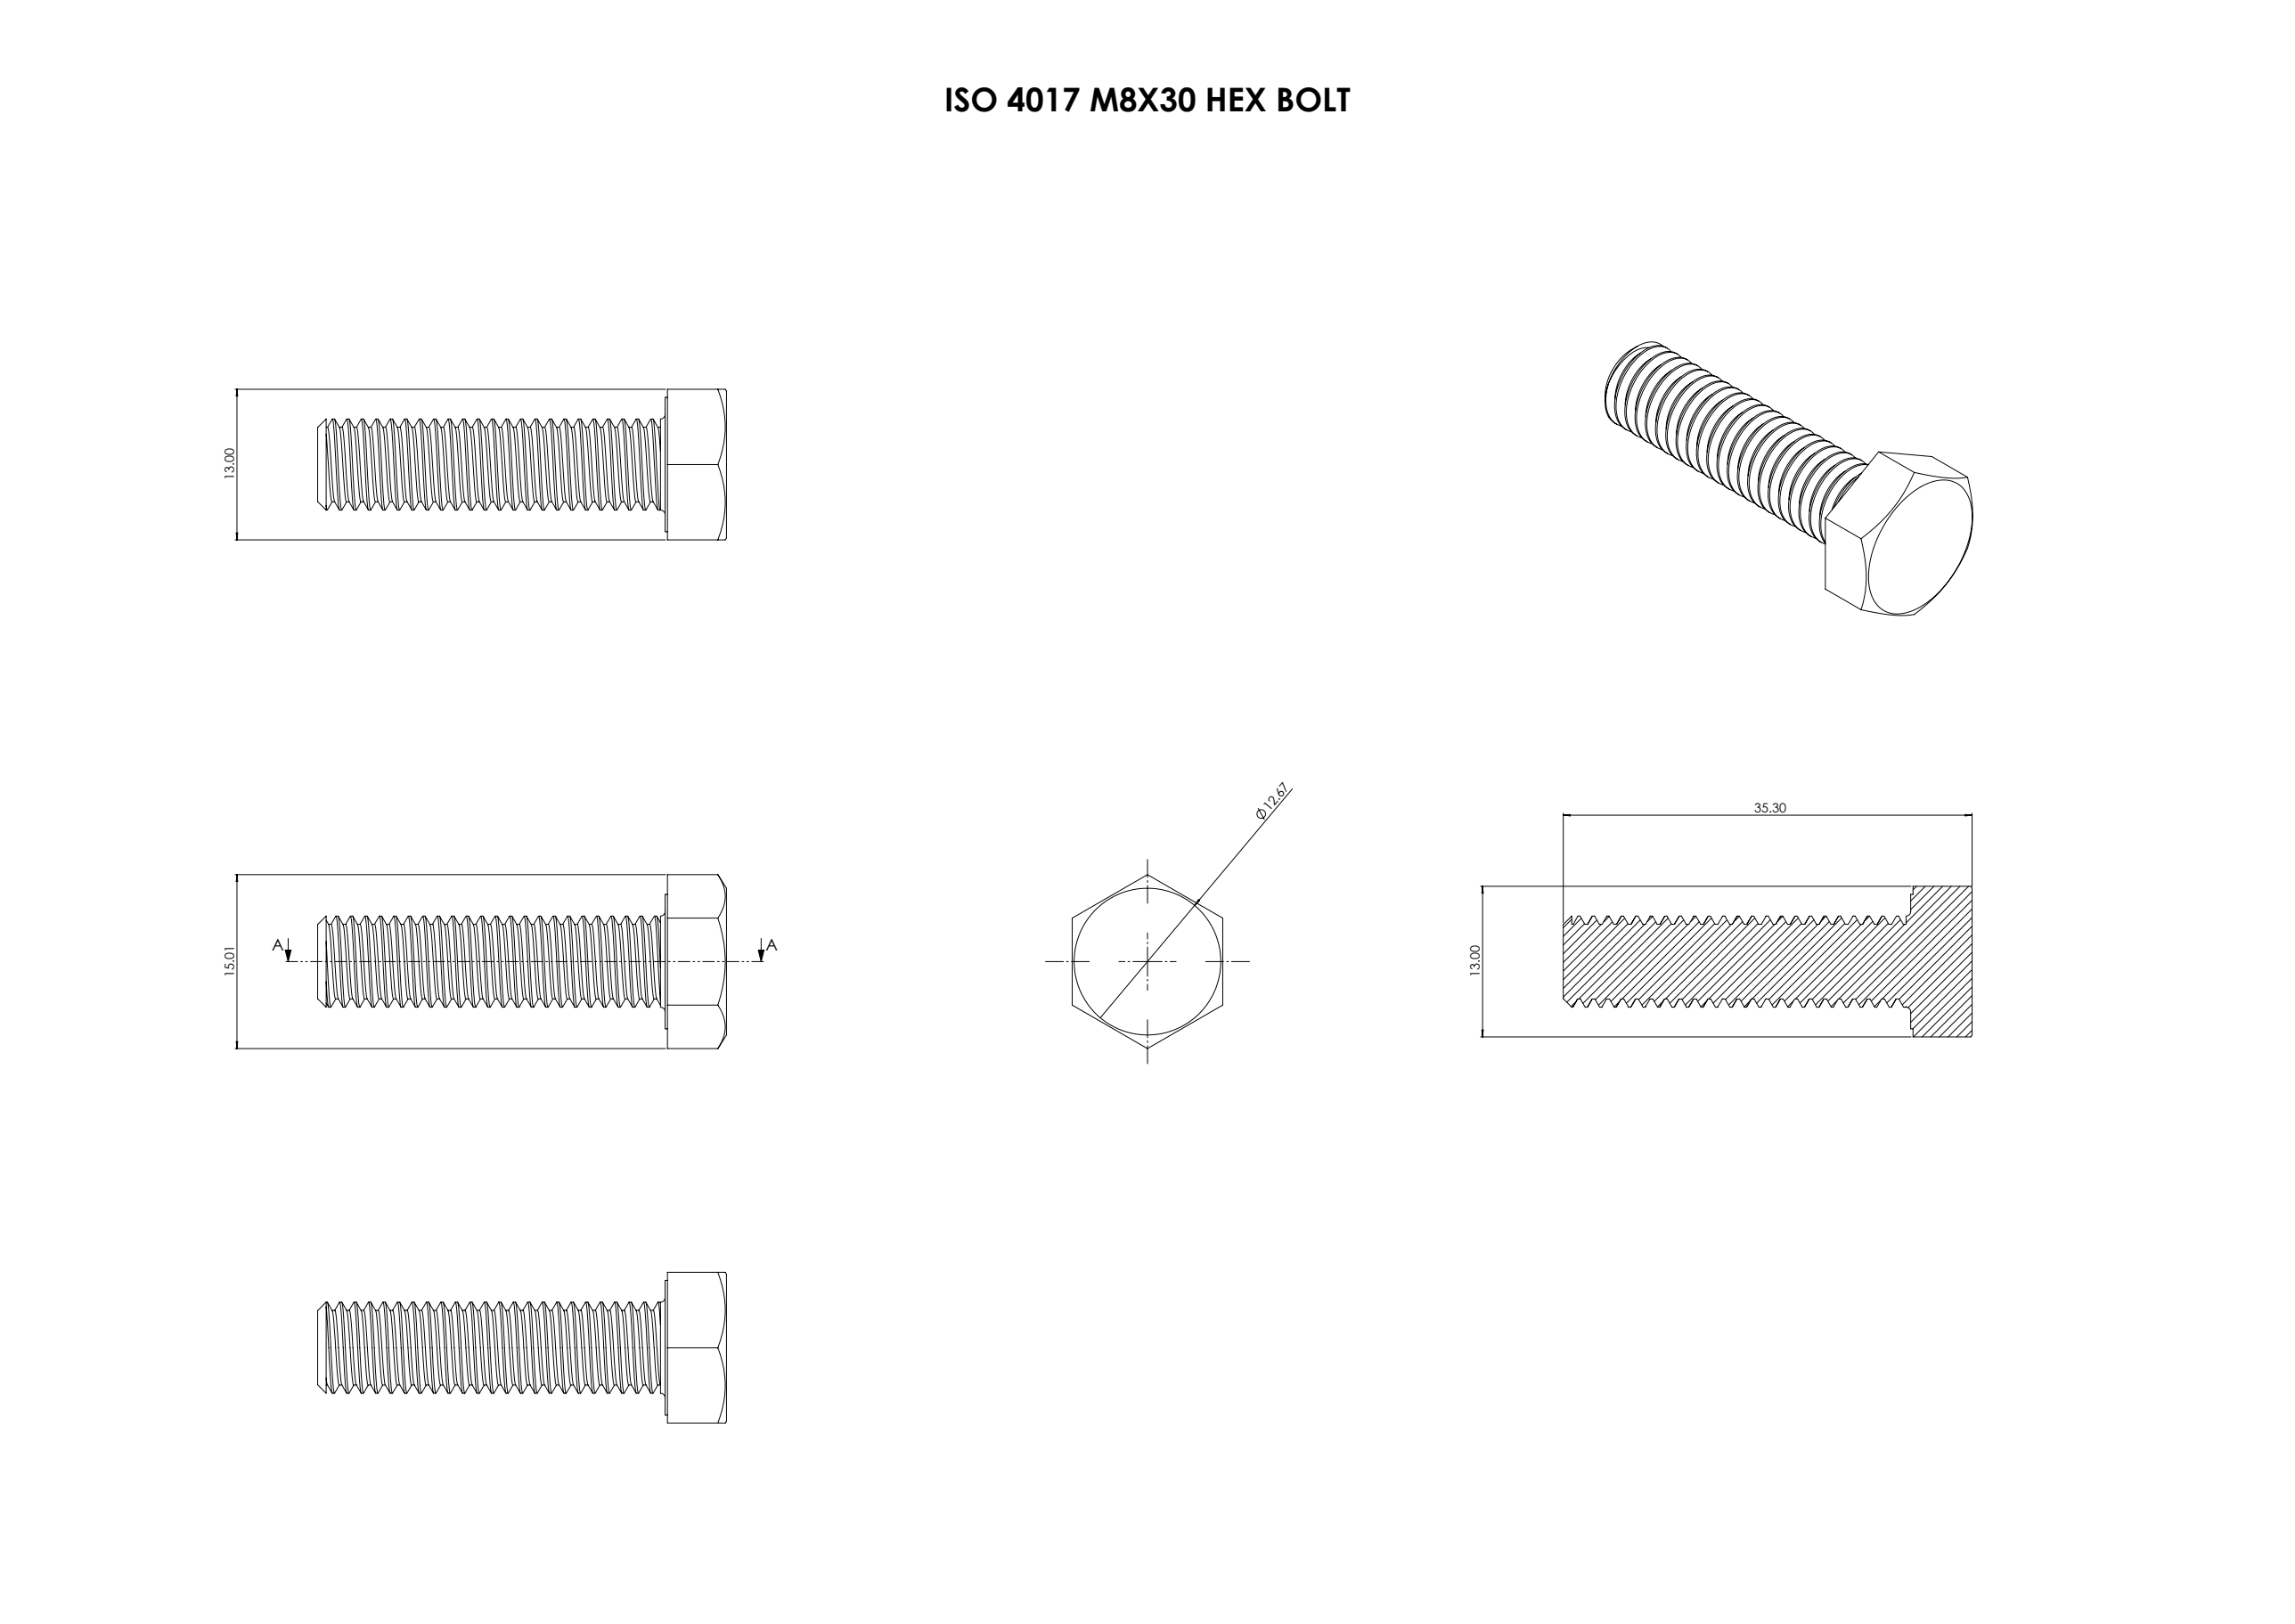
ISO-10303-21;
HEADER;
/* Generated by software containing ST-Developer
 * from STEP Tools, Inc. (www.steptools.com) 
 */

FILE_DESCRIPTION(
/* description */ (''),
/* implementation_level */ '2;1');

FILE_NAME(
/* name */ '11_ISO_4017_M8x30_Hex_Bolt.step',
/* time_stamp */ '2026-10-11T08:27:52-07:00',
/* author */ (''),
/* organization */ (''),
/* preprocessor_version */ 'ST-DEVELOPER v20.2',
/* originating_system */ 'Autodesk Translation Framework v15.15.0.0',
/* authorisation */ '');

FILE_SCHEMA (('AUTOMOTIVE_DESIGN { 1 0 10303 214 3 1 1 }'));
ENDSEC;

DATA;
#10=MECHANICAL_DESIGN_GEOMETRIC_PRESENTATION_REPRESENTATION('',(#929),#94301);
#619=B_SPLINE_CURVE_WITH_KNOTS('',3,(#90636,#90637,#90638,#90639,#90640,
#90641,#90642,#90643,#90644,#90645),.UNSPECIFIED.,.F.,.F.,(4,3,3,4),(-4.09274904019423,
-3.97736675155131,-2.98302506366348,-2.06120159751574),.UNSPECIFIED.);
#620=B_SPLINE_CURVE_WITH_KNOTS('',3,(#90648,#90649,#90650,#90651,#90652,
#90653,#90654),.UNSPECIFIED.,.F.,.F.,(4,3,4),(0.,0.994341687887822,1.11004521091126),
 .UNSPECIFIED.);
#621=B_SPLINE_CURVE_WITH_KNOTS('',3,(#90659,#90660,#90661,#90662,#90663,
#90664,#90665,#90666,#90667,#90668,#90669,#90670,#90671,#90672,#90673,#90674,
#90675,#90676,#90677,#90678,#90679,#90680),.UNSPECIFIED.,.F.,.F.,(4,3,3,
3,3,3,3,4),(-10.3759343473738,-9.94341687887826,-8.94907519099043,-7.95473350310261,
-6.96039181521478,-5.96605012732696,-4.97170843943913,-4.09274904019423),
 .UNSPECIFIED.);
#622=B_SPLINE_CURVE_WITH_KNOTS('',3,(#90681,#90682,#90683,#90684,#90685,
#90686,#90687,#90688,#90689,#90690,#90691,#90692,#90693,#90694,#90695,#90696,
#90697,#90698,#90699,#90700,#90701,#90702),.UNSPECIFIED.,.F.,.F.,(4,3,3,
3,3,3,3,4),(1.11004521091126,1.98868337577565,2.98302506366347,3.9773667515513,
4.97170843943912,5.96605012732695,6.96039181521477,7.39323051809085),
 .UNSPECIFIED.);
#623=B_SPLINE_CURVE_WITH_KNOTS('',3,(#90707,#90708,#90709,#90710,#90711,
#90712,#90713,#90714,#90715,#90716,#90717,#90718,#90719,#90720,#90721,#90722,
#90723,#90724,#90725,#90726,#90727,#90728),.UNSPECIFIED.,.F.,.F.,(4,3,3,
3,3,3,3,4),(-16.6591196545534,-15.9094670062052,-14.9151253183174,-13.9207836304296,
-12.9264419425417,-11.9321002546539,-10.9377585667661,-10.3759343473738),
 .UNSPECIFIED.);
#624=B_SPLINE_CURVE_WITH_KNOTS('',3,(#90729,#90730,#90731,#90732,#90733,
#90734,#90735,#90736,#90737,#90738,#90739,#90740,#90741,#90742,#90743,#90744,
#90745,#90746,#90747,#90748,#90749,#90750),.UNSPECIFIED.,.F.,.F.,(4,3,3,
3,3,3,3,4),(7.39323051809085,7.9547335031026,8.94907519099043,9.94341687887826,
10.9377585667661,11.9321002546539,12.9264419425418,13.6764158252704),
 .UNSPECIFIED.);
#625=B_SPLINE_CURVE_WITH_KNOTS('',3,(#90755,#90756,#90757,#90758,#90759,
#90760,#90761,#90762,#90763,#90764,#90765,#90766,#90767,#90768,#90769,#90770,
#90771,#90772,#90773,#90774,#90775,#90776,#90777,#90778,#90779),
 .UNSPECIFIED.,.F.,.F.,(4,3,3,3,3,3,3,3,4),(-22.942304961733,-22.86985882142,
-21.8755171335322,-20.8811754456444,-19.8868337577565,-18.8924920698687,
-17.8981503819809,-16.903808694093,-16.6591196545534),.UNSPECIFIED.);
#626=B_SPLINE_CURVE_WITH_KNOTS('',3,(#90780,#90781,#90782,#90783,#90784,
#90785,#90786,#90787,#90788,#90789,#90790,#90791,#90792,#90793,#90794,#90795,
#90796,#90797,#90798,#90799,#90800,#90801,#90802,#90803,#90804),
 .UNSPECIFIED.,.F.,.F.,(4,3,3,3,3,3,3,3,4),(13.6764158252704,13.9207836304296,
14.9151253183174,15.9094670062052,16.9038086940931,17.8981503819809,18.8924920698687,
19.8868337577565,19.95960113245),.UNSPECIFIED.);
#627=B_SPLINE_CURVE_WITH_KNOTS('',3,(#90809,#90810,#90811,#90812,#90813,
#90814,#90815,#90816,#90817,#90818,#90819,#90820,#90821,#90822,#90823,#90824,
#90825,#90826,#90827,#90828,#90829,#90830),.UNSPECIFIED.,.F.,.F.,(4,3,3,
3,3,3,3,4),(-29.2254902689126,-28.835908948747,-27.8415672608591,-26.8472255729713,
-25.8528838850835,-24.8585421971957,-23.8642005093078,-22.942304961733),
 .UNSPECIFIED.);
#628=B_SPLINE_CURVE_WITH_KNOTS('',3,(#90831,#90832,#90833,#90834,#90835,
#90836,#90837,#90838,#90839,#90840,#90841,#90842,#90843,#90844,#90845,#90846,
#90847,#90848,#90849,#90850,#90851,#90852),.UNSPECIFIED.,.F.,.F.,(4,3,3,
3,3,3,3,4),(19.95960113245,20.8811754456443,21.8755171335322,22.86985882142,
23.8642005093078,24.8585421971956,25.8528838850835,26.2427864396296),
 .UNSPECIFIED.);
#629=B_SPLINE_CURVE_WITH_KNOTS('',3,(#90857,#90858,#90859,#90860,#90861,
#90862,#90863,#90864,#90865,#90866,#90867,#90868,#90869,#90870,#90871,#90872,
#90873,#90874,#90875,#90876,#90877,#90878),.UNSPECIFIED.,.F.,.F.,(4,3,3,
3,3,3,3,4),(-35.5086755760922,-34.8019590760739,-33.8076173881861,-32.8132757002983,
-31.8189340124104,-30.8245923245226,-29.8302506366348,-29.2254902689126),
 .UNSPECIFIED.);
#630=B_SPLINE_CURVE_WITH_KNOTS('',3,(#90879,#90880,#90881,#90882,#90883,
#90884,#90885,#90886,#90887,#90888,#90889,#90890,#90891,#90892,#90893,#90894,
#90895,#90896,#90897,#90898,#90899,#90900),.UNSPECIFIED.,.F.,.F.,(4,3,3,
3,3,3,3,4),(26.2427864396296,26.8472255729713,27.8415672608591,28.8359089487469,
29.8302506366348,30.8245923245226,31.8189340124104,32.5259717468092),
 .UNSPECIFIED.);
#631=B_SPLINE_CURVE_WITH_KNOTS('',3,(#90905,#90906,#90907,#90908,#90909,
#90910,#90911,#90912,#90913,#90914,#90915,#90916,#90917,#90918,#90919,#90920,
#90921,#90922,#90923,#90924,#90925,#90926,#90927,#90928,#90929),
 .UNSPECIFIED.,.F.,.F.,(4,3,3,3,3,3,3,3,4),(-41.7918608832717,-41.7623508912887,
-40.7680092034009,-39.773667515513,-38.7793258276252,-37.7849841397374,
-36.7906424518496,-35.7963007639617,-35.5086755760922),.UNSPECIFIED.);
#632=B_SPLINE_CURVE_WITH_KNOTS('',3,(#90930,#90931,#90932,#90933,#90934,
#90935,#90936,#90937,#90938,#90939,#90940,#90941,#90942,#90943,#90944,#90945,
#90946,#90947,#90948,#90949,#90950,#90951,#90952,#90953,#90954),
 .UNSPECIFIED.,.F.,.F.,(4,3,3,3,3,3,3,3,4),(32.5259717468092,32.8132757002983,
33.8076173881861,34.8019590760739,35.7963007639617,36.7906424518496,37.7849841397374,
38.7793258276252,38.8091570539888),.UNSPECIFIED.);
#633=B_SPLINE_CURVE_WITH_KNOTS('',3,(#90959,#90960,#90961,#90962,#90963,
#90964,#90965,#90966,#90967,#90968,#90969,#90970,#90971,#90972,#90973,#90974,
#90975,#90976,#90977,#90978,#90979,#90980),.UNSPECIFIED.,.F.,.F.,(4,3,3,
3,3,3,3,4),(-48.0750461904514,-47.7284010186156,-46.7340593307278,-45.73971764284,
-44.7453759549522,-43.7510342670644,-42.7566925791765,-41.7918608832717),
 .UNSPECIFIED.);
#634=B_SPLINE_CURVE_WITH_KNOTS('',3,(#90981,#90982,#90983,#90984,#90985,
#90986,#90987,#90988,#90989,#90990,#90991,#90992,#90993,#90994,#90995,#90996,
#90997,#90998,#90999,#91000,#91001,#91002),.UNSPECIFIED.,.F.,.F.,(4,3,3,
3,3,3,3,4),(38.8091570539888,39.773667515513,40.7680092034009,41.7623508912887,
42.7566925791765,43.7510342670643,44.7453759549522,45.0923423611684),
 .UNSPECIFIED.);
#635=B_SPLINE_CURVE_WITH_KNOTS('',3,(#91007,#91008,#91009,#91010,#91011,
#91012,#91013,#91014,#91015,#91016,#91017,#91018,#91019,#91020,#91021,#91022,
#91023,#91024,#91025,#91026,#91027,#91028),.UNSPECIFIED.,.F.,.F.,(4,3,3,
3,3,3,3,4),(-54.3582314976309,-53.6944511459426,-52.7001094580548,-51.705767770167,
-50.7114260822791,-49.7170843943913,-48.7227427065035,-48.0750461904514),
 .UNSPECIFIED.);
#636=B_SPLINE_CURVE_WITH_KNOTS('',3,(#91029,#91030,#91031,#91032,#91033,
#91034,#91035,#91036,#91037,#91038,#91039,#91040,#91041,#91042,#91043,#91044,
#91045,#91046,#91047,#91048,#91049,#91050),.UNSPECIFIED.,.F.,.F.,(4,3,3,
3,3,3,3,4),(45.0923423611684,45.73971764284,46.7340593307278,47.7284010186156,
48.7227427065035,49.7170843943913,50.7114260822791,51.375527668348),
 .UNSPECIFIED.);
#637=B_SPLINE_CURVE_WITH_KNOTS('',3,(#91055,#91056,#91057,#91058,#91059,
#91060,#91061,#91062,#91063,#91064,#91065,#91066,#91067,#91068,#91069,#91070,
#91071,#91072,#91073,#91074,#91075,#91076),.UNSPECIFIED.,.F.,.F.,(4,3,3,
3,3,3,3,4),(-60.6414168048105,-59.6605012732696,-58.6661595853817,-57.6718178974939,
-56.6774762096061,-55.6831345217183,-54.6887928338304,-54.3582314976309),
 .UNSPECIFIED.);
#638=B_SPLINE_CURVE_WITH_KNOTS('',3,(#91077,#91078,#91079,#91080,#91081,
#91082,#91083,#91084,#91085,#91086,#91087,#91088,#91089,#91090,#91091,#91092,
#91093,#91094,#91095,#91096,#91097,#91098),.UNSPECIFIED.,.F.,.F.,(4,3,3,
3,3,3,3,4),(51.375527668348,51.705767770167,52.7001094580548,53.6944511459426,
54.6887928338304,55.6831345217183,56.6774762096061,57.6587129755276),
 .UNSPECIFIED.);
#639=B_SPLINE_CURVE_WITH_KNOTS('',3,(#91103,#91104,#91105,#91106,#91107,
#91108,#91109,#91110,#91111,#91112,#91113,#91114,#91115,#91116,#91117,#91118,
#91119,#91120,#91121,#91122,#91123,#91124,#91125,#91126,#91127),
 .UNSPECIFIED.,.F.,.F.,(4,3,3,3,3,3,3,3,4),(-66.9246021119901,-66.6208930884844,
-65.6265514005965,-64.6322097127087,-63.6378680248209,-62.643526336933,
-61.6491846490452,-60.6548429611574,-60.6414168048105),.UNSPECIFIED.);
#640=B_SPLINE_CURVE_WITH_KNOTS('',3,(#91128,#91129,#91130,#91131,#91132,
#91133,#91134,#91135,#91136,#91137,#91138,#91139,#91140,#91141,#91142,#91143,
#91144,#91145,#91146,#91147,#91148,#91149,#91150,#91151,#91152),
 .UNSPECIFIED.,.F.,.F.,(4,3,3,3,3,3,3,3,4),(57.6587129755276,57.6718178974939,
58.6661595853817,59.6605012732696,60.6548429611574,61.6491846490452,62.643526336933,
63.6378680248209,63.9418982827072),.UNSPECIFIED.);
#641=B_SPLINE_CURVE_WITH_KNOTS('',3,(#91157,#91158,#91159,#91160,#91161,
#91162,#91163,#91164,#91165,#91166,#91167,#91168,#91169,#91170,#91171,#91172,
#91173,#91174,#91175,#91176,#91177,#91178),.UNSPECIFIED.,.F.,.F.,(4,3,3,
3,3,3,3,4),(-73.2077874191697,-72.5869432158113,-71.5926015279235,-70.5982598400356,
-69.6039181521478,-68.60957646426,-67.6152347763722,-66.9246021119901),
 .UNSPECIFIED.);
#642=B_SPLINE_CURVE_WITH_KNOTS('',3,(#91179,#91180,#91181,#91182,#91183,
#91184,#91185,#91186,#91187,#91188,#91189,#91190,#91191,#91192,#91193,#91194,
#91195,#91196,#91197,#91198,#91199,#91200),.UNSPECIFIED.,.F.,.F.,(4,3,3,
3,3,3,3,4),(63.9418982827072,64.6322097127087,65.6265514005965,66.6208930884843,
67.6152347763722,68.60957646426,69.6039181521478,70.2250835898868),
 .UNSPECIFIED.);
#643=B_SPLINE_CURVE_WITH_KNOTS('',3,(#91205,#91206,#91207,#91208,#91209,
#91210,#91211,#91212,#91213,#91214,#91215,#91216,#91217,#91218,#91219,#91220,
#91221,#91222,#91223,#91224,#91225,#91226),.UNSPECIFIED.,.F.,.F.,(4,3,3,
3,3,3,3,4),(-79.4909727263493,-78.5529933431383,-77.5586516552504,-76.5643099673626,
-75.5699682794748,-74.575626591587,-73.5812849036991,-73.2077874191697),
 .UNSPECIFIED.);
#644=B_SPLINE_CURVE_WITH_KNOTS('',3,(#91227,#91228,#91229,#91230,#91231,
#91232,#91233,#91234,#91235,#91236,#91237,#91238,#91239,#91240,#91241,#91242,
#91243,#91244,#91245,#91246,#91247,#91248),.UNSPECIFIED.,.F.,.F.,(4,3,3,
3,3,3,3,4),(70.2250835898868,70.5982598400356,71.5926015279234,72.5869432158113,
73.5812849036991,74.5756265915869,75.5699682794748,76.5082688970663),
 .UNSPECIFIED.);
#645=B_SPLINE_CURVE_WITH_KNOTS('',3,(#91253,#91254,#91255,#91256,#91257,
#91258,#91259,#91260,#91261,#91262,#91263,#91264,#91265,#91266,#91267,#91268,
#91269,#91270,#91271,#91272,#91273,#91274,#91275,#91276,#91277),
 .UNSPECIFIED.,.F.,.F.,(4,3,3,3,3,3,3,3,4),(-85.7741580335289,-85.513385158353,
-84.5190434704652,-83.5247017825774,-82.5303600946896,-81.5360184068017,
-80.5416767189139,-79.5473350310261,-79.4909727263493),.UNSPECIFIED.);
#646=B_SPLINE_CURVE_WITH_KNOTS('',3,(#91278,#91279,#91280,#91281,#91282,
#91283,#91284,#91285,#91286,#91287,#91288,#91289,#91290,#91291,#91292,#91293,
#91294,#91295,#91296,#91297,#91298,#91299,#91300,#91301,#91302),
 .UNSPECIFIED.,.F.,.F.,(4,3,3,3,3,3,3,3,4),(76.5082688970663,76.5643099673626,
77.5586516552504,78.5529933431382,79.5473350310261,80.5416767189139,81.5360184068017,
82.5303600946895,82.7914542042459),.UNSPECIFIED.);
#647=B_SPLINE_CURVE_WITH_KNOTS('',3,(#91307,#91308,#91309,#91310,#91311,
#91312,#91313,#91314,#91315,#91316,#91317,#91318,#91319,#91320,#91321,#91322,
#91323,#91324,#91325,#91326,#91327,#91328),.UNSPECIFIED.,.F.,.F.,(4,3,3,
3,3,3,3,4),(-92.0573433407085,-91.47943528568,-90.4850935977922,-89.4907519099043,
-88.4964102220165,-87.5020685341287,-86.5077268462409,-85.7741580335289),
 .UNSPECIFIED.);
#648=B_SPLINE_CURVE_WITH_KNOTS('',3,(#91329,#91330,#91331,#91332,#91333,
#91334,#91335,#91336,#91337,#91338,#91339,#91340,#91341,#91342,#91343,#91344,
#91345,#91346,#91347,#91348,#91349,#91350),.UNSPECIFIED.,.F.,.F.,(4,3,3,
3,3,3,3,4),(82.7914542042459,83.5247017825774,84.5190434704652,85.513385158353,
86.5077268462408,87.5020685341287,88.4964102220165,89.0746395114255),
 .UNSPECIFIED.);
#649=B_SPLINE_CURVE_WITH_KNOTS('',3,(#91355,#91356,#91357,#91358,#91359,
#91360,#91361,#91362,#91363,#91364,#91365,#91366,#91367,#91368,#91369,#91370,
#91371,#91372,#91373,#91374,#91375,#91376),.UNSPECIFIED.,.F.,.F.,(4,3,3,
3,3,3,3,4),(-98.3405286478881,-97.4454854130069,-96.4511437251191,-95.4568020372313,
-94.4624603493435,-93.4681186614556,-92.4737769735678,-92.0573433407085),
 .UNSPECIFIED.);
#650=B_SPLINE_CURVE_WITH_KNOTS('',3,(#91377,#91378,#91379,#91380,#91381,
#91382,#91383,#91384,#91385,#91386,#91387,#91388,#91389,#91390,#91391,#91392,
#91393,#91394,#91395,#91396,#91397,#91398),.UNSPECIFIED.,.F.,.F.,(4,3,3,
3,3,3,3,4),(89.0746395114255,89.4907519099043,90.4850935977922,91.47943528568,
92.4737769735678,93.4681186614556,94.4624603493435,95.3578248186051),
 .UNSPECIFIED.);
#651=B_SPLINE_CURVE_WITH_KNOTS('',3,(#91403,#91404,#91405,#91406,#91407,
#91408,#91409,#91410,#91411,#91412,#91413,#91414,#91415,#91416,#91417,#91418,
#91419,#91420,#91421,#91422,#91423,#91424,#91425,#91426,#91427),
 .UNSPECIFIED.,.F.,.F.,(4,3,3,3,3,3,3,3,4),(-104.623713955068,-104.405877228222,
-103.411535540334,-102.417193852446,-101.422852164558,-100.42851047667,
-99.4341687887826,-98.4398271008948,-98.3405286478881),.UNSPECIFIED.);
#652=B_SPLINE_CURVE_WITH_KNOTS('',3,(#91428,#91429,#91430,#91431,#91432,
#91433,#91434,#91435,#91436,#91437,#91438,#91439,#91440,#91441,#91442,#91443,
#91444,#91445,#91446,#91447,#91448,#91449,#91450,#91451,#91452),
 .UNSPECIFIED.,.F.,.F.,(4,3,3,3,3,3,3,3,4),(95.3578248186051,95.4568020372313,
96.4511437251191,97.4454854130069,98.4398271008948,99.4341687887826,100.42851047667,
101.422852164558,101.641010125785),.UNSPECIFIED.);
#653=B_SPLINE_CURVE_WITH_KNOTS('',3,(#91457,#91458,#91459,#91460,#91461,
#91462,#91463,#91464,#91465,#91466,#91467,#91468,#91469,#91470,#91471,#91472,
#91473,#91474,#91475,#91476,#91477,#91478),.UNSPECIFIED.,.F.,.F.,(4,3,3,
3,3,3,3,4),(-110.906899262247,-110.371927355549,-109.377585667661,-108.383243979773,
-107.388902291885,-106.394560603997,-105.40021891611,-104.623713955068),
 .UNSPECIFIED.);
#654=B_SPLINE_CURVE_WITH_KNOTS('',3,(#91479,#91480,#91481,#91482,#91483,
#91484,#91485,#91486,#91487,#91488,#91489,#91490,#91491,#91492,#91493,#91494,
#91495,#91496,#91497,#91498,#91499,#91500),.UNSPECIFIED.,.F.,.F.,(4,3,3,
3,3,3,3,4),(101.641010125785,102.417193852446,103.411535540334,104.405877228222,
105.40021891611,106.394560603997,107.388902291885,107.924195432964),
 .UNSPECIFIED.);
#655=B_SPLINE_CURVE_WITH_KNOTS('',3,(#91505,#91506,#91507,#91508,#91509,
#91510,#91511,#91512,#91513,#91514,#91515,#91516,#91517,#91518,#91519,#91520,
#91521,#91522,#91523,#91524,#91525,#91526),.UNSPECIFIED.,.F.,.F.,(4,3,3,
3,3,3,3,4),(-117.190084569427,-116.337977482876,-115.343635794988,-114.3492941071,
-113.354952419212,-112.360610731324,-111.366269043437,-110.906899262247),
 .UNSPECIFIED.);
#656=B_SPLINE_CURVE_WITH_KNOTS('',3,(#91527,#91528,#91529,#91530,#91531,
#91532,#91533,#91534,#91535,#91536,#91537,#91538,#91539,#91540,#91541,#91542,
#91543,#91544,#91545,#91546,#91547,#91548),.UNSPECIFIED.,.F.,.F.,(4,3,3,
3,3,3,3,4),(107.924195432964,108.383243979773,109.377585667661,110.371927355549,
111.366269043437,112.360610731324,113.354952419212,114.207380740144),
 .UNSPECIFIED.);
#657=B_SPLINE_CURVE_WITH_KNOTS('',3,(#91553,#91554,#91555,#91556,#91557,
#91558,#91559,#91560,#91561,#91562,#91563,#91564,#91565,#91566,#91567,#91568,
#91569,#91570,#91571,#91572,#91573,#91574,#91575,#91576,#91577),
 .UNSPECIFIED.,.F.,.F.,(4,3,3,3,3,3,3,3,4),(-123.473269876606,-123.29836929809,
-122.304027610203,-121.309685922315,-120.315344234427,-119.321002546539,
-118.326660858651,-117.332319170763,-117.190084569427),.UNSPECIFIED.);
#658=B_SPLINE_CURVE_WITH_KNOTS('',3,(#91578,#91579,#91580,#91581,#91582,
#91583,#91584,#91585,#91586,#91587,#91588,#91589,#91590,#91591,#91592,#91593,
#91594,#91595,#91596,#91597,#91598,#91599,#91600,#91601,#91602),
 .UNSPECIFIED.,.F.,.F.,(4,3,3,3,3,3,3,3,4),(114.207380740144,114.3492941071,
115.343635794988,116.337977482876,117.332319170763,118.326660858651,119.321002546539,
120.315344234427,120.490566047323),.UNSPECIFIED.);
#659=B_SPLINE_CURVE_WITH_KNOTS('',3,(#91607,#91608,#91609,#91610,#91611,
#91612,#91613,#91614,#91615,#91616,#91617,#91618,#91619,#91620,#91621,#91622,
#91623,#91624,#91625,#91626,#91627,#91628),.UNSPECIFIED.,.F.,.F.,(4,3,3,
3,3,3,3,4),(-129.756455183786,-129.264419425417,-128.27007773753,-127.275736049642,
-126.281394361754,-125.287052673866,-124.292710985978,-123.473269876606),
 .UNSPECIFIED.);
#660=B_SPLINE_CURVE_WITH_KNOTS('',3,(#91629,#91630,#91631,#91632,#91633,
#91634,#91635,#91636,#91637,#91638,#91639,#91640,#91641,#91642,#91643,#91644,
#91645,#91646,#91647,#91648,#91649,#91650),.UNSPECIFIED.,.F.,.F.,(4,3,3,
3,3,3,3,4),(120.490566047323,121.309685922315,122.304027610203,123.29836929809,
124.292710985978,125.287052673866,126.281394361754,126.773751354503),
 .UNSPECIFIED.);
#661=B_SPLINE_CURVE_WITH_KNOTS('',3,(#91655,#91656,#91657,#91658,#91659,
#91660,#91661,#91662,#91663,#91664,#91665,#91666,#91667,#91668,#91669,#91670,
#91671,#91672,#91673,#91674,#91675,#91676),.UNSPECIFIED.,.F.,.F.,(4,3,3,
3,3,3,3,4),(-136.039640490966,-135.230469552744,-134.236127864856,-133.241786176969,
-132.247444489081,-131.253102801193,-130.258761113305,-129.756455183786),
 .UNSPECIFIED.);
#662=B_SPLINE_CURVE_WITH_KNOTS('',3,(#91677,#91678,#91679,#91680,#91681,
#91682,#91683,#91684,#91685,#91686,#91687,#91688,#91689,#91690,#91691,#91692,
#91693,#91694,#91695,#91696,#91697,#91698),.UNSPECIFIED.,.F.,.F.,(4,3,3,
3,3,3,3,4),(126.773751354503,127.275736049642,128.27007773753,129.264419425417,
130.258761113305,131.253102801193,132.247444489081,133.056936661683),
 .UNSPECIFIED.);
#663=B_SPLINE_CURVE_WITH_KNOTS('',3,(#91703,#91704,#91705,#91706,#91707,
#91708,#91709,#91710,#91711,#91712,#91713,#91714,#91715,#91716,#91717,#91718,
#91719,#91720,#91721,#91722,#91723,#91724,#91725,#91726,#91727),
 .UNSPECIFIED.,.F.,.F.,(4,3,3,3,3,3,3,3,4),(-142.322825798145,-142.190861367959,
-141.196519680071,-140.202177992183,-139.207836304296,-138.213494616408,
-137.21915292852,-136.224811240632,-136.039640490966),.UNSPECIFIED.);
#664=B_SPLINE_CURVE_WITH_KNOTS('',3,(#91728,#91729,#91730,#91731,#91732,
#91733,#91734,#91735,#91736,#91737,#91738,#91739,#91740,#91741,#91742,#91743,
#91744,#91745,#91746,#91747,#91748,#91749,#91750,#91751,#91752),
 .UNSPECIFIED.,.F.,.F.,(4,3,3,3,3,3,3,3,4),(133.056936661683,133.241786176969,
134.236127864857,135.230469552744,136.224811240632,137.21915292852,138.213494616408,
139.207836304296,139.340121968862),.UNSPECIFIED.);
#665=B_SPLINE_CURVE_WITH_KNOTS('',3,(#91758,#91759,#91760,#91761,#91762,
#91763),.UNSPECIFIED.,.F.,.F.,(4,1,1,4),(153.9380400259,154.800417283602,
155.79475897149,156.716582437637),.UNSPECIFIED.);
#666=B_SPLINE_CURVE_WITH_KNOTS('',3,(#91766,#91767,#91768,#91769,#91770),
 .UNSPECIFIED.,.F.,.F.,(4,1,4),(153.9380400259,154.482960869368,155.477302557256),
 .UNSPECIFIED.);
#667=B_SPLINE_CURVE_WITH_KNOTS('',3,(#91775,#91776,#91777,#91778,#91779,
#91780,#91781,#91782,#91783,#91784,#91785),.UNSPECIFIED.,.F.,.F.,(4,1,1,
1,1,1,1,1,4),(147.65485471872,147.840025468387,148.834367156275,149.828708844163,
150.82305053205,151.817392219938,152.811733907826,153.806075595714,153.9380400259),
 .UNSPECIFIED.);
#668=B_SPLINE_CURVE_WITH_KNOTS('',3,(#91786,#91787,#91788,#91789,#91790,
#91791,#91792,#91793,#91794,#91795),.UNSPECIFIED.,.F.,.F.,(4,1,1,1,1,1,
1,4),(147.65485471872,148.516910742041,149.511252429929,150.505594117817,
151.499935805705,152.494277493593,153.488619181481,153.9380400259),
 .UNSPECIFIED.);
#669=B_SPLINE_CURVE_WITH_KNOTS('',3,(#91800,#91801,#91802,#91803,#91804,
#91805,#91806,#91807,#91808,#91809),.UNSPECIFIED.,.F.,.F.,(4,1,1,1,1,1,
1,4),(141.371669411541,141.87397534106,142.868317028948,143.862658716836,
144.857000404723,145.851342092611,146.845683780499,147.65485471872),
 .UNSPECIFIED.);
#670=B_SPLINE_CURVE_WITH_KNOTS('',3,(#91810,#91811,#91812,#91813,#91814,
#91815,#91816,#91817,#91818,#91819,#91820),.UNSPECIFIED.,.F.,.F.,(4,1,1,
1,1,1,1,1,4),(141.371669411541,141.556518926827,142.550860614715,143.545202302602,
144.53954399049,145.533885678378,146.528227366266,147.522569054154,147.65485471872),
 .UNSPECIFIED.);
#671=B_SPLINE_CURVE_WITH_KNOTS('',3,(#91825,#91826,#91827,#91828,#91829,
#91830,#91831,#91832,#91833,#91834),.UNSPECIFIED.,.F.,.F.,(4,1,1,1,1,1,
1,4),(135.088484104361,135.907925213733,136.902266901621,137.896608589509,
138.890950277396,139.885291965284,140.879633653172,141.371669411541),
 .UNSPECIFIED.);
#672=B_SPLINE_CURVE_WITH_KNOTS('',3,(#91835,#91836,#91837,#91838,#91839,
#91840,#91841,#91842,#91843,#91844),.UNSPECIFIED.,.F.,.F.,(4,1,1,1,1,1,
1,4),(135.088484104361,135.5904687995,136.584810487388,137.579152175275,
138.573493863163,139.567835551051,140.562177238939,141.371669411541),
 .UNSPECIFIED.);
#673=B_SPLINE_CURVE_WITH_KNOTS('',3,(#91849,#91850,#91851,#91852,#91853,
#91854,#91855,#91856,#91857,#91858,#91859),.UNSPECIFIED.,.F.,.F.,(4,1,1,
1,1,1,1,1,4),(128.805298797182,128.947533398518,129.941875086406,130.936216774294,
131.930558462182,132.92490015007,133.919241837957,134.913583525845,135.088484104361),
 .UNSPECIFIED.);
#674=B_SPLINE_CURVE_WITH_KNOTS('',3,(#91860,#91861,#91862,#91863,#91864,
#91865,#91866,#91867,#91868,#91869),.UNSPECIFIED.,.F.,.F.,(4,1,1,1,1,1,
1,4),(128.805298797182,129.624418672173,130.618760360061,131.613102047948,
132.607443735836,133.601785423724,134.596127111612,135.088484104361),
 .UNSPECIFIED.);
#675=B_SPLINE_CURVE_WITH_KNOTS('',3,(#91874,#91875,#91876,#91877,#91878,
#91879,#91880,#91881,#91882,#91883),.UNSPECIFIED.,.F.,.F.,(4,1,1,1,1,1,
1,4),(122.522113490002,122.981483271191,123.975824959079,124.970166646967,
125.964508334855,126.958850022743,127.95319171063,128.805298797182),
 .UNSPECIFIED.);
#676=B_SPLINE_CURVE_WITH_KNOTS('',3,(#91884,#91885,#91886,#91887,#91888,
#91889,#91890,#91891,#91892,#91893,#91894),.UNSPECIFIED.,.F.,.F.,(4,1,1,
1,1,1,1,1,4),(122.522113490002,122.664026856958,123.658368544846,124.652710232734,
125.647051920622,126.641393608509,127.635735296397,128.630076984285,128.805298797182),
 .UNSPECIFIED.);
#677=B_SPLINE_CURVE_WITH_KNOTS('',3,(#91899,#91900,#91901,#91902,#91903,
#91904,#91905,#91906,#91907,#91908),.UNSPECIFIED.,.F.,.F.,(4,1,1,1,1,1,
1,4),(116.238928182822,117.015433143864,118.009774831752,119.00411651964,
119.998458207528,120.992799895416,121.987141583303,122.522113490002),
 .UNSPECIFIED.);
#678=B_SPLINE_CURVE_WITH_KNOTS('',3,(#91909,#91910,#91911,#91912,#91913,
#91914,#91915,#91916,#91917,#91918),.UNSPECIFIED.,.F.,.F.,(4,1,1,1,1,1,
1,4),(116.238928182822,116.697976729631,117.692318417519,118.686660105407,
119.681001793295,120.675343481182,121.66968516907,122.522113490002),
 .UNSPECIFIED.);
#679=B_SPLINE_CURVE_WITH_KNOTS('',3,(#91923,#91924,#91925,#91926,#91927,
#91928,#91929,#91930,#91931,#91932,#91933),.UNSPECIFIED.,.F.,.F.,(4,1,1,
1,1,1,1,1,4),(109.955742875643,110.05504132865,111.049383016537,112.043724704425,
113.038066392313,114.032408080201,115.026749768089,116.021091455976,116.238928182822),
 .UNSPECIFIED.);
#680=B_SPLINE_CURVE_WITH_KNOTS('',3,(#91934,#91935,#91936,#91937,#91938,
#91939,#91940,#91941,#91942,#91943),.UNSPECIFIED.,.F.,.F.,(4,1,1,1,1,1,
1,4),(109.955742875643,110.731926602304,111.726268290192,112.72060997808,
113.714951665968,114.709293353855,115.703635041743,116.238928182822),
 .UNSPECIFIED.);
#681=B_SPLINE_CURVE_WITH_KNOTS('',3,(#91948,#91949,#91950,#91951,#91952,
#91953,#91954,#91955,#91956,#91957),.UNSPECIFIED.,.F.,.F.,(4,1,1,1,1,1,
1,4),(103.672557568463,104.088991201323,105.08333288921,106.077674577098,
107.072016264986,108.066357952874,109.060699640762,109.955742875643),
 .UNSPECIFIED.);
#682=B_SPLINE_CURVE_WITH_KNOTS('',3,(#91958,#91959,#91960,#91961,#91962,
#91963,#91964,#91965,#91966,#91967,#91968),.UNSPECIFIED.,.F.,.F.,(4,1,1,
1,1,1,1,1,4),(103.672557568463,103.771534787089,104.765876474977,105.760218162865,
106.754559850753,107.748901538641,108.743243226528,109.737584914416,109.955742875643),
 .UNSPECIFIED.);
#683=B_SPLINE_CURVE_WITH_KNOTS('',3,(#91973,#91974,#91975,#91976,#91977,
#91978,#91979,#91980,#91981,#91982),.UNSPECIFIED.,.F.,.F.,(4,1,1,1,1,1,
1,4),(97.3893722612836,98.1229410739956,99.1172827618834,100.111624449771,
101.105966137659,102.100307825547,103.094649513435,103.672557568463),
 .UNSPECIFIED.);
#684=B_SPLINE_CURVE_WITH_KNOTS('',3,(#91983,#91984,#91985,#91986,#91987,
#91988,#91989,#91990,#91991,#91992),.UNSPECIFIED.,.F.,.F.,(4,1,1,1,1,1,
1,4),(97.3893722612836,97.8054846597624,98.7998263476502,99.794168035538,
100.788509723426,101.782851411314,102.777193099202,103.672557568463),
 .UNSPECIFIED.);
#685=B_SPLINE_CURVE_WITH_KNOTS('',3,(#91997,#91998,#91999,#92000,#92001,
#92002,#92003,#92004,#92005,#92006,#92007),.UNSPECIFIED.,.F.,.F.,(4,1,1,
1,1,1,1,1,4),(91.106186954104,91.1625492587808,92.1568909466686,93.1512326345565,
94.1455743224443,95.1399160103321,96.13425769822,97.1285993861078,97.3893722612836),
 .UNSPECIFIED.);
#686=B_SPLINE_CURVE_WITH_KNOTS('',3,(#92008,#92009,#92010,#92011,#92012,
#92013,#92014,#92015,#92016,#92017),.UNSPECIFIED.,.F.,.F.,(4,1,1,1,1,1,
1,4),(91.106186954104,91.8394345324354,92.8337762203232,93.8281179082111,
94.8224595960989,95.8168012839867,96.8111429718745,97.3893722612836),
 .UNSPECIFIED.);
#687=B_SPLINE_CURVE_WITH_KNOTS('',3,(#92022,#92023,#92024,#92025,#92026,
#92027,#92028,#92029,#92030,#92031),.UNSPECIFIED.,.F.,.F.,(4,1,1,1,1,1,
1,4),(84.8230016469244,85.1964991314539,86.1908408193417,87.1851825072295,
88.1795241951173,89.1738658830052,90.168207570893,91.106186954104),
 .UNSPECIFIED.);
#688=B_SPLINE_CURVE_WITH_KNOTS('',3,(#92032,#92033,#92034,#92035,#92036,
#92037,#92038,#92039,#92040,#92041,#92042),.UNSPECIFIED.,.F.,.F.,(4,1,1,
1,1,1,1,1,4),(84.8230016469244,84.8790427172206,85.8733844051085,86.8677260929963,
87.8620677808841,88.8564094687719,89.8507511566598,90.8450928445476,91.106186954104),
 .UNSPECIFIED.);
#689=B_SPLINE_CURVE_WITH_KNOTS('',3,(#92047,#92048,#92049,#92050,#92051,
#92052,#92053,#92054,#92055,#92056),.UNSPECIFIED.,.F.,.F.,(4,1,1,1,1,1,
1,4),(78.5398163397448,79.2304490041269,80.2247906920147,81.2191323799026,
82.2134740677904,83.2078157556782,84.202157443566,84.8230016469244),
 .UNSPECIFIED.);
#690=B_SPLINE_CURVE_WITH_KNOTS('',3,(#92057,#92058,#92059,#92060,#92061,
#92062,#92063,#92064,#92065,#92066),.UNSPECIFIED.,.F.,.F.,(4,1,1,1,1,1,
1,4),(78.5398163397448,78.9129925898937,79.9073342777815,80.9016759656693,
81.8960176535572,82.890359341445,83.8847010293328,84.8230016469244),
 .UNSPECIFIED.);
#691=B_SPLINE_CURVE_WITH_KNOTS('',3,(#92071,#92072,#92073,#92074,#92075,
#92076,#92077,#92078,#92079,#92080,#92081),.UNSPECIFIED.,.F.,.F.,(4,1,1,
1,1,1,1,1,4),(72.2566310325653,72.2700571889121,73.2643988768,74.2587405646878,
75.2530822525756,76.2474239404634,77.2417656283513,78.2361073162391,78.5398163397448),
 .UNSPECIFIED.);
#692=B_SPLINE_CURVE_WITH_KNOTS('',3,(#92082,#92083,#92084,#92085,#92086,
#92087,#92088,#92089,#92090,#92091),.UNSPECIFIED.,.F.,.F.,(4,1,1,1,1,1,
1,4),(72.2566310325653,72.9469424625667,73.9412841504546,74.9356258383424,
75.9299675262302,76.924309214118,77.9186509020059,78.5398163397448),
 .UNSPECIFIED.);
#693=B_SPLINE_CURVE_WITH_KNOTS('',3,(#92096,#92097,#92098,#92099,#92100,
#92101,#92102,#92103,#92104,#92105),.UNSPECIFIED.,.F.,.F.,(4,1,1,1,1,1,
1,4),(65.9734457253856,66.3040070615852,67.298348749473,68.2926904373608,
69.2870321252486,70.2813738131365,71.2757155010243,72.2566310325653),
 .UNSPECIFIED.);
#694=B_SPLINE_CURVE_WITH_KNOTS('',3,(#92106,#92107,#92108,#92109,#92110,
#92111,#92112,#92113,#92114,#92115,#92116),.UNSPECIFIED.,.F.,.F.,(4,1,1,
1,1,1,1,1,4),(65.9734457253856,65.9865506473519,66.9808923352398,67.9752340231276,
68.9695757110154,69.9639173989032,70.9582590867911,71.9526007746789,72.2566310325653),
 .UNSPECIFIED.);
#695=B_SPLINE_CURVE_WITH_KNOTS('',3,(#92121,#92122,#92123,#92124,#92125,
#92126,#92127,#92128,#92129,#92130),.UNSPECIFIED.,.F.,.F.,(4,1,1,1,1,1,
1,4),(59.6902604182061,60.3379569342582,61.332298622146,62.3266403100339,
63.3209819979217,64.3153236858095,65.3096653736973,65.9734457253856),
 .UNSPECIFIED.);
#696=B_SPLINE_CURVE_WITH_KNOTS('',3,(#92131,#92132,#92133,#92134,#92135,
#92136,#92137,#92138,#92139,#92140),.UNSPECIFIED.,.F.,.F.,(4,1,1,1,1,1,
1,4),(59.6902604182061,60.020500520025,61.0148422079128,62.0091838958006,
63.0035255836885,63.9978672715763,64.9922089594641,65.9734457253856),
 .UNSPECIFIED.);
#697=B_SPLINE_CURVE_WITH_KNOTS('',3,(#92145,#92146,#92147,#92148,#92149,
#92150,#92151,#92152,#92153,#92154),.UNSPECIFIED.,.F.,.F.,(4,1,1,1,1,1,
1,4),(53.4070751110265,54.3719068069313,55.3662484948191,56.3605901827069,
57.3549318705947,58.3492735584826,59.3436152463704,59.6902604182061),
 .UNSPECIFIED.);
#698=B_SPLINE_CURVE_WITH_KNOTS('',3,(#92155,#92156,#92157,#92158,#92159,
#92160,#92161,#92162,#92163,#92164),.UNSPECIFIED.,.F.,.F.,(4,1,1,1,1,1,
1,4),(53.4070751110265,54.054450392698,55.0487920805859,56.0431337684737,
57.0374754563615,58.0318171442493,59.0261588321372,59.6902604182061),
 .UNSPECIFIED.);
#699=B_SPLINE_CURVE_WITH_KNOTS('',3,(#92169,#92170,#92171,#92172,#92173,
#92174,#92175,#92176,#92177,#92178,#92179),.UNSPECIFIED.,.F.,.F.,(4,1,1,
1,1,1,1,1,4),(47.1238898038469,47.4115149917165,48.4058566796043,49.4001983674921,
50.3945400553799,51.3888817432678,52.3832234311556,53.3775651190434,53.4070751110265),
 .UNSPECIFIED.);
#700=B_SPLINE_CURVE_WITH_KNOTS('',3,(#92180,#92181,#92182,#92183,#92184,
#92185,#92186,#92187,#92188,#92189),.UNSPECIFIED.,.F.,.F.,(4,1,1,1,1,1,
1,4),(47.1238898038469,48.0884002653711,49.0827419532589,50.0770836411467,
51.0714253290346,52.0657670169224,53.0601087048102,53.4070751110265),
 .UNSPECIFIED.);
#701=B_SPLINE_CURVE_WITH_KNOTS('',3,(#92194,#92195,#92196,#92197,#92198,
#92199,#92200,#92201,#92202,#92203),.UNSPECIFIED.,.F.,.F.,(4,1,1,1,1,1,
1,4),(40.8407044966673,41.4454648643895,42.4398065522773,43.4341482401652,
44.428489928053,45.4228316159408,46.4171733038286,47.1238898038469),
 .UNSPECIFIED.);
#702=B_SPLINE_CURVE_WITH_KNOTS('',3,(#92204,#92205,#92206,#92207,#92208,
#92209,#92210,#92211,#92212,#92213,#92214),.UNSPECIFIED.,.F.,.F.,(4,1,1,
1,1,1,1,1,4),(40.8407044966673,41.1280084501563,42.1223501380441,43.116691825932,
44.1110335138198,45.1053752017076,46.0997168895954,47.0940585774833,47.1238898038469),
 .UNSPECIFIED.);
#703=B_SPLINE_CURVE_WITH_KNOTS('',3,(#92219,#92220,#92221,#92222,#92223,
#92224,#92225,#92226,#92227,#92228),.UNSPECIFIED.,.F.,.F.,(4,1,1,1,1,1,
1,4),(34.5575191894877,35.4794147370626,36.4737564249504,37.4680981128382,
38.462439800726,39.4567814886139,40.4511231765017,40.8407044966673),
 .UNSPECIFIED.);
#704=B_SPLINE_CURVE_WITH_KNOTS('',3,(#92229,#92230,#92231,#92232,#92233,
#92234,#92235,#92236,#92237,#92238),.UNSPECIFIED.,.F.,.F.,(4,1,1,1,1,1,
1,4),(34.5575191894877,35.1619583228293,36.1563000107172,37.150641698605,
38.1449833864928,39.1393250743807,40.1336667622685,40.8407044966673),
 .UNSPECIFIED.);
#705=B_SPLINE_CURVE_WITH_KNOTS('',3,(#92243,#92244,#92245,#92246,#92247,
#92248,#92249,#92250,#92251,#92252,#92253),.UNSPECIFIED.,.F.,.F.,(4,1,1,
1,1,1,1,1,4),(28.2743338823081,28.5190229218478,29.5133646097356,30.5077062976234,
31.5020479855113,32.4963896733991,33.4907313612869,34.4850730491747,34.5575191894877),
 .UNSPECIFIED.);
#706=B_SPLINE_CURVE_WITH_KNOTS('',3,(#92254,#92255,#92256,#92257,#92258,
#92259,#92260,#92261,#92262,#92263),.UNSPECIFIED.,.F.,.F.,(4,1,1,1,1,1,
1,4),(28.2743338823081,29.1959081955024,30.1902498833902,31.184591571278,
32.1789332591659,33.1732749470537,34.1676166349415,34.5575191894877),
 .UNSPECIFIED.);
#707=B_SPLINE_CURVE_WITH_KNOTS('',3,(#92268,#92269,#92270,#92271,#92272,
#92273,#92274,#92275,#92276,#92277),.UNSPECIFIED.,.F.,.F.,(4,1,1,1,1,1,
1,4),(21.9911485751285,22.5529727945208,23.5473144824086,24.5416561702965,
25.5359978581843,26.5303395460721,27.52468123396,28.2743338823081),
 .UNSPECIFIED.);
#708=B_SPLINE_CURVE_WITH_KNOTS('',3,(#92278,#92279,#92280,#92281,#92282,
#92283,#92284,#92285,#92286,#92287,#92288),.UNSPECIFIED.,.F.,.F.,(4,1,1,
1,1,1,1,1,4),(21.9911485751285,22.2355163802876,23.2298580681754,24.2241997560633,
25.2185414439511,26.2128831318389,27.2072248197267,28.2015665076146,28.2743338823081),
 .UNSPECIFIED.);
#709=B_SPLINE_CURVE_WITH_KNOTS('',3,(#92293,#92294,#92295,#92296,#92297,
#92298,#92299,#92300,#92301,#92302),.UNSPECIFIED.,.F.,.F.,(4,1,1,1,1,1,
1,4),(15.7079632679489,16.5869226671939,17.5812643550817,18.5756060429695,
19.5699477308573,20.5642894187452,21.558631106633,21.9911485751285),
 .UNSPECIFIED.);
#710=B_SPLINE_CURVE_WITH_KNOTS('',3,(#92303,#92304,#92305,#92306,#92307,
#92308,#92309,#92310,#92311,#92312),.UNSPECIFIED.,.F.,.F.,(4,1,1,1,1,1,
1,4),(15.7079632679489,16.2694662529607,17.2638079408485,18.2581496287363,
19.2524913166241,20.246833004512,21.2411746923998,21.9911485751285),
 .UNSPECIFIED.);
#711=B_SPLINE_CURVE_WITH_KNOTS('',3,(#92315,#92316,#92317,#92318,#92319,
#92320,#92321,#92322,#92323,#92324,#92325,#92326,#92327,#92328,#92329,#92330,
#92331,#92332,#92333,#92334,#92335,#92336,#92337,#92338,#92339,#92340,#92341,
#92342,#92343,#92344,#92345,#92346,#92347,#92348,#92349,#92350,#92351,#92352,
#92353,#92354,#92355,#92356,#92357,#92358,#92359,#92360,#92361,#92362,#92363,
#92364,#92365,#92366,#92367,#92368,#92369,#92370,#92371,#92372,#92373,#92374,
#92375,#92376,#92377,#92378,#92379,#92380,#92381,#92382,#92383,#92384,#92385,
#92386,#92387,#92388,#92389,#92390,#92391,#92392,#92393,#92394,#92395,#92396,
#92397,#92398,#92399,#92400,#92401,#92402,#92403,#92404,#92405,#92406,#92407,
#92408,#92409,#92410,#92411),.UNSPECIFIED.,.F.,.F.,(4,3,3,3,3,3,3,3,3,3,
3,3,3,3,3,3,3,3,3,3,3,3,3,3,3,3,3,3,3,3,3,3,4),(-0.744397949170625,-0.720695733926605,
-0.689559276510196,-0.670036103351393,-0.659844114683856,-0.653655602764569,
-0.621646994773415,-0.591089683672906,-0.577510322236719,-0.571672000985749,
-0.566558200256387,-0.533181563358221,-0.499287246195234,-0.465487035108622,
-0.443412402823803,-0.436945256166294,-0.431748865628828,-0.396836613409468,
-0.377188505969346,-0.343448059020756,-0.309075827600796,-0.297163948119586,
-0.292811939195563,-0.258415064258314,-0.222910728343378,-0.187071424676623,
-0.163687496592045,-0.150656708009009,-0.145666602593747,-0.108928864805471,
-0.0721282795251585,-0.0360213506839708,0.),.UNSPECIFIED.);
#712=B_SPLINE_CURVE_WITH_KNOTS('',3,(#92416,#92417,#92418,#92419,#92420,
#92421,#92422,#92423,#92424,#92425,#92426,#92427,#92428,#92429,#92430,#92431,
#92432,#92433,#92434,#92435,#92436,#92437,#92438,#92439,#92440,#92441,#92442,
#92443,#92444,#92445,#92446,#92447,#92448,#92449,#92450,#92451,#92452,#92453,
#92454,#92455,#92456,#92457,#92458,#92459,#92460,#92461,#92462,#92463,#92464,
#92465,#92466,#92467,#92468,#92469,#92470,#92471,#92472,#92473,#92474,#92475,
#92476,#92477,#92478,#92479,#92480,#92481,#92482,#92483,#92484,#92485,#92486,
#92487,#92488,#92489,#92490,#92491,#92492,#92493,#92494,#92495,#92496,#92497,
#92498,#92499,#92500,#92501,#92502,#92503,#92504,#92505,#92506,#92507,#92508,
#92509,#92510,#92511,#92512),.UNSPECIFIED.,.F.,.F.,(4,3,3,3,3,3,3,3,3,3,
3,3,3,3,3,3,3,3,3,3,3,3,3,3,3,3,3,3,3,3,3,3,4),(-0.741270768406274,-0.712807950605837,
-0.676238641188094,-0.655219890693859,-0.642041516507432,-0.635990628203364,
-0.598984128837985,-0.566603441893278,-0.552436891354969,-0.544103215434064,
-0.537640090039063,-0.502240448549675,-0.467092661838385,-0.432981215367342,
-0.409720569845589,-0.402357089590634,-0.397540473388326,-0.363890224767345,
-0.339938633280332,-0.305661805073138,-0.27125659544551,-0.263740502835797,
-0.257191774771573,-0.223767368565723,-0.190306650667009,-0.157253142518131,
-0.137596499703365,-0.128270421992769,-0.123230695487105,-0.0910288793094783,
-0.0592786340288667,-0.0285032472800834,0.),.UNSPECIFIED.);
#713=B_SPLINE_CURVE_WITH_KNOTS('',3,(#93117,#93118,#93119,#93120,#93121,
#93122,#93123,#93124,#93125,#93126,#93127,#93128,#93129,#93130,#93131,#93132,
#93133,#93134,#93135),.UNSPECIFIED.,.F.,.F.,(4,3,3,3,3,3,4),(139.340121968862,
140.202177992183,141.196519680071,142.190861367959,143.185203055847,144.179544743735,
145.101368209882),.UNSPECIFIED.);
#714=B_SPLINE_CURVE_WITH_KNOTS('',3,(#93137,#93138,#93139,#93140,#93141,
#93142,#93143,#93144,#93145,#93146,#93147,#93148,#93149,#93150,#93151,#93152,
#93153,#93154,#93155,#93156,#93157,#93158,#93159,#93160,#93161,#93162,#93163,
#93164,#93165,#93166,#93167,#93168,#93169,#93170,#93171,#93172,#93173,#93174,
#93175,#93176,#93177,#93178,#93179,#93180,#93181,#93182,#93183,#93184,#93185,
#93186,#93187,#93188,#93189,#93190,#93191,#93192,#93193,#93194,#93195,#93196,
#93197,#93198,#93199,#93200,#93201,#93202,#93203,#93204,#93205,#93206,#93207,
#93208,#93209,#93210,#93211,#93212,#93213,#93214,#93215,#93216,#93217,#93218,
#93219,#93220,#93221,#93222,#93223,#93224,#93225,#93226,#93227,#93228,#93229,
#93230,#93231,#93232,#93233),.UNSPECIFIED.,.F.,.F.,(4,3,3,3,3,3,3,3,3,3,
3,3,3,3,3,3,3,3,3,3,3,3,3,3,3,3,3,3,3,3,3,3,4),(-0.744397949170602,-0.720695733926586,
-0.6895592934692,-0.670036119250459,-0.659844170884589,-0.653655608554017,
-0.621647015639673,-0.591089701930882,-0.577510352001926,-0.571671825159275,
-0.566558171753553,-0.533181542619665,-0.499287226983445,-0.465487016280342,
-0.443412388702592,-0.436945445960127,-0.431748880838135,-0.39683662780105,
-0.377188505969343,-0.343448066421773,-0.309075843625405,-0.297163975261819,
-0.292811966402081,-0.258415099070131,-0.222910772035957,-0.187071472120164,
-0.163687538105144,-0.150656788140358,-0.145666622445593,-0.108928889508498,
-0.072128300796967,-0.0360213509544539,0.),.UNSPECIFIED.);
#715=B_SPLINE_CURVE_WITH_KNOTS('',3,(#93234,#93235,#93236,#93237,#93238,
#93239,#93240,#93241,#93242),.UNSPECIFIED.,.F.,.F.,(4,1,1,1,1,1,4),(10.3759343473738,
11.2977578135215,12.2920995014094,13.2864411892972,14.280782877185,15.2751245650728,
15.7079632679489),.UNSPECIFIED.);
#716=B_SPLINE_CURVE_WITH_KNOTS('',3,(#93248,#93249,#93250,#93251,#93252,
#93253,#93254,#93255,#93256,#93257,#93258,#93259,#93260,#93261,#93262,#93263,
#93264,#93265,#93266,#93267,#93268,#93269,#93270,#93271,#93272,#93273,#93274,
#93275,#93276,#93277,#93278,#93279,#93280,#93281,#93282,#93283,#93284,#93285,
#93286,#93287,#93288,#93289,#93290,#93291,#93292,#93293,#93294,#93295,#93296,
#93297,#93298,#93299,#93300,#93301,#93302,#93303,#93304,#93305,#93306,#93307,
#93308,#93309,#93310,#93311,#93312,#93313,#93314,#93315,#93316,#93317,#93318,
#93319,#93320,#93321,#93322,#93323,#93324,#93325,#93326,#93327,#93328,#93329,
#93330,#93331,#93332,#93333,#93334,#93335,#93336,#93337,#93338,#93339,#93340,
#93341,#93342,#93343,#93344),.UNSPECIFIED.,.F.,.F.,(4,3,3,3,3,3,3,3,3,3,
3,3,3,3,3,3,3,3,3,3,3,3,3,3,3,3,3,3,3,3,3,3,4),(-0.741270768406348,-0.712807950605888,
-0.676238640305255,-0.655219889866198,-0.642041511505912,-0.635990623215072,
-0.598984124473231,-0.566603438074119,-0.552436887774508,-0.544103204743418,
-0.537640086026196,-0.50224044348667,-0.467092649849235,-0.432981184709489,
-0.409720546852202,-0.402357044665001,-0.397540380185969,-0.36389011877745,
-0.33993863328034,-0.305661795379487,-0.271256588274296,-0.263740488713404,
-0.2571917764368,-0.223767364341805,-0.190306652230719,-0.15725316132804,
-0.137596516162035,-0.128270487710825,-0.123230703086563,-0.091028901639038,
-0.0592786783268478,-0.0285033201413548,0.),.UNSPECIFIED.);
#717=B_SPLINE_CURVE_WITH_KNOTS('',3,(#93347,#93348,#93349,#93350,#93351,
#93352,#93353,#93354),.UNSPECIFIED.,.F.,.F.,(4,1,1,1,1,4),(11.6152142277547,
12.6095559156426,13.6038976035304,14.5982392914182,15.592580979306,15.7079632679489),
 .UNSPECIFIED.);
#718=B_SPLINE_CURVE_WITH_KNOTS('',3,(#93959,#93960,#93961,#93962,#93963,
#93964,#93965,#93966,#93967,#93968,#93969,#93970,#93971,#93972,#93973,#93974),
 .UNSPECIFIED.,.F.,.F.,(4,3,3,3,3,4),(-147.162569807398,-146.16822811951,
-145.173886431623,-144.179544743735,-143.185203055847,-142.322825798145),
 .UNSPECIFIED.);
#889=B_SPLINE_SURFACE_WITH_KNOTS('',3,3,((#92513,#92514,#92515,#92516,#92517,
#92518,#92519,#92520,#92521,#92522,#92523,#92524,#92525,#92526,#92527,#92528,
#92529,#92530,#92531,#92532,#92533,#92534,#92535,#92536,#92537,#92538,#92539,
#92540,#92541,#92542,#92543,#92544,#92545,#92546,#92547,#92548,#92549,#92550,
#92551,#92552,#92553,#92554,#92555,#92556,#92557,#92558,#92559,#92560,#92561,
#92562,#92563,#92564,#92565,#92566,#92567,#92568,#92569,#92570,#92571,#92572,
#92573,#92574,#92575,#92576,#92577,#92578,#92579,#92580,#92581,#92582,#92583,
#92584,#92585,#92586,#92587,#92588,#92589,#92590,#92591,#92592,#92593,#92594,
#92595,#92596,#92597,#92598,#92599,#92600,#92601,#92602,#92603,#92604,#92605,
#92606,#92607,#92608,#92609,#92610,#92611,#92612,#92613,#92614,#92615,#92616,
#92617,#92618,#92619,#92620,#92621,#92622,#92623,#92624,#92625,#92626,#92627,
#92628,#92629,#92630,#92631,#92632,#92633,#92634,#92635,#92636,#92637,#92638,
#92639,#92640,#92641,#92642,#92643,#92644,#92645,#92646,#92647,#92648,#92649,
#92650,#92651,#92652,#92653,#92654,#92655,#92656,#92657,#92658,#92659,#92660,
#92661,#92662,#92663),(#92664,#92665,#92666,#92667,#92668,#92669,#92670,
#92671,#92672,#92673,#92674,#92675,#92676,#92677,#92678,#92679,#92680,#92681,
#92682,#92683,#92684,#92685,#92686,#92687,#92688,#92689,#92690,#92691,#92692,
#92693,#92694,#92695,#92696,#92697,#92698,#92699,#92700,#92701,#92702,#92703,
#92704,#92705,#92706,#92707,#92708,#92709,#92710,#92711,#92712,#92713,#92714,
#92715,#92716,#92717,#92718,#92719,#92720,#92721,#92722,#92723,#92724,#92725,
#92726,#92727,#92728,#92729,#92730,#92731,#92732,#92733,#92734,#92735,#92736,
#92737,#92738,#92739,#92740,#92741,#92742,#92743,#92744,#92745,#92746,#92747,
#92748,#92749,#92750,#92751,#92752,#92753,#92754,#92755,#92756,#92757,#92758,
#92759,#92760,#92761,#92762,#92763,#92764,#92765,#92766,#92767,#92768,#92769,
#92770,#92771,#92772,#92773,#92774,#92775,#92776,#92777,#92778,#92779,#92780,
#92781,#92782,#92783,#92784,#92785,#92786,#92787,#92788,#92789,#92790,#92791,
#92792,#92793,#92794,#92795,#92796,#92797,#92798,#92799,#92800,#92801,#92802,
#92803,#92804,#92805,#92806,#92807,#92808,#92809,#92810,#92811,#92812,#92813,
#92814),(#92815,#92816,#92817,#92818,#92819,#92820,#92821,#92822,#92823,
#92824,#92825,#92826,#92827,#92828,#92829,#92830,#92831,#92832,#92833,#92834,
#92835,#92836,#92837,#92838,#92839,#92840,#92841,#92842,#92843,#92844,#92845,
#92846,#92847,#92848,#92849,#92850,#92851,#92852,#92853,#92854,#92855,#92856,
#92857,#92858,#92859,#92860,#92861,#92862,#92863,#92864,#92865,#92866,#92867,
#92868,#92869,#92870,#92871,#92872,#92873,#92874,#92875,#92876,#92877,#92878,
#92879,#92880,#92881,#92882,#92883,#92884,#92885,#92886,#92887,#92888,#92889,
#92890,#92891,#92892,#92893,#92894,#92895,#92896,#92897,#92898,#92899,#92900,
#92901,#92902,#92903,#92904,#92905,#92906,#92907,#92908,#92909,#92910,#92911,
#92912,#92913,#92914,#92915,#92916,#92917,#92918,#92919,#92920,#92921,#92922,
#92923,#92924,#92925,#92926,#92927,#92928,#92929,#92930,#92931,#92932,#92933,
#92934,#92935,#92936,#92937,#92938,#92939,#92940,#92941,#92942,#92943,#92944,
#92945,#92946,#92947,#92948,#92949,#92950,#92951,#92952,#92953,#92954,#92955,
#92956,#92957,#92958,#92959,#92960,#92961,#92962,#92963,#92964,#92965),
(#92966,#92967,#92968,#92969,#92970,#92971,#92972,#92973,#92974,#92975,
#92976,#92977,#92978,#92979,#92980,#92981,#92982,#92983,#92984,#92985,#92986,
#92987,#92988,#92989,#92990,#92991,#92992,#92993,#92994,#92995,#92996,#92997,
#92998,#92999,#93000,#93001,#93002,#93003,#93004,#93005,#93006,#93007,#93008,
#93009,#93010,#93011,#93012,#93013,#93014,#93015,#93016,#93017,#93018,#93019,
#93020,#93021,#93022,#93023,#93024,#93025,#93026,#93027,#93028,#93029,#93030,
#93031,#93032,#93033,#93034,#93035,#93036,#93037,#93038,#93039,#93040,#93041,
#93042,#93043,#93044,#93045,#93046,#93047,#93048,#93049,#93050,#93051,#93052,
#93053,#93054,#93055,#93056,#93057,#93058,#93059,#93060,#93061,#93062,#93063,
#93064,#93065,#93066,#93067,#93068,#93069,#93070,#93071,#93072,#93073,#93074,
#93075,#93076,#93077,#93078,#93079,#93080,#93081,#93082,#93083,#93084,#93085,
#93086,#93087,#93088,#93089,#93090,#93091,#93092,#93093,#93094,#93095,#93096,
#93097,#93098,#93099,#93100,#93101,#93102,#93103,#93104,#93105,#93106,#93107,
#93108,#93109,#93110,#93111,#93112,#93113,#93114,#93115,#93116)),
 .UNSPECIFIED.,.F.,.F.,.F.,(4,4),(4,1,1,1,1,1,1,1,1,1,1,1,1,1,1,1,1,1,1,
1,1,1,1,1,1,1,1,1,1,1,1,1,1,1,1,1,1,1,1,1,1,1,1,1,1,1,1,1,1,1,1,1,1,1,1,
1,1,1,1,1,1,1,1,1,1,1,1,1,1,1,1,1,1,1,1,1,1,1,1,1,1,1,1,1,1,1,1,1,1,1,1,
1,1,1,1,1,1,1,1,1,1,1,1,1,1,1,1,1,1,1,1,1,1,1,1,1,1,1,1,1,1,1,1,1,1,1,1,
1,1,1,1,1,1,1,1,1,1,1,1,1,1,1,1,1,1,1,1,1,4),(0.,0.0820126057383863),(8.31473274985805,
9.30907443774587,10.3034161256337,11.2977578135215,12.2920995014094,13.2864411892972,
14.280782877185,15.2751245650728,16.2694662529607,17.2638079408485,18.2581496287363,
19.2524913166241,20.246833004512,21.2411746923998,22.2355163802876,23.2298580681754,
24.2241997560633,25.2185414439511,26.2128831318389,27.2072248197267,28.2015665076146,
29.1959081955024,30.1902498833902,31.184591571278,32.1789332591659,33.1732749470537,
34.1676166349415,35.1619583228293,36.1563000107172,37.150641698605,38.1449833864928,
39.1393250743807,40.1336667622685,41.1280084501563,42.1223501380441,43.116691825932,
44.1110335138198,45.1053752017076,46.0997168895954,47.0940585774833,48.0884002653711,
49.0827419532589,50.0770836411467,51.0714253290346,52.0657670169224,53.0601087048102,
54.054450392698,55.0487920805859,56.0431337684737,57.0374754563615,58.0318171442493,
59.0261588321372,60.020500520025,61.0148422079128,62.0091838958006,63.0035255836885,
63.9978672715763,64.9922089594641,65.9865506473519,66.9808923352398,67.9752340231276,
68.9695757110154,69.9639173989032,70.9582590867911,71.9526007746789,72.9469424625667,
73.9412841504546,74.9356258383424,75.9299675262302,76.924309214118,77.9186509020059,
78.9129925898937,79.9073342777815,80.9016759656693,81.8960176535572,82.890359341445,
83.8847010293328,84.8790427172206,85.8733844051085,86.8677260929963,87.8620677808841,
88.8564094687719,89.8507511566598,90.8450928445476,91.8394345324354,92.8337762203232,
93.8281179082111,94.8224595960989,95.8168012839867,96.8111429718745,97.8054846597624,
98.7998263476502,99.794168035538,100.788509723426,101.782851411314,102.777193099202,
103.771534787089,104.765876474977,105.760218162865,106.754559850753,107.748901538641,
108.743243226528,109.737584914416,110.731926602304,111.726268290192,112.72060997808,
113.714951665968,114.709293353855,115.703635041743,116.697976729631,117.692318417519,
118.686660105407,119.681001793295,120.675343481182,121.66968516907,122.664026856958,
123.658368544846,124.652710232734,125.647051920622,126.641393608509,127.635735296397,
128.630076984285,129.624418672173,130.618760360061,131.613102047948,132.607443735836,
133.601785423724,134.596127111612,135.5904687995,136.584810487388,137.579152175275,
138.573493863163,139.567835551051,140.562177238939,141.556518926827,142.550860614715,
143.545202302602,144.53954399049,145.533885678378,146.528227366266,147.522569054154,
148.516910742041,149.511252429929,150.505594117817,151.499935805705,152.494277493593,
153.488619181481,154.482960869368,155.477302557256),.UNSPECIFIED.);
#890=B_SPLINE_SURFACE_WITH_KNOTS('',3,3,((#93355,#93356,#93357,#93358,#93359,
#93360,#93361,#93362,#93363,#93364,#93365,#93366,#93367,#93368,#93369,#93370,
#93371,#93372,#93373,#93374,#93375,#93376,#93377,#93378,#93379,#93380,#93381,
#93382,#93383,#93384,#93385,#93386,#93387,#93388,#93389,#93390,#93391,#93392,
#93393,#93394,#93395,#93396,#93397,#93398,#93399,#93400,#93401,#93402,#93403,
#93404,#93405,#93406,#93407,#93408,#93409,#93410,#93411,#93412,#93413,#93414,
#93415,#93416,#93417,#93418,#93419,#93420,#93421,#93422,#93423,#93424,#93425,
#93426,#93427,#93428,#93429,#93430,#93431,#93432,#93433,#93434,#93435,#93436,
#93437,#93438,#93439,#93440,#93441,#93442,#93443,#93444,#93445,#93446,#93447,
#93448,#93449,#93450,#93451,#93452,#93453,#93454,#93455,#93456,#93457,#93458,
#93459,#93460,#93461,#93462,#93463,#93464,#93465,#93466,#93467,#93468,#93469,
#93470,#93471,#93472,#93473,#93474,#93475,#93476,#93477,#93478,#93479,#93480,
#93481,#93482,#93483,#93484,#93485,#93486,#93487,#93488,#93489,#93490,#93491,
#93492,#93493,#93494,#93495,#93496,#93497,#93498,#93499,#93500,#93501,#93502,
#93503,#93504,#93505),(#93506,#93507,#93508,#93509,#93510,#93511,#93512,
#93513,#93514,#93515,#93516,#93517,#93518,#93519,#93520,#93521,#93522,#93523,
#93524,#93525,#93526,#93527,#93528,#93529,#93530,#93531,#93532,#93533,#93534,
#93535,#93536,#93537,#93538,#93539,#93540,#93541,#93542,#93543,#93544,#93545,
#93546,#93547,#93548,#93549,#93550,#93551,#93552,#93553,#93554,#93555,#93556,
#93557,#93558,#93559,#93560,#93561,#93562,#93563,#93564,#93565,#93566,#93567,
#93568,#93569,#93570,#93571,#93572,#93573,#93574,#93575,#93576,#93577,#93578,
#93579,#93580,#93581,#93582,#93583,#93584,#93585,#93586,#93587,#93588,#93589,
#93590,#93591,#93592,#93593,#93594,#93595,#93596,#93597,#93598,#93599,#93600,
#93601,#93602,#93603,#93604,#93605,#93606,#93607,#93608,#93609,#93610,#93611,
#93612,#93613,#93614,#93615,#93616,#93617,#93618,#93619,#93620,#93621,#93622,
#93623,#93624,#93625,#93626,#93627,#93628,#93629,#93630,#93631,#93632,#93633,
#93634,#93635,#93636,#93637,#93638,#93639,#93640,#93641,#93642,#93643,#93644,
#93645,#93646,#93647,#93648,#93649,#93650,#93651,#93652,#93653,#93654,#93655,
#93656),(#93657,#93658,#93659,#93660,#93661,#93662,#93663,#93664,#93665,
#93666,#93667,#93668,#93669,#93670,#93671,#93672,#93673,#93674,#93675,#93676,
#93677,#93678,#93679,#93680,#93681,#93682,#93683,#93684,#93685,#93686,#93687,
#93688,#93689,#93690,#93691,#93692,#93693,#93694,#93695,#93696,#93697,#93698,
#93699,#93700,#93701,#93702,#93703,#93704,#93705,#93706,#93707,#93708,#93709,
#93710,#93711,#93712,#93713,#93714,#93715,#93716,#93717,#93718,#93719,#93720,
#93721,#93722,#93723,#93724,#93725,#93726,#93727,#93728,#93729,#93730,#93731,
#93732,#93733,#93734,#93735,#93736,#93737,#93738,#93739,#93740,#93741,#93742,
#93743,#93744,#93745,#93746,#93747,#93748,#93749,#93750,#93751,#93752,#93753,
#93754,#93755,#93756,#93757,#93758,#93759,#93760,#93761,#93762,#93763,#93764,
#93765,#93766,#93767,#93768,#93769,#93770,#93771,#93772,#93773,#93774,#93775,
#93776,#93777,#93778,#93779,#93780,#93781,#93782,#93783,#93784,#93785,#93786,
#93787,#93788,#93789,#93790,#93791,#93792,#93793,#93794,#93795,#93796,#93797,
#93798,#93799,#93800,#93801,#93802,#93803,#93804,#93805,#93806,#93807),
(#93808,#93809,#93810,#93811,#93812,#93813,#93814,#93815,#93816,#93817,
#93818,#93819,#93820,#93821,#93822,#93823,#93824,#93825,#93826,#93827,#93828,
#93829,#93830,#93831,#93832,#93833,#93834,#93835,#93836,#93837,#93838,#93839,
#93840,#93841,#93842,#93843,#93844,#93845,#93846,#93847,#93848,#93849,#93850,
#93851,#93852,#93853,#93854,#93855,#93856,#93857,#93858,#93859,#93860,#93861,
#93862,#93863,#93864,#93865,#93866,#93867,#93868,#93869,#93870,#93871,#93872,
#93873,#93874,#93875,#93876,#93877,#93878,#93879,#93880,#93881,#93882,#93883,
#93884,#93885,#93886,#93887,#93888,#93889,#93890,#93891,#93892,#93893,#93894,
#93895,#93896,#93897,#93898,#93899,#93900,#93901,#93902,#93903,#93904,#93905,
#93906,#93907,#93908,#93909,#93910,#93911,#93912,#93913,#93914,#93915,#93916,
#93917,#93918,#93919,#93920,#93921,#93922,#93923,#93924,#93925,#93926,#93927,
#93928,#93929,#93930,#93931,#93932,#93933,#93934,#93935,#93936,#93937,#93938,
#93939,#93940,#93941,#93942,#93943,#93944,#93945,#93946,#93947,#93948,#93949,
#93950,#93951,#93952,#93953,#93954,#93955,#93956,#93957,#93958)),
 .UNSPECIFIED.,.F.,.F.,.F.,(4,4),(4,1,1,1,1,1,1,1,1,1,1,1,1,1,1,1,1,1,1,
1,1,1,1,1,1,1,1,1,1,1,1,1,1,1,1,1,1,1,1,1,1,1,1,1,1,1,1,1,1,1,1,1,1,1,1,
1,1,1,1,1,1,1,1,1,1,1,1,1,1,1,1,1,1,1,1,1,1,1,1,1,1,1,1,1,1,1,1,1,1,1,1,
1,1,1,1,1,1,1,1,1,1,1,1,1,1,1,1,1,1,1,1,1,1,1,1,1,1,1,1,1,1,1,1,1,1,1,1,
1,1,1,1,1,1,1,1,1,1,1,1,1,1,1,1,1,1,1,1,1,4),(0.,0.0820126057383863),(11.6152142277547,
12.6095559156426,13.6038976035304,14.5982392914182,15.592580979306,16.5869226671939,
17.5812643550817,18.5756060429695,19.5699477308573,20.5642894187452,21.558631106633,
22.5529727945208,23.5473144824086,24.5416561702965,25.5359978581843,26.5303395460721,
27.52468123396,28.5190229218478,29.5133646097356,30.5077062976234,31.5020479855113,
32.4963896733991,33.4907313612869,34.4850730491747,35.4794147370626,36.4737564249504,
37.4680981128382,38.462439800726,39.4567814886139,40.4511231765017,41.4454648643895,
42.4398065522773,43.4341482401652,44.428489928053,45.4228316159408,46.4171733038286,
47.4115149917165,48.4058566796043,49.4001983674921,50.3945400553799,51.3888817432678,
52.3832234311556,53.3775651190434,54.3719068069313,55.3662484948191,56.3605901827069,
57.3549318705947,58.3492735584826,59.3436152463704,60.3379569342582,61.332298622146,
62.3266403100339,63.3209819979217,64.3153236858095,65.3096653736973,66.3040070615852,
67.298348749473,68.2926904373608,69.2870321252486,70.2813738131365,71.2757155010243,
72.2700571889121,73.2643988768,74.2587405646878,75.2530822525756,76.2474239404634,
77.2417656283513,78.2361073162391,79.2304490041269,80.2247906920147,81.2191323799026,
82.2134740677904,83.2078157556782,84.202157443566,85.1964991314539,86.1908408193417,
87.1851825072295,88.1795241951173,89.1738658830052,90.168207570893,91.1625492587808,
92.1568909466686,93.1512326345565,94.1455743224443,95.1399160103321,96.13425769822,
97.1285993861078,98.1229410739956,99.1172827618834,100.111624449771,101.105966137659,
102.100307825547,103.094649513435,104.088991201323,105.08333288921,106.077674577098,
107.072016264986,108.066357952874,109.060699640762,110.05504132865,111.049383016537,
112.043724704425,113.038066392313,114.032408080201,115.026749768089,116.021091455976,
117.015433143864,118.009774831752,119.00411651964,119.998458207528,120.992799895416,
121.987141583303,122.981483271191,123.975824959079,124.970166646967,125.964508334855,
126.958850022743,127.95319171063,128.947533398518,129.941875086406,130.936216774294,
131.930558462182,132.92490015007,133.919241837957,134.913583525845,135.907925213733,
136.902266901621,137.896608589509,138.890950277396,139.885291965284,140.879633653172,
141.87397534106,142.868317028948,143.862658716836,144.857000404723,145.851342092611,
146.845683780499,147.840025468387,148.834367156275,149.828708844163,150.82305053205,
151.817392219938,152.811733907826,153.806075595714,154.800417283602,155.79475897149,
156.789100659377,157.783442347265,158.777784035153),.UNSPECIFIED.);
#901=SHAPE_REPRESENTATION_RELATIONSHIP('SRR','None',#94381,#915);
#915=ADVANCED_BREP_SHAPE_REPRESENTATION('',(#943),#94297);
#929=STYLED_ITEM('',(#94588),#943);
#943=MANIFOLD_SOLID_BREP('Body1',#51028);
#958=TOROIDAL_SURFACE('',#55249,4.333,0.4);
#1038=FACE_BOUND('',#18648,.T.);
#1039=FACE_BOUND('',#18661,.T.);
#1233=CYLINDRICAL_SURFACE('',#55193,3.933);
#1234=CYLINDRICAL_SURFACE('',#55195,3.933);
#1235=CYLINDRICAL_SURFACE('',#55196,3.933);
#1236=CYLINDRICAL_SURFACE('',#55197,3.933);
#1237=CYLINDRICAL_SURFACE('',#55198,3.933);
#1238=CYLINDRICAL_SURFACE('',#55199,3.933);
#1239=CYLINDRICAL_SURFACE('',#55200,3.933);
#1240=CYLINDRICAL_SURFACE('',#55201,3.933);
#1241=CYLINDRICAL_SURFACE('',#55202,3.933);
#1242=CYLINDRICAL_SURFACE('',#55203,3.933);
#1243=CYLINDRICAL_SURFACE('',#55204,3.933);
#1244=CYLINDRICAL_SURFACE('',#55205,3.933);
#1245=CYLINDRICAL_SURFACE('',#55206,3.933);
#1246=CYLINDRICAL_SURFACE('',#55207,3.933);
#1247=CYLINDRICAL_SURFACE('',#55208,3.933);
#1248=CYLINDRICAL_SURFACE('',#55209,3.933);
#1249=CYLINDRICAL_SURFACE('',#55210,3.933);
#1250=CYLINDRICAL_SURFACE('',#55211,3.933);
#1251=CYLINDRICAL_SURFACE('',#55212,3.933);
#1252=CYLINDRICAL_SURFACE('',#55213,3.933);
#1253=CYLINDRICAL_SURFACE('',#55214,3.933);
#1254=CYLINDRICAL_SURFACE('',#55215,3.933);
#1255=CYLINDRICAL_SURFACE('',#55216,3.933);
#1256=CYLINDRICAL_SURFACE('',#55217,3.22275);
#1257=CYLINDRICAL_SURFACE('',#55219,3.22275);
#1258=CYLINDRICAL_SURFACE('',#55220,3.22275);
#1259=CYLINDRICAL_SURFACE('',#55221,3.22275);
#1260=CYLINDRICAL_SURFACE('',#55222,3.22275);
#1261=CYLINDRICAL_SURFACE('',#55223,3.22275);
#1262=CYLINDRICAL_SURFACE('',#55224,3.22275);
#1263=CYLINDRICAL_SURFACE('',#55225,3.22275);
#1264=CYLINDRICAL_SURFACE('',#55226,3.22275);
#1265=CYLINDRICAL_SURFACE('',#55227,3.22275);
#1266=CYLINDRICAL_SURFACE('',#55228,3.22275);
#1267=CYLINDRICAL_SURFACE('',#55229,3.22275);
#1268=CYLINDRICAL_SURFACE('',#55230,3.22275);
#1269=CYLINDRICAL_SURFACE('',#55231,3.22275);
#1270=CYLINDRICAL_SURFACE('',#55232,3.22275);
#1271=CYLINDRICAL_SURFACE('',#55233,3.22275);
#1272=CYLINDRICAL_SURFACE('',#55234,3.22275);
#1273=CYLINDRICAL_SURFACE('',#55235,3.22275);
#1274=CYLINDRICAL_SURFACE('',#55236,3.22275);
#1275=CYLINDRICAL_SURFACE('',#55237,3.22275);
#1276=CYLINDRICAL_SURFACE('',#55238,3.22275);
#1277=CYLINDRICAL_SURFACE('',#55239,3.22275);
#1278=CYLINDRICAL_SURFACE('',#55240,3.22275);
#1279=CYLINDRICAL_SURFACE('',#55248,3.22275);
#1280=CYLINDRICAL_SURFACE('',#55253,3.933);
#1281=CYLINDRICAL_SURFACE('',#55261,5.8);
#6605=LINE('',#90634,#11133);
#6606=LINE('',#90658,#11134);
#6607=LINE('',#90706,#11135);
#6608=LINE('',#90754,#11136);
#6609=LINE('',#90808,#11137);
#6610=LINE('',#90856,#11138);
#6611=LINE('',#90904,#11139);
#6612=LINE('',#90958,#11140);
#6613=LINE('',#91006,#11141);
#6614=LINE('',#91054,#11142);
#6615=LINE('',#91102,#11143);
#6616=LINE('',#91156,#11144);
#6617=LINE('',#91204,#11145);
#6618=LINE('',#91252,#11146);
#6619=LINE('',#91306,#11147);
#6620=LINE('',#91354,#11148);
#6621=LINE('',#91402,#11149);
#6622=LINE('',#91456,#11150);
#6623=LINE('',#91504,#11151);
#6624=LINE('',#91552,#11152);
#6625=LINE('',#91606,#11153);
#6626=LINE('',#91654,#11154);
#6627=LINE('',#91702,#11155);
#6628=LINE('',#91756,#11156);
#6629=LINE('',#91774,#11157);
#6630=LINE('',#91799,#11158);
#6631=LINE('',#91824,#11159);
#6632=LINE('',#91848,#11160);
#6633=LINE('',#91873,#11161);
#6634=LINE('',#91898,#11162);
#6635=LINE('',#91922,#11163);
#6636=LINE('',#91947,#11164);
#6637=LINE('',#91972,#11165);
#6638=LINE('',#91996,#11166);
#6639=LINE('',#92021,#11167);
#6640=LINE('',#92046,#11168);
#6641=LINE('',#92070,#11169);
#6642=LINE('',#92095,#11170);
#6643=LINE('',#92120,#11171);
#6644=LINE('',#92144,#11172);
#6645=LINE('',#92168,#11173);
#6646=LINE('',#92193,#11174);
#6647=LINE('',#92218,#11175);
#6648=LINE('',#92242,#11176);
#6649=LINE('',#92267,#11177);
#6650=LINE('',#92292,#11178);
#6651=LINE('',#94007,#11179);
#6652=LINE('',#94014,#11180);
#6653=LINE('',#94016,#11181);
#6654=LINE('',#94017,#11182);
#6655=LINE('',#94020,#11183);
#6656=LINE('',#94021,#11184);
#6657=LINE('',#94024,#11185);
#6658=LINE('',#94025,#11186);
#6659=LINE('',#94029,#11187);
#6660=LINE('',#94034,#11188);
#6661=LINE('',#94037,#11189);
#6662=LINE('',#94038,#11190);
#6663=LINE('',#94041,#11191);
#6664=LINE('',#94042,#11192);
#6665=LINE('',#94044,#11193);
#11133=VECTOR('',#67827,4.);
#11134=VECTOR('',#67832,4.);
#11135=VECTOR('',#67835,4.);
#11136=VECTOR('',#67838,4.);
#11137=VECTOR('',#67841,4.);
#11138=VECTOR('',#67844,4.);
#11139=VECTOR('',#67847,4.);
#11140=VECTOR('',#67850,4.);
#11141=VECTOR('',#67853,4.);
#11142=VECTOR('',#67856,4.);
#11143=VECTOR('',#67859,4.);
#11144=VECTOR('',#67862,4.);
#11145=VECTOR('',#67865,4.);
#11146=VECTOR('',#67868,4.);
#11147=VECTOR('',#67871,4.);
#11148=VECTOR('',#67874,4.);
#11149=VECTOR('',#67877,4.);
#11150=VECTOR('',#67880,4.);
#11151=VECTOR('',#67883,4.);
#11152=VECTOR('',#67886,4.);
#11153=VECTOR('',#67889,4.);
#11154=VECTOR('',#67892,4.);
#11155=VECTOR('',#67895,4.);
#11156=VECTOR('',#67898,3.22275);
#11157=VECTOR('',#67903,3.22275);
#11158=VECTOR('',#67906,3.22275);
#11159=VECTOR('',#67909,3.22275);
#11160=VECTOR('',#67912,3.22275);
#11161=VECTOR('',#67915,3.22275);
#11162=VECTOR('',#67918,3.22275);
#11163=VECTOR('',#67921,3.22275);
#11164=VECTOR('',#67924,3.22275);
#11165=VECTOR('',#67927,3.22275);
#11166=VECTOR('',#67930,3.22275);
#11167=VECTOR('',#67933,3.22275);
#11168=VECTOR('',#67936,3.22275);
#11169=VECTOR('',#67939,3.22275);
#11170=VECTOR('',#67942,3.22275);
#11171=VECTOR('',#67945,3.22275);
#11172=VECTOR('',#67948,3.22275);
#11173=VECTOR('',#67951,3.22275);
#11174=VECTOR('',#67954,3.22275);
#11175=VECTOR('',#67957,3.22275);
#11176=VECTOR('',#67960,3.22275);
#11177=VECTOR('',#67963,3.22275);
#11178=VECTOR('',#67966,3.22275);
#11179=VECTOR('',#67999,7.09027674973257);
#11180=VECTOR('',#68004,10.);
#11181=VECTOR('',#68005,10.);
#11182=VECTOR('',#68006,10.);
#11183=VECTOR('',#68009,10.);
#11184=VECTOR('',#68010,10.);
#11185=VECTOR('',#68013,10.);
#11186=VECTOR('',#68014,10.);
#11187=VECTOR('',#68019,5.8);
#11188=VECTOR('',#68026,3.6);
#11189=VECTOR('',#68029,10.);
#11190=VECTOR('',#68030,10.);
#11191=VECTOR('',#68033,10.);
#11192=VECTOR('',#68034,10.);
#11193=VECTOR('',#68037,10.);
#13223=PLANE('',#55241);
#13224=PLANE('',#55244);
#13225=PLANE('',#55254);
#13226=PLANE('',#55258);
#13227=PLANE('',#55259);
#13228=PLANE('',#55260);
#13229=PLANE('',#55263);
#13230=PLANE('',#55266);
#13231=PLANE('',#55267);
#13232=PLANE('',#55268);
#13233=PLANE('',#55269);
#13234=PLANE('',#55270);
#15833=FACE_OUTER_BOUND('',#18594,.T.);
#15834=FACE_OUTER_BOUND('',#18595,.T.);
#15835=FACE_OUTER_BOUND('',#18596,.T.);
#15836=FACE_OUTER_BOUND('',#18597,.T.);
#15837=FACE_OUTER_BOUND('',#18598,.T.);
#15838=FACE_OUTER_BOUND('',#18599,.T.);
#15839=FACE_OUTER_BOUND('',#18600,.T.);
#15840=FACE_OUTER_BOUND('',#18601,.T.);
#15841=FACE_OUTER_BOUND('',#18602,.T.);
#15842=FACE_OUTER_BOUND('',#18603,.T.);
#15843=FACE_OUTER_BOUND('',#18604,.T.);
#15844=FACE_OUTER_BOUND('',#18605,.T.);
#15845=FACE_OUTER_BOUND('',#18606,.T.);
#15846=FACE_OUTER_BOUND('',#18607,.T.);
#15847=FACE_OUTER_BOUND('',#18608,.T.);
#15848=FACE_OUTER_BOUND('',#18609,.T.);
#15849=FACE_OUTER_BOUND('',#18610,.T.);
#15850=FACE_OUTER_BOUND('',#18611,.T.);
#15851=FACE_OUTER_BOUND('',#18612,.T.);
#15852=FACE_OUTER_BOUND('',#18613,.T.);
#15853=FACE_OUTER_BOUND('',#18614,.T.);
#15854=FACE_OUTER_BOUND('',#18615,.T.);
#15855=FACE_OUTER_BOUND('',#18616,.T.);
#15856=FACE_OUTER_BOUND('',#18617,.T.);
#15857=FACE_OUTER_BOUND('',#18618,.T.);
#15858=FACE_OUTER_BOUND('',#18619,.T.);
#15859=FACE_OUTER_BOUND('',#18620,.T.);
#15860=FACE_OUTER_BOUND('',#18621,.T.);
#15861=FACE_OUTER_BOUND('',#18622,.T.);
#15862=FACE_OUTER_BOUND('',#18623,.T.);
#15863=FACE_OUTER_BOUND('',#18624,.T.);
#15864=FACE_OUTER_BOUND('',#18625,.T.);
#15865=FACE_OUTER_BOUND('',#18626,.T.);
#15866=FACE_OUTER_BOUND('',#18627,.T.);
#15867=FACE_OUTER_BOUND('',#18628,.T.);
#15868=FACE_OUTER_BOUND('',#18629,.T.);
#15869=FACE_OUTER_BOUND('',#18630,.T.);
#15870=FACE_OUTER_BOUND('',#18631,.T.);
#15871=FACE_OUTER_BOUND('',#18632,.T.);
#15872=FACE_OUTER_BOUND('',#18633,.T.);
#15873=FACE_OUTER_BOUND('',#18634,.T.);
#15874=FACE_OUTER_BOUND('',#18635,.T.);
#15875=FACE_OUTER_BOUND('',#18636,.T.);
#15876=FACE_OUTER_BOUND('',#18637,.T.);
#15877=FACE_OUTER_BOUND('',#18638,.T.);
#15878=FACE_OUTER_BOUND('',#18639,.T.);
#15879=FACE_OUTER_BOUND('',#18640,.T.);
#15880=FACE_OUTER_BOUND('',#18641,.T.);
#15881=FACE_OUTER_BOUND('',#18642,.T.);
#15882=FACE_OUTER_BOUND('',#18643,.T.);
#15883=FACE_OUTER_BOUND('',#18644,.T.);
#15884=FACE_OUTER_BOUND('',#18645,.T.);
#15885=FACE_OUTER_BOUND('',#18646,.T.);
#15886=FACE_OUTER_BOUND('',#18647,.T.);
#15887=FACE_OUTER_BOUND('',#18649,.T.);
#15888=FACE_OUTER_BOUND('',#18650,.T.);
#15889=FACE_OUTER_BOUND('',#18651,.T.);
#15890=FACE_OUTER_BOUND('',#18652,.T.);
#15891=FACE_OUTER_BOUND('',#18653,.T.);
#15892=FACE_OUTER_BOUND('',#18654,.T.);
#15893=FACE_OUTER_BOUND('',#18655,.T.);
#15894=FACE_OUTER_BOUND('',#18656,.T.);
#15895=FACE_OUTER_BOUND('',#18657,.T.);
#15896=FACE_OUTER_BOUND('',#18658,.T.);
#15897=FACE_OUTER_BOUND('',#18659,.T.);
#15898=FACE_OUTER_BOUND('',#18660,.T.);
#18594=EDGE_LOOP('',(#47613,#47614,#47615,#47616));
#18595=EDGE_LOOP('',(#47617,#47618,#47619,#47620));
#18596=EDGE_LOOP('',(#47621,#47622,#47623,#47624));
#18597=EDGE_LOOP('',(#47625,#47626,#47627,#47628));
#18598=EDGE_LOOP('',(#47629,#47630,#47631,#47632));
#18599=EDGE_LOOP('',(#47633,#47634,#47635,#47636));
#18600=EDGE_LOOP('',(#47637,#47638,#47639,#47640));
#18601=EDGE_LOOP('',(#47641,#47642,#47643,#47644));
#18602=EDGE_LOOP('',(#47645,#47646,#47647,#47648));
#18603=EDGE_LOOP('',(#47649,#47650,#47651,#47652));
#18604=EDGE_LOOP('',(#47653,#47654,#47655,#47656));
#18605=EDGE_LOOP('',(#47657,#47658,#47659,#47660));
#18606=EDGE_LOOP('',(#47661,#47662,#47663,#47664));
#18607=EDGE_LOOP('',(#47665,#47666,#47667,#47668));
#18608=EDGE_LOOP('',(#47669,#47670,#47671,#47672));
#18609=EDGE_LOOP('',(#47673,#47674,#47675,#47676));
#18610=EDGE_LOOP('',(#47677,#47678,#47679,#47680));
#18611=EDGE_LOOP('',(#47681,#47682,#47683,#47684));
#18612=EDGE_LOOP('',(#47685,#47686,#47687,#47688));
#18613=EDGE_LOOP('',(#47689,#47690,#47691,#47692));
#18614=EDGE_LOOP('',(#47693,#47694,#47695,#47696));
#18615=EDGE_LOOP('',(#47697,#47698,#47699,#47700));
#18616=EDGE_LOOP('',(#47701,#47702,#47703,#47704));
#18617=EDGE_LOOP('',(#47705,#47706,#47707,#47708));
#18618=EDGE_LOOP('',(#47709,#47710,#47711,#47712));
#18619=EDGE_LOOP('',(#47713,#47714,#47715,#47716));
#18620=EDGE_LOOP('',(#47717,#47718,#47719,#47720));
#18621=EDGE_LOOP('',(#47721,#47722,#47723,#47724));
#18622=EDGE_LOOP('',(#47725,#47726,#47727,#47728));
#18623=EDGE_LOOP('',(#47729,#47730,#47731,#47732));
#18624=EDGE_LOOP('',(#47733,#47734,#47735,#47736));
#18625=EDGE_LOOP('',(#47737,#47738,#47739,#47740));
#18626=EDGE_LOOP('',(#47741,#47742,#47743,#47744));
#18627=EDGE_LOOP('',(#47745,#47746,#47747,#47748));
#18628=EDGE_LOOP('',(#47749,#47750,#47751,#47752));
#18629=EDGE_LOOP('',(#47753,#47754,#47755,#47756));
#18630=EDGE_LOOP('',(#47757,#47758,#47759,#47760));
#18631=EDGE_LOOP('',(#47761,#47762,#47763,#47764));
#18632=EDGE_LOOP('',(#47765,#47766,#47767,#47768));
#18633=EDGE_LOOP('',(#47769,#47770,#47771,#47772));
#18634=EDGE_LOOP('',(#47773,#47774,#47775,#47776));
#18635=EDGE_LOOP('',(#47777,#47778,#47779,#47780));
#18636=EDGE_LOOP('',(#47781,#47782,#47783,#47784));
#18637=EDGE_LOOP('',(#47785,#47786,#47787,#47788));
#18638=EDGE_LOOP('',(#47789,#47790,#47791,#47792));
#18639=EDGE_LOOP('',(#47793,#47794,#47795,#47796));
#18640=EDGE_LOOP('',(#47797,#47798,#47799,#47800,#47801));
#18641=EDGE_LOOP('',(#47802,#47803,#47804,#47805,#47806,#47807,#47808,#47809,
#47810,#47811,#47812,#47813,#47814,#47815,#47816,#47817,#47818,#47819,#47820,
#47821,#47822,#47823,#47824,#47825,#47826,#47827,#47828,#47829,#47830,#47831,
#47832,#47833,#47834,#47835,#47836,#47837,#47838,#47839,#47840,#47841,#47842,
#47843,#47844,#47845,#47846,#47847,#47848,#47849,#47850,#47851));
#18642=EDGE_LOOP('',(#47852,#47853,#47854,#47855,#47856));
#18643=EDGE_LOOP('',(#47857,#47858,#47859,#47860));
#18644=EDGE_LOOP('',(#47861,#47862,#47863,#47864,#47865,#47866,#47867,#47868,
#47869,#47870,#47871,#47872,#47873,#47874,#47875,#47876,#47877,#47878,#47879,
#47880,#47881,#47882,#47883,#47884,#47885,#47886,#47887,#47888,#47889,#47890,
#47891,#47892,#47893,#47894,#47895,#47896,#47897,#47898,#47899,#47900,#47901,
#47902,#47903,#47904,#47905,#47906,#47907,#47908,#47909,#47910));
#18645=EDGE_LOOP('',(#47911,#47912,#47913,#47914,#47915,#47916));
#18646=EDGE_LOOP('',(#47917,#47918,#47919,#47920));
#18647=EDGE_LOOP('',(#47921));
#18648=EDGE_LOOP('',(#47922));
#18649=EDGE_LOOP('',(#47923,#47924,#47925,#47926,#47927,#47928,#47929,#47930,
#47931));
#18650=EDGE_LOOP('',(#47932,#47933,#47934,#47935));
#18651=EDGE_LOOP('',(#47936,#47937,#47938,#47939));
#18652=EDGE_LOOP('',(#47940,#47941,#47942,#47943));
#18653=EDGE_LOOP('',(#47944,#47945,#47946,#47947));
#18654=EDGE_LOOP('',(#47948));
#18655=EDGE_LOOP('',(#47949,#47950,#47951,#47952,#47953,#47954));
#18656=EDGE_LOOP('',(#47955,#47956,#47957,#47958));
#18657=EDGE_LOOP('',(#47959,#47960,#47961,#47962));
#18658=EDGE_LOOP('',(#47963,#47964,#47965,#47966));
#18659=EDGE_LOOP('',(#47967));
#18660=EDGE_LOOP('',(#47968,#47969,#47970,#47971,#47972,#47973));
#18661=EDGE_LOOP('',(#47974));
#19548=(
BOUNDED_CURVE()
B_SPLINE_CURVE(2,(#93987,#93988,#93989),.UNSPECIFIED.,.F.,.F.)
B_SPLINE_CURVE_WITH_KNOTS((3,3),(0.0802593534055511,0.873558161927064),
 .UNSPECIFIED.)
CURVE()
GEOMETRIC_REPRESENTATION_ITEM()
RATIONAL_B_SPLINE_CURVE((1.03570012424137,1.19592349106096,1.03570012424137))
REPRESENTATION_ITEM('')
);
#19549=(
BOUNDED_CURVE()
B_SPLINE_CURVE(2,(#93991,#93992,#93993),.UNSPECIFIED.,.F.,.F.)
B_SPLINE_CURVE_WITH_KNOTS((3,3),(0.0802593534055511,0.873558161927064),
 .UNSPECIFIED.)
CURVE()
GEOMETRIC_REPRESENTATION_ITEM()
RATIONAL_B_SPLINE_CURVE((1.03570012424137,1.19592349106096,1.03570012424137))
REPRESENTATION_ITEM('')
);
#19550=(
BOUNDED_CURVE()
B_SPLINE_CURVE(2,(#93995,#93996,#93997),.UNSPECIFIED.,.F.,.F.)
B_SPLINE_CURVE_WITH_KNOTS((3,3),(0.0802593534055514,0.873558161927064),
 .UNSPECIFIED.)
CURVE()
GEOMETRIC_REPRESENTATION_ITEM()
RATIONAL_B_SPLINE_CURVE((1.03570012424137,1.19592349106096,1.03570012424137))
REPRESENTATION_ITEM('')
);
#19551=(
BOUNDED_CURVE()
B_SPLINE_CURVE(2,(#93999,#94000,#94001),.UNSPECIFIED.,.F.,.F.)
B_SPLINE_CURVE_WITH_KNOTS((3,3),(0.0802593534055513,0.873558161927064),
 .UNSPECIFIED.)
CURVE()
GEOMETRIC_REPRESENTATION_ITEM()
RATIONAL_B_SPLINE_CURVE((1.03570012424137,1.19592349106096,1.03570012424137))
REPRESENTATION_ITEM('')
);
#19552=(
BOUNDED_CURVE()
B_SPLINE_CURVE(2,(#94003,#94004,#94005),.UNSPECIFIED.,.F.,.F.)
B_SPLINE_CURVE_WITH_KNOTS((3,3),(0.080259353405551,0.873558161927064),
 .UNSPECIFIED.)
CURVE()
GEOMETRIC_REPRESENTATION_ITEM()
RATIONAL_B_SPLINE_CURVE((1.03570012424137,1.19592349106096,1.03570012424137))
REPRESENTATION_ITEM('')
);
#19553=(
BOUNDED_CURVE()
B_SPLINE_CURVE(2,(#94009,#94010,#94011),.UNSPECIFIED.,.F.,.F.)
B_SPLINE_CURVE_WITH_KNOTS((3,3),(0.0802593534055507,0.873558161927063),
 .UNSPECIFIED.)
CURVE()
GEOMETRIC_REPRESENTATION_ITEM()
RATIONAL_B_SPLINE_CURVE((1.03570012424137,1.19592349106096,1.03570012424137))
REPRESENTATION_ITEM('')
);
#20286=CIRCLE('',#55194,3.933);
#20287=CIRCLE('',#55218,3.22275);
#20288=CIRCLE('',#55242,3.933);
#20289=CIRCLE('',#55243,3.933);
#20290=CIRCLE('',#55245,3.933);
#20291=CIRCLE('',#55246,3.933);
#20292=CIRCLE('',#55247,3.22275);
#20293=CIRCLE('',#55250,0.4);
#20294=CIRCLE('',#55251,4.333);
#20295=CIRCLE('',#55252,3.933);
#20296=CIRCLE('',#55255,5.8);
#20297=CIRCLE('',#55257,6.33323321723195);
#20298=CIRCLE('',#55262,5.8);
#20299=CIRCLE('',#55264,3.2);
#25158=VERTEX_POINT('',#90632);
#25159=VERTEX_POINT('',#90633);
#25160=VERTEX_POINT('',#90635);
#25161=VERTEX_POINT('',#90646);
#25162=VERTEX_POINT('',#90656);
#25163=VERTEX_POINT('',#90657);
#25164=VERTEX_POINT('',#90704);
#25165=VERTEX_POINT('',#90705);
#25166=VERTEX_POINT('',#90752);
#25167=VERTEX_POINT('',#90753);
#25168=VERTEX_POINT('',#90806);
#25169=VERTEX_POINT('',#90807);
#25170=VERTEX_POINT('',#90854);
#25171=VERTEX_POINT('',#90855);
#25172=VERTEX_POINT('',#90902);
#25173=VERTEX_POINT('',#90903);
#25174=VERTEX_POINT('',#90956);
#25175=VERTEX_POINT('',#90957);
#25176=VERTEX_POINT('',#91004);
#25177=VERTEX_POINT('',#91005);
#25178=VERTEX_POINT('',#91052);
#25179=VERTEX_POINT('',#91053);
#25180=VERTEX_POINT('',#91100);
#25181=VERTEX_POINT('',#91101);
#25182=VERTEX_POINT('',#91154);
#25183=VERTEX_POINT('',#91155);
#25184=VERTEX_POINT('',#91202);
#25185=VERTEX_POINT('',#91203);
#25186=VERTEX_POINT('',#91250);
#25187=VERTEX_POINT('',#91251);
#25188=VERTEX_POINT('',#91304);
#25189=VERTEX_POINT('',#91305);
#25190=VERTEX_POINT('',#91352);
#25191=VERTEX_POINT('',#91353);
#25192=VERTEX_POINT('',#91400);
#25193=VERTEX_POINT('',#91401);
#25194=VERTEX_POINT('',#91454);
#25195=VERTEX_POINT('',#91455);
#25196=VERTEX_POINT('',#91502);
#25197=VERTEX_POINT('',#91503);
#25198=VERTEX_POINT('',#91550);
#25199=VERTEX_POINT('',#91551);
#25200=VERTEX_POINT('',#91604);
#25201=VERTEX_POINT('',#91605);
#25202=VERTEX_POINT('',#91652);
#25203=VERTEX_POINT('',#91653);
#25204=VERTEX_POINT('',#91700);
#25205=VERTEX_POINT('',#91701);
#25206=VERTEX_POINT('',#91754);
#25207=VERTEX_POINT('',#91755);
#25208=VERTEX_POINT('',#91757);
#25209=VERTEX_POINT('',#91764);
#25210=VERTEX_POINT('',#91772);
#25211=VERTEX_POINT('',#91773);
#25212=VERTEX_POINT('',#91797);
#25213=VERTEX_POINT('',#91798);
#25214=VERTEX_POINT('',#91822);
#25215=VERTEX_POINT('',#91823);
#25216=VERTEX_POINT('',#91846);
#25217=VERTEX_POINT('',#91847);
#25218=VERTEX_POINT('',#91871);
#25219=VERTEX_POINT('',#91872);
#25220=VERTEX_POINT('',#91896);
#25221=VERTEX_POINT('',#91897);
#25222=VERTEX_POINT('',#91920);
#25223=VERTEX_POINT('',#91921);
#25224=VERTEX_POINT('',#91945);
#25225=VERTEX_POINT('',#91946);
#25226=VERTEX_POINT('',#91970);
#25227=VERTEX_POINT('',#91971);
#25228=VERTEX_POINT('',#91994);
#25229=VERTEX_POINT('',#91995);
#25230=VERTEX_POINT('',#92019);
#25231=VERTEX_POINT('',#92020);
#25232=VERTEX_POINT('',#92044);
#25233=VERTEX_POINT('',#92045);
#25234=VERTEX_POINT('',#92068);
#25235=VERTEX_POINT('',#92069);
#25236=VERTEX_POINT('',#92093);
#25237=VERTEX_POINT('',#92094);
#25238=VERTEX_POINT('',#92118);
#25239=VERTEX_POINT('',#92119);
#25240=VERTEX_POINT('',#92142);
#25241=VERTEX_POINT('',#92143);
#25242=VERTEX_POINT('',#92166);
#25243=VERTEX_POINT('',#92167);
#25244=VERTEX_POINT('',#92191);
#25245=VERTEX_POINT('',#92192);
#25246=VERTEX_POINT('',#92216);
#25247=VERTEX_POINT('',#92217);
#25248=VERTEX_POINT('',#92240);
#25249=VERTEX_POINT('',#92241);
#25250=VERTEX_POINT('',#92265);
#25251=VERTEX_POINT('',#92266);
#25252=VERTEX_POINT('',#92290);
#25253=VERTEX_POINT('',#92291);
#25254=VERTEX_POINT('',#92314);
#25255=VERTEX_POINT('',#92412);
#25256=VERTEX_POINT('',#92414);
#25257=VERTEX_POINT('',#93136);
#25258=VERTEX_POINT('',#93244);
#25259=VERTEX_POINT('',#93247);
#25260=VERTEX_POINT('',#93976);
#25261=VERTEX_POINT('',#93982);
#25262=VERTEX_POINT('',#93985);
#25263=VERTEX_POINT('',#93986);
#25264=VERTEX_POINT('',#93990);
#25265=VERTEX_POINT('',#93994);
#25266=VERTEX_POINT('',#93998);
#25267=VERTEX_POINT('',#94002);
#25268=VERTEX_POINT('',#94006);
#25269=VERTEX_POINT('',#94013);
#25270=VERTEX_POINT('',#94015);
#25271=VERTEX_POINT('',#94019);
#25272=VERTEX_POINT('',#94023);
#25273=VERTEX_POINT('',#94027);
#25274=VERTEX_POINT('',#94031);
#25275=VERTEX_POINT('',#94036);
#25276=VERTEX_POINT('',#94040);
#32668=EDGE_CURVE('',#25158,#25159,#6605,.T.);
#32669=EDGE_CURVE('',#25158,#25160,#619,.T.);
#32670=EDGE_CURVE('',#25160,#25161,#20286,.T.);
#32671=EDGE_CURVE('',#25161,#25159,#620,.T.);
#32672=EDGE_CURVE('',#25162,#25163,#6606,.T.);
#32673=EDGE_CURVE('',#25162,#25158,#621,.T.);
#32674=EDGE_CURVE('',#25159,#25163,#622,.T.);
#32675=EDGE_CURVE('',#25164,#25165,#6607,.T.);
#32676=EDGE_CURVE('',#25164,#25162,#623,.T.);
#32677=EDGE_CURVE('',#25163,#25165,#624,.T.);
#32678=EDGE_CURVE('',#25166,#25167,#6608,.T.);
#32679=EDGE_CURVE('',#25166,#25164,#625,.T.);
#32680=EDGE_CURVE('',#25165,#25167,#626,.T.);
#32681=EDGE_CURVE('',#25168,#25169,#6609,.T.);
#32682=EDGE_CURVE('',#25168,#25166,#627,.T.);
#32683=EDGE_CURVE('',#25167,#25169,#628,.T.);
#32684=EDGE_CURVE('',#25170,#25171,#6610,.T.);
#32685=EDGE_CURVE('',#25170,#25168,#629,.T.);
#32686=EDGE_CURVE('',#25169,#25171,#630,.T.);
#32687=EDGE_CURVE('',#25172,#25173,#6611,.T.);
#32688=EDGE_CURVE('',#25172,#25170,#631,.T.);
#32689=EDGE_CURVE('',#25171,#25173,#632,.T.);
#32690=EDGE_CURVE('',#25174,#25175,#6612,.T.);
#32691=EDGE_CURVE('',#25174,#25172,#633,.T.);
#32692=EDGE_CURVE('',#25173,#25175,#634,.T.);
#32693=EDGE_CURVE('',#25176,#25177,#6613,.T.);
#32694=EDGE_CURVE('',#25176,#25174,#635,.T.);
#32695=EDGE_CURVE('',#25175,#25177,#636,.T.);
#32696=EDGE_CURVE('',#25178,#25179,#6614,.T.);
#32697=EDGE_CURVE('',#25178,#25176,#637,.T.);
#32698=EDGE_CURVE('',#25177,#25179,#638,.T.);
#32699=EDGE_CURVE('',#25180,#25181,#6615,.T.);
#32700=EDGE_CURVE('',#25180,#25178,#639,.T.);
#32701=EDGE_CURVE('',#25179,#25181,#640,.T.);
#32702=EDGE_CURVE('',#25182,#25183,#6616,.T.);
#32703=EDGE_CURVE('',#25182,#25180,#641,.T.);
#32704=EDGE_CURVE('',#25181,#25183,#642,.T.);
#32705=EDGE_CURVE('',#25184,#25185,#6617,.T.);
#32706=EDGE_CURVE('',#25184,#25182,#643,.T.);
#32707=EDGE_CURVE('',#25183,#25185,#644,.T.);
#32708=EDGE_CURVE('',#25186,#25187,#6618,.T.);
#32709=EDGE_CURVE('',#25186,#25184,#645,.T.);
#32710=EDGE_CURVE('',#25185,#25187,#646,.T.);
#32711=EDGE_CURVE('',#25188,#25189,#6619,.T.);
#32712=EDGE_CURVE('',#25188,#25186,#647,.T.);
#32713=EDGE_CURVE('',#25187,#25189,#648,.T.);
#32714=EDGE_CURVE('',#25190,#25191,#6620,.T.);
#32715=EDGE_CURVE('',#25190,#25188,#649,.T.);
#32716=EDGE_CURVE('',#25189,#25191,#650,.T.);
#32717=EDGE_CURVE('',#25192,#25193,#6621,.T.);
#32718=EDGE_CURVE('',#25192,#25190,#651,.T.);
#32719=EDGE_CURVE('',#25191,#25193,#652,.T.);
#32720=EDGE_CURVE('',#25194,#25195,#6622,.T.);
#32721=EDGE_CURVE('',#25194,#25192,#653,.T.);
#32722=EDGE_CURVE('',#25193,#25195,#654,.T.);
#32723=EDGE_CURVE('',#25196,#25197,#6623,.T.);
#32724=EDGE_CURVE('',#25196,#25194,#655,.T.);
#32725=EDGE_CURVE('',#25195,#25197,#656,.T.);
#32726=EDGE_CURVE('',#25198,#25199,#6624,.T.);
#32727=EDGE_CURVE('',#25198,#25196,#657,.T.);
#32728=EDGE_CURVE('',#25197,#25199,#658,.T.);
#32729=EDGE_CURVE('',#25200,#25201,#6625,.T.);
#32730=EDGE_CURVE('',#25200,#25198,#659,.T.);
#32731=EDGE_CURVE('',#25199,#25201,#660,.T.);
#32732=EDGE_CURVE('',#25202,#25203,#6626,.T.);
#32733=EDGE_CURVE('',#25202,#25200,#661,.T.);
#32734=EDGE_CURVE('',#25201,#25203,#662,.T.);
#32735=EDGE_CURVE('',#25204,#25205,#6627,.T.);
#32736=EDGE_CURVE('',#25204,#25202,#663,.T.);
#32737=EDGE_CURVE('',#25203,#25205,#664,.T.);
#32738=EDGE_CURVE('',#25206,#25207,#6628,.T.);
#32739=EDGE_CURVE('',#25206,#25208,#665,.T.);
#32740=EDGE_CURVE('',#25209,#25208,#20287,.T.);
#32741=EDGE_CURVE('',#25207,#25209,#666,.T.);
#32742=EDGE_CURVE('',#25210,#25211,#6629,.T.);
#32743=EDGE_CURVE('',#25210,#25206,#667,.T.);
#32744=EDGE_CURVE('',#25211,#25207,#668,.T.);
#32745=EDGE_CURVE('',#25212,#25213,#6630,.T.);
#32746=EDGE_CURVE('',#25212,#25210,#669,.T.);
#32747=EDGE_CURVE('',#25213,#25211,#670,.T.);
#32748=EDGE_CURVE('',#25214,#25215,#6631,.T.);
#32749=EDGE_CURVE('',#25214,#25212,#671,.T.);
#32750=EDGE_CURVE('',#25215,#25213,#672,.T.);
#32751=EDGE_CURVE('',#25216,#25217,#6632,.T.);
#32752=EDGE_CURVE('',#25216,#25214,#673,.T.);
#32753=EDGE_CURVE('',#25217,#25215,#674,.T.);
#32754=EDGE_CURVE('',#25218,#25219,#6633,.T.);
#32755=EDGE_CURVE('',#25218,#25216,#675,.T.);
#32756=EDGE_CURVE('',#25219,#25217,#676,.T.);
#32757=EDGE_CURVE('',#25220,#25221,#6634,.T.);
#32758=EDGE_CURVE('',#25220,#25218,#677,.T.);
#32759=EDGE_CURVE('',#25221,#25219,#678,.T.);
#32760=EDGE_CURVE('',#25222,#25223,#6635,.T.);
#32761=EDGE_CURVE('',#25222,#25220,#679,.T.);
#32762=EDGE_CURVE('',#25223,#25221,#680,.T.);
#32763=EDGE_CURVE('',#25224,#25225,#6636,.T.);
#32764=EDGE_CURVE('',#25224,#25222,#681,.T.);
#32765=EDGE_CURVE('',#25225,#25223,#682,.T.);
#32766=EDGE_CURVE('',#25226,#25227,#6637,.T.);
#32767=EDGE_CURVE('',#25226,#25224,#683,.T.);
#32768=EDGE_CURVE('',#25227,#25225,#684,.T.);
#32769=EDGE_CURVE('',#25228,#25229,#6638,.T.);
#32770=EDGE_CURVE('',#25228,#25226,#685,.T.);
#32771=EDGE_CURVE('',#25229,#25227,#686,.T.);
#32772=EDGE_CURVE('',#25230,#25231,#6639,.T.);
#32773=EDGE_CURVE('',#25230,#25228,#687,.T.);
#32774=EDGE_CURVE('',#25231,#25229,#688,.T.);
#32775=EDGE_CURVE('',#25232,#25233,#6640,.T.);
#32776=EDGE_CURVE('',#25232,#25230,#689,.T.);
#32777=EDGE_CURVE('',#25233,#25231,#690,.T.);
#32778=EDGE_CURVE('',#25234,#25235,#6641,.T.);
#32779=EDGE_CURVE('',#25234,#25232,#691,.T.);
#32780=EDGE_CURVE('',#25235,#25233,#692,.T.);
#32781=EDGE_CURVE('',#25236,#25237,#6642,.T.);
#32782=EDGE_CURVE('',#25236,#25234,#693,.T.);
#32783=EDGE_CURVE('',#25237,#25235,#694,.T.);
#32784=EDGE_CURVE('',#25238,#25239,#6643,.T.);
#32785=EDGE_CURVE('',#25238,#25236,#695,.T.);
#32786=EDGE_CURVE('',#25239,#25237,#696,.T.);
#32787=EDGE_CURVE('',#25240,#25241,#6644,.T.);
#32788=EDGE_CURVE('',#25240,#25238,#697,.T.);
#32789=EDGE_CURVE('',#25241,#25239,#698,.T.);
#32790=EDGE_CURVE('',#25242,#25243,#6645,.T.);
#32791=EDGE_CURVE('',#25242,#25240,#699,.T.);
#32792=EDGE_CURVE('',#25243,#25241,#700,.T.);
#32793=EDGE_CURVE('',#25244,#25245,#6646,.T.);
#32794=EDGE_CURVE('',#25244,#25242,#701,.T.);
#32795=EDGE_CURVE('',#25245,#25243,#702,.T.);
#32796=EDGE_CURVE('',#25246,#25247,#6647,.T.);
#32797=EDGE_CURVE('',#25246,#25244,#703,.T.);
#32798=EDGE_CURVE('',#25247,#25245,#704,.T.);
#32799=EDGE_CURVE('',#25248,#25249,#6648,.T.);
#32800=EDGE_CURVE('',#25248,#25246,#705,.T.);
#32801=EDGE_CURVE('',#25249,#25247,#706,.T.);
#32802=EDGE_CURVE('',#25250,#25251,#6649,.T.);
#32803=EDGE_CURVE('',#25250,#25248,#707,.T.);
#32804=EDGE_CURVE('',#25251,#25249,#708,.T.);
#32805=EDGE_CURVE('',#25252,#25253,#6650,.T.);
#32806=EDGE_CURVE('',#25252,#25250,#709,.T.);
#32807=EDGE_CURVE('',#25253,#25251,#710,.T.);
#32808=EDGE_CURVE('',#25208,#25254,#711,.T.);
#32809=EDGE_CURVE('',#25255,#25254,#20288,.T.);
#32810=EDGE_CURVE('',#25256,#25255,#20289,.T.);
#32811=EDGE_CURVE('',#25256,#25209,#712,.T.);
#32812=EDGE_CURVE('',#25205,#25256,#713,.T.);
#32813=EDGE_CURVE('',#25257,#25161,#714,.T.);
#32814=EDGE_CURVE('',#25257,#25253,#715,.T.);
#32815=EDGE_CURVE('',#25161,#25258,#20290,.T.);
#32816=EDGE_CURVE('',#25258,#25160,#20291,.T.);
#32817=EDGE_CURVE('',#25160,#25259,#716,.T.);
#32818=EDGE_CURVE('',#25259,#25257,#20292,.T.);
#32819=EDGE_CURVE('',#25259,#25252,#717,.T.);
#32820=EDGE_CURVE('',#25254,#25204,#718,.T.);
#32821=EDGE_CURVE('',#25255,#25260,#20293,.T.);
#32822=EDGE_CURVE('',#25260,#25260,#20294,.T.);
#32823=EDGE_CURVE('',#25254,#25256,#20295,.T.);
#32824=EDGE_CURVE('',#25261,#25261,#20296,.T.);
#32825=EDGE_CURVE('',#25262,#25263,#19548,.T.);
#32826=EDGE_CURVE('',#25264,#25262,#19549,.T.);
#32827=EDGE_CURVE('',#25265,#25264,#19550,.T.);
#32828=EDGE_CURVE('',#25266,#25265,#19551,.T.);
#32829=EDGE_CURVE('',#25267,#25266,#19552,.T.);
#32830=EDGE_CURVE('',#25267,#25268,#6651,.T.);
#32831=EDGE_CURVE('',#25268,#25268,#20297,.T.);
#32832=EDGE_CURVE('',#25263,#25267,#19553,.T.);
#32833=EDGE_CURVE('',#25269,#25265,#6652,.T.);
#32834=EDGE_CURVE('',#25269,#25270,#6653,.T.);
#32835=EDGE_CURVE('',#25270,#25266,#6654,.T.);
#32836=EDGE_CURVE('',#25271,#25264,#6655,.T.);
#32837=EDGE_CURVE('',#25271,#25269,#6656,.T.);
#32838=EDGE_CURVE('',#25272,#25262,#6657,.T.);
#32839=EDGE_CURVE('',#25272,#25271,#6658,.T.);
#32840=EDGE_CURVE('',#25273,#25273,#20298,.T.);
#32841=EDGE_CURVE('',#25273,#25261,#6659,.T.);
#32842=EDGE_CURVE('',#25274,#25274,#20299,.T.);
#32843=EDGE_CURVE('',#25258,#25274,#6660,.T.);
#32844=EDGE_CURVE('',#25275,#25263,#6661,.T.);
#32845=EDGE_CURVE('',#25275,#25272,#6662,.T.);
#32846=EDGE_CURVE('',#25276,#25267,#6663,.T.);
#32847=EDGE_CURVE('',#25276,#25275,#6664,.T.);
#32848=EDGE_CURVE('',#25270,#25276,#6665,.T.);
#47613=ORIENTED_EDGE('',*,*,#32668,.F.);
#47614=ORIENTED_EDGE('',*,*,#32669,.T.);
#47615=ORIENTED_EDGE('',*,*,#32670,.T.);
#47616=ORIENTED_EDGE('',*,*,#32671,.T.);
#47617=ORIENTED_EDGE('',*,*,#32672,.F.);
#47618=ORIENTED_EDGE('',*,*,#32673,.T.);
#47619=ORIENTED_EDGE('',*,*,#32668,.T.);
#47620=ORIENTED_EDGE('',*,*,#32674,.T.);
#47621=ORIENTED_EDGE('',*,*,#32675,.F.);
#47622=ORIENTED_EDGE('',*,*,#32676,.T.);
#47623=ORIENTED_EDGE('',*,*,#32672,.T.);
#47624=ORIENTED_EDGE('',*,*,#32677,.T.);
#47625=ORIENTED_EDGE('',*,*,#32678,.F.);
#47626=ORIENTED_EDGE('',*,*,#32679,.T.);
#47627=ORIENTED_EDGE('',*,*,#32675,.T.);
#47628=ORIENTED_EDGE('',*,*,#32680,.T.);
#47629=ORIENTED_EDGE('',*,*,#32681,.F.);
#47630=ORIENTED_EDGE('',*,*,#32682,.T.);
#47631=ORIENTED_EDGE('',*,*,#32678,.T.);
#47632=ORIENTED_EDGE('',*,*,#32683,.T.);
#47633=ORIENTED_EDGE('',*,*,#32684,.F.);
#47634=ORIENTED_EDGE('',*,*,#32685,.T.);
#47635=ORIENTED_EDGE('',*,*,#32681,.T.);
#47636=ORIENTED_EDGE('',*,*,#32686,.T.);
#47637=ORIENTED_EDGE('',*,*,#32687,.F.);
#47638=ORIENTED_EDGE('',*,*,#32688,.T.);
#47639=ORIENTED_EDGE('',*,*,#32684,.T.);
#47640=ORIENTED_EDGE('',*,*,#32689,.T.);
#47641=ORIENTED_EDGE('',*,*,#32690,.F.);
#47642=ORIENTED_EDGE('',*,*,#32691,.T.);
#47643=ORIENTED_EDGE('',*,*,#32687,.T.);
#47644=ORIENTED_EDGE('',*,*,#32692,.T.);
#47645=ORIENTED_EDGE('',*,*,#32693,.F.);
#47646=ORIENTED_EDGE('',*,*,#32694,.T.);
#47647=ORIENTED_EDGE('',*,*,#32690,.T.);
#47648=ORIENTED_EDGE('',*,*,#32695,.T.);
#47649=ORIENTED_EDGE('',*,*,#32696,.F.);
#47650=ORIENTED_EDGE('',*,*,#32697,.T.);
#47651=ORIENTED_EDGE('',*,*,#32693,.T.);
#47652=ORIENTED_EDGE('',*,*,#32698,.T.);
#47653=ORIENTED_EDGE('',*,*,#32699,.F.);
#47654=ORIENTED_EDGE('',*,*,#32700,.T.);
#47655=ORIENTED_EDGE('',*,*,#32696,.T.);
#47656=ORIENTED_EDGE('',*,*,#32701,.T.);
#47657=ORIENTED_EDGE('',*,*,#32702,.F.);
#47658=ORIENTED_EDGE('',*,*,#32703,.T.);
#47659=ORIENTED_EDGE('',*,*,#32699,.T.);
#47660=ORIENTED_EDGE('',*,*,#32704,.T.);
#47661=ORIENTED_EDGE('',*,*,#32705,.F.);
#47662=ORIENTED_EDGE('',*,*,#32706,.T.);
#47663=ORIENTED_EDGE('',*,*,#32702,.T.);
#47664=ORIENTED_EDGE('',*,*,#32707,.T.);
#47665=ORIENTED_EDGE('',*,*,#32708,.F.);
#47666=ORIENTED_EDGE('',*,*,#32709,.T.);
#47667=ORIENTED_EDGE('',*,*,#32705,.T.);
#47668=ORIENTED_EDGE('',*,*,#32710,.T.);
#47669=ORIENTED_EDGE('',*,*,#32711,.F.);
#47670=ORIENTED_EDGE('',*,*,#32712,.T.);
#47671=ORIENTED_EDGE('',*,*,#32708,.T.);
#47672=ORIENTED_EDGE('',*,*,#32713,.T.);
#47673=ORIENTED_EDGE('',*,*,#32714,.F.);
#47674=ORIENTED_EDGE('',*,*,#32715,.T.);
#47675=ORIENTED_EDGE('',*,*,#32711,.T.);
#47676=ORIENTED_EDGE('',*,*,#32716,.T.);
#47677=ORIENTED_EDGE('',*,*,#32717,.F.);
#47678=ORIENTED_EDGE('',*,*,#32718,.T.);
#47679=ORIENTED_EDGE('',*,*,#32714,.T.);
#47680=ORIENTED_EDGE('',*,*,#32719,.T.);
#47681=ORIENTED_EDGE('',*,*,#32720,.F.);
#47682=ORIENTED_EDGE('',*,*,#32721,.T.);
#47683=ORIENTED_EDGE('',*,*,#32717,.T.);
#47684=ORIENTED_EDGE('',*,*,#32722,.T.);
#47685=ORIENTED_EDGE('',*,*,#32723,.F.);
#47686=ORIENTED_EDGE('',*,*,#32724,.T.);
#47687=ORIENTED_EDGE('',*,*,#32720,.T.);
#47688=ORIENTED_EDGE('',*,*,#32725,.T.);
#47689=ORIENTED_EDGE('',*,*,#32726,.F.);
#47690=ORIENTED_EDGE('',*,*,#32727,.T.);
#47691=ORIENTED_EDGE('',*,*,#32723,.T.);
#47692=ORIENTED_EDGE('',*,*,#32728,.T.);
#47693=ORIENTED_EDGE('',*,*,#32729,.F.);
#47694=ORIENTED_EDGE('',*,*,#32730,.T.);
#47695=ORIENTED_EDGE('',*,*,#32726,.T.);
#47696=ORIENTED_EDGE('',*,*,#32731,.T.);
#47697=ORIENTED_EDGE('',*,*,#32732,.F.);
#47698=ORIENTED_EDGE('',*,*,#32733,.T.);
#47699=ORIENTED_EDGE('',*,*,#32729,.T.);
#47700=ORIENTED_EDGE('',*,*,#32734,.T.);
#47701=ORIENTED_EDGE('',*,*,#32735,.F.);
#47702=ORIENTED_EDGE('',*,*,#32736,.T.);
#47703=ORIENTED_EDGE('',*,*,#32732,.T.);
#47704=ORIENTED_EDGE('',*,*,#32737,.T.);
#47705=ORIENTED_EDGE('',*,*,#32738,.F.);
#47706=ORIENTED_EDGE('',*,*,#32739,.T.);
#47707=ORIENTED_EDGE('',*,*,#32740,.F.);
#47708=ORIENTED_EDGE('',*,*,#32741,.F.);
#47709=ORIENTED_EDGE('',*,*,#32742,.F.);
#47710=ORIENTED_EDGE('',*,*,#32743,.T.);
#47711=ORIENTED_EDGE('',*,*,#32738,.T.);
#47712=ORIENTED_EDGE('',*,*,#32744,.F.);
#47713=ORIENTED_EDGE('',*,*,#32745,.F.);
#47714=ORIENTED_EDGE('',*,*,#32746,.T.);
#47715=ORIENTED_EDGE('',*,*,#32742,.T.);
#47716=ORIENTED_EDGE('',*,*,#32747,.F.);
#47717=ORIENTED_EDGE('',*,*,#32748,.F.);
#47718=ORIENTED_EDGE('',*,*,#32749,.T.);
#47719=ORIENTED_EDGE('',*,*,#32745,.T.);
#47720=ORIENTED_EDGE('',*,*,#32750,.F.);
#47721=ORIENTED_EDGE('',*,*,#32751,.F.);
#47722=ORIENTED_EDGE('',*,*,#32752,.T.);
#47723=ORIENTED_EDGE('',*,*,#32748,.T.);
#47724=ORIENTED_EDGE('',*,*,#32753,.F.);
#47725=ORIENTED_EDGE('',*,*,#32754,.F.);
#47726=ORIENTED_EDGE('',*,*,#32755,.T.);
#47727=ORIENTED_EDGE('',*,*,#32751,.T.);
#47728=ORIENTED_EDGE('',*,*,#32756,.F.);
#47729=ORIENTED_EDGE('',*,*,#32757,.F.);
#47730=ORIENTED_EDGE('',*,*,#32758,.T.);
#47731=ORIENTED_EDGE('',*,*,#32754,.T.);
#47732=ORIENTED_EDGE('',*,*,#32759,.F.);
#47733=ORIENTED_EDGE('',*,*,#32760,.F.);
#47734=ORIENTED_EDGE('',*,*,#32761,.T.);
#47735=ORIENTED_EDGE('',*,*,#32757,.T.);
#47736=ORIENTED_EDGE('',*,*,#32762,.F.);
#47737=ORIENTED_EDGE('',*,*,#32763,.F.);
#47738=ORIENTED_EDGE('',*,*,#32764,.T.);
#47739=ORIENTED_EDGE('',*,*,#32760,.T.);
#47740=ORIENTED_EDGE('',*,*,#32765,.F.);
#47741=ORIENTED_EDGE('',*,*,#32766,.F.);
#47742=ORIENTED_EDGE('',*,*,#32767,.T.);
#47743=ORIENTED_EDGE('',*,*,#32763,.T.);
#47744=ORIENTED_EDGE('',*,*,#32768,.F.);
#47745=ORIENTED_EDGE('',*,*,#32769,.F.);
#47746=ORIENTED_EDGE('',*,*,#32770,.T.);
#47747=ORIENTED_EDGE('',*,*,#32766,.T.);
#47748=ORIENTED_EDGE('',*,*,#32771,.F.);
#47749=ORIENTED_EDGE('',*,*,#32772,.F.);
#47750=ORIENTED_EDGE('',*,*,#32773,.T.);
#47751=ORIENTED_EDGE('',*,*,#32769,.T.);
#47752=ORIENTED_EDGE('',*,*,#32774,.F.);
#47753=ORIENTED_EDGE('',*,*,#32775,.F.);
#47754=ORIENTED_EDGE('',*,*,#32776,.T.);
#47755=ORIENTED_EDGE('',*,*,#32772,.T.);
#47756=ORIENTED_EDGE('',*,*,#32777,.F.);
#47757=ORIENTED_EDGE('',*,*,#32778,.F.);
#47758=ORIENTED_EDGE('',*,*,#32779,.T.);
#47759=ORIENTED_EDGE('',*,*,#32775,.T.);
#47760=ORIENTED_EDGE('',*,*,#32780,.F.);
#47761=ORIENTED_EDGE('',*,*,#32781,.F.);
#47762=ORIENTED_EDGE('',*,*,#32782,.T.);
#47763=ORIENTED_EDGE('',*,*,#32778,.T.);
#47764=ORIENTED_EDGE('',*,*,#32783,.F.);
#47765=ORIENTED_EDGE('',*,*,#32784,.F.);
#47766=ORIENTED_EDGE('',*,*,#32785,.T.);
#47767=ORIENTED_EDGE('',*,*,#32781,.T.);
#47768=ORIENTED_EDGE('',*,*,#32786,.F.);
#47769=ORIENTED_EDGE('',*,*,#32787,.F.);
#47770=ORIENTED_EDGE('',*,*,#32788,.T.);
#47771=ORIENTED_EDGE('',*,*,#32784,.T.);
#47772=ORIENTED_EDGE('',*,*,#32789,.F.);
#47773=ORIENTED_EDGE('',*,*,#32790,.F.);
#47774=ORIENTED_EDGE('',*,*,#32791,.T.);
#47775=ORIENTED_EDGE('',*,*,#32787,.T.);
#47776=ORIENTED_EDGE('',*,*,#32792,.F.);
#47777=ORIENTED_EDGE('',*,*,#32793,.F.);
#47778=ORIENTED_EDGE('',*,*,#32794,.T.);
#47779=ORIENTED_EDGE('',*,*,#32790,.T.);
#47780=ORIENTED_EDGE('',*,*,#32795,.F.);
#47781=ORIENTED_EDGE('',*,*,#32796,.F.);
#47782=ORIENTED_EDGE('',*,*,#32797,.T.);
#47783=ORIENTED_EDGE('',*,*,#32793,.T.);
#47784=ORIENTED_EDGE('',*,*,#32798,.F.);
#47785=ORIENTED_EDGE('',*,*,#32799,.F.);
#47786=ORIENTED_EDGE('',*,*,#32800,.T.);
#47787=ORIENTED_EDGE('',*,*,#32796,.T.);
#47788=ORIENTED_EDGE('',*,*,#32801,.F.);
#47789=ORIENTED_EDGE('',*,*,#32802,.F.);
#47790=ORIENTED_EDGE('',*,*,#32803,.T.);
#47791=ORIENTED_EDGE('',*,*,#32799,.T.);
#47792=ORIENTED_EDGE('',*,*,#32804,.F.);
#47793=ORIENTED_EDGE('',*,*,#32805,.F.);
#47794=ORIENTED_EDGE('',*,*,#32806,.T.);
#47795=ORIENTED_EDGE('',*,*,#32802,.T.);
#47796=ORIENTED_EDGE('',*,*,#32807,.F.);
#47797=ORIENTED_EDGE('',*,*,#32740,.T.);
#47798=ORIENTED_EDGE('',*,*,#32808,.T.);
#47799=ORIENTED_EDGE('',*,*,#32809,.F.);
#47800=ORIENTED_EDGE('',*,*,#32810,.F.);
#47801=ORIENTED_EDGE('',*,*,#32811,.T.);
#47802=ORIENTED_EDGE('',*,*,#32811,.F.);
#47803=ORIENTED_EDGE('',*,*,#32812,.F.);
#47804=ORIENTED_EDGE('',*,*,#32737,.F.);
#47805=ORIENTED_EDGE('',*,*,#32734,.F.);
#47806=ORIENTED_EDGE('',*,*,#32731,.F.);
#47807=ORIENTED_EDGE('',*,*,#32728,.F.);
#47808=ORIENTED_EDGE('',*,*,#32725,.F.);
#47809=ORIENTED_EDGE('',*,*,#32722,.F.);
#47810=ORIENTED_EDGE('',*,*,#32719,.F.);
#47811=ORIENTED_EDGE('',*,*,#32716,.F.);
#47812=ORIENTED_EDGE('',*,*,#32713,.F.);
#47813=ORIENTED_EDGE('',*,*,#32710,.F.);
#47814=ORIENTED_EDGE('',*,*,#32707,.F.);
#47815=ORIENTED_EDGE('',*,*,#32704,.F.);
#47816=ORIENTED_EDGE('',*,*,#32701,.F.);
#47817=ORIENTED_EDGE('',*,*,#32698,.F.);
#47818=ORIENTED_EDGE('',*,*,#32695,.F.);
#47819=ORIENTED_EDGE('',*,*,#32692,.F.);
#47820=ORIENTED_EDGE('',*,*,#32689,.F.);
#47821=ORIENTED_EDGE('',*,*,#32686,.F.);
#47822=ORIENTED_EDGE('',*,*,#32683,.F.);
#47823=ORIENTED_EDGE('',*,*,#32680,.F.);
#47824=ORIENTED_EDGE('',*,*,#32677,.F.);
#47825=ORIENTED_EDGE('',*,*,#32674,.F.);
#47826=ORIENTED_EDGE('',*,*,#32671,.F.);
#47827=ORIENTED_EDGE('',*,*,#32813,.F.);
#47828=ORIENTED_EDGE('',*,*,#32814,.T.);
#47829=ORIENTED_EDGE('',*,*,#32807,.T.);
#47830=ORIENTED_EDGE('',*,*,#32804,.T.);
#47831=ORIENTED_EDGE('',*,*,#32801,.T.);
#47832=ORIENTED_EDGE('',*,*,#32798,.T.);
#47833=ORIENTED_EDGE('',*,*,#32795,.T.);
#47834=ORIENTED_EDGE('',*,*,#32792,.T.);
#47835=ORIENTED_EDGE('',*,*,#32789,.T.);
#47836=ORIENTED_EDGE('',*,*,#32786,.T.);
#47837=ORIENTED_EDGE('',*,*,#32783,.T.);
#47838=ORIENTED_EDGE('',*,*,#32780,.T.);
#47839=ORIENTED_EDGE('',*,*,#32777,.T.);
#47840=ORIENTED_EDGE('',*,*,#32774,.T.);
#47841=ORIENTED_EDGE('',*,*,#32771,.T.);
#47842=ORIENTED_EDGE('',*,*,#32768,.T.);
#47843=ORIENTED_EDGE('',*,*,#32765,.T.);
#47844=ORIENTED_EDGE('',*,*,#32762,.T.);
#47845=ORIENTED_EDGE('',*,*,#32759,.T.);
#47846=ORIENTED_EDGE('',*,*,#32756,.T.);
#47847=ORIENTED_EDGE('',*,*,#32753,.T.);
#47848=ORIENTED_EDGE('',*,*,#32750,.T.);
#47849=ORIENTED_EDGE('',*,*,#32747,.T.);
#47850=ORIENTED_EDGE('',*,*,#32744,.T.);
#47851=ORIENTED_EDGE('',*,*,#32741,.T.);
#47852=ORIENTED_EDGE('',*,*,#32815,.T.);
#47853=ORIENTED_EDGE('',*,*,#32816,.T.);
#47854=ORIENTED_EDGE('',*,*,#32817,.T.);
#47855=ORIENTED_EDGE('',*,*,#32818,.T.);
#47856=ORIENTED_EDGE('',*,*,#32813,.T.);
#47857=ORIENTED_EDGE('',*,*,#32805,.T.);
#47858=ORIENTED_EDGE('',*,*,#32814,.F.);
#47859=ORIENTED_EDGE('',*,*,#32818,.F.);
#47860=ORIENTED_EDGE('',*,*,#32819,.T.);
#47861=ORIENTED_EDGE('',*,*,#32808,.F.);
#47862=ORIENTED_EDGE('',*,*,#32739,.F.);
#47863=ORIENTED_EDGE('',*,*,#32743,.F.);
#47864=ORIENTED_EDGE('',*,*,#32746,.F.);
#47865=ORIENTED_EDGE('',*,*,#32749,.F.);
#47866=ORIENTED_EDGE('',*,*,#32752,.F.);
#47867=ORIENTED_EDGE('',*,*,#32755,.F.);
#47868=ORIENTED_EDGE('',*,*,#32758,.F.);
#47869=ORIENTED_EDGE('',*,*,#32761,.F.);
#47870=ORIENTED_EDGE('',*,*,#32764,.F.);
#47871=ORIENTED_EDGE('',*,*,#32767,.F.);
#47872=ORIENTED_EDGE('',*,*,#32770,.F.);
#47873=ORIENTED_EDGE('',*,*,#32773,.F.);
#47874=ORIENTED_EDGE('',*,*,#32776,.F.);
#47875=ORIENTED_EDGE('',*,*,#32779,.F.);
#47876=ORIENTED_EDGE('',*,*,#32782,.F.);
#47877=ORIENTED_EDGE('',*,*,#32785,.F.);
#47878=ORIENTED_EDGE('',*,*,#32788,.F.);
#47879=ORIENTED_EDGE('',*,*,#32791,.F.);
#47880=ORIENTED_EDGE('',*,*,#32794,.F.);
#47881=ORIENTED_EDGE('',*,*,#32797,.F.);
#47882=ORIENTED_EDGE('',*,*,#32800,.F.);
#47883=ORIENTED_EDGE('',*,*,#32803,.F.);
#47884=ORIENTED_EDGE('',*,*,#32806,.F.);
#47885=ORIENTED_EDGE('',*,*,#32819,.F.);
#47886=ORIENTED_EDGE('',*,*,#32817,.F.);
#47887=ORIENTED_EDGE('',*,*,#32669,.F.);
#47888=ORIENTED_EDGE('',*,*,#32673,.F.);
#47889=ORIENTED_EDGE('',*,*,#32676,.F.);
#47890=ORIENTED_EDGE('',*,*,#32679,.F.);
#47891=ORIENTED_EDGE('',*,*,#32682,.F.);
#47892=ORIENTED_EDGE('',*,*,#32685,.F.);
#47893=ORIENTED_EDGE('',*,*,#32688,.F.);
#47894=ORIENTED_EDGE('',*,*,#32691,.F.);
#47895=ORIENTED_EDGE('',*,*,#32694,.F.);
#47896=ORIENTED_EDGE('',*,*,#32697,.F.);
#47897=ORIENTED_EDGE('',*,*,#32700,.F.);
#47898=ORIENTED_EDGE('',*,*,#32703,.F.);
#47899=ORIENTED_EDGE('',*,*,#32706,.F.);
#47900=ORIENTED_EDGE('',*,*,#32709,.F.);
#47901=ORIENTED_EDGE('',*,*,#32712,.F.);
#47902=ORIENTED_EDGE('',*,*,#32715,.F.);
#47903=ORIENTED_EDGE('',*,*,#32718,.F.);
#47904=ORIENTED_EDGE('',*,*,#32721,.F.);
#47905=ORIENTED_EDGE('',*,*,#32724,.F.);
#47906=ORIENTED_EDGE('',*,*,#32727,.F.);
#47907=ORIENTED_EDGE('',*,*,#32730,.F.);
#47908=ORIENTED_EDGE('',*,*,#32733,.F.);
#47909=ORIENTED_EDGE('',*,*,#32736,.F.);
#47910=ORIENTED_EDGE('',*,*,#32820,.F.);
#47911=ORIENTED_EDGE('',*,*,#32810,.T.);
#47912=ORIENTED_EDGE('',*,*,#32821,.T.);
#47913=ORIENTED_EDGE('',*,*,#32822,.T.);
#47914=ORIENTED_EDGE('',*,*,#32821,.F.);
#47915=ORIENTED_EDGE('',*,*,#32809,.T.);
#47916=ORIENTED_EDGE('',*,*,#32823,.T.);
#47917=ORIENTED_EDGE('',*,*,#32735,.T.);
#47918=ORIENTED_EDGE('',*,*,#32812,.T.);
#47919=ORIENTED_EDGE('',*,*,#32823,.F.);
#47920=ORIENTED_EDGE('',*,*,#32820,.T.);
#47921=ORIENTED_EDGE('',*,*,#32824,.F.);
#47922=ORIENTED_EDGE('',*,*,#32822,.F.);
#47923=ORIENTED_EDGE('',*,*,#32825,.F.);
#47924=ORIENTED_EDGE('',*,*,#32826,.F.);
#47925=ORIENTED_EDGE('',*,*,#32827,.F.);
#47926=ORIENTED_EDGE('',*,*,#32828,.F.);
#47927=ORIENTED_EDGE('',*,*,#32829,.F.);
#47928=ORIENTED_EDGE('',*,*,#32830,.T.);
#47929=ORIENTED_EDGE('',*,*,#32831,.F.);
#47930=ORIENTED_EDGE('',*,*,#32830,.F.);
#47931=ORIENTED_EDGE('',*,*,#32832,.F.);
#47932=ORIENTED_EDGE('',*,*,#32828,.T.);
#47933=ORIENTED_EDGE('',*,*,#32833,.F.);
#47934=ORIENTED_EDGE('',*,*,#32834,.T.);
#47935=ORIENTED_EDGE('',*,*,#32835,.T.);
#47936=ORIENTED_EDGE('',*,*,#32827,.T.);
#47937=ORIENTED_EDGE('',*,*,#32836,.F.);
#47938=ORIENTED_EDGE('',*,*,#32837,.T.);
#47939=ORIENTED_EDGE('',*,*,#32833,.T.);
#47940=ORIENTED_EDGE('',*,*,#32826,.T.);
#47941=ORIENTED_EDGE('',*,*,#32838,.F.);
#47942=ORIENTED_EDGE('',*,*,#32839,.T.);
#47943=ORIENTED_EDGE('',*,*,#32836,.T.);
#47944=ORIENTED_EDGE('',*,*,#32840,.F.);
#47945=ORIENTED_EDGE('',*,*,#32841,.T.);
#47946=ORIENTED_EDGE('',*,*,#32824,.T.);
#47947=ORIENTED_EDGE('',*,*,#32841,.F.);
#47948=ORIENTED_EDGE('',*,*,#32842,.F.);
#47949=ORIENTED_EDGE('',*,*,#32815,.F.);
#47950=ORIENTED_EDGE('',*,*,#32670,.F.);
#47951=ORIENTED_EDGE('',*,*,#32816,.F.);
#47952=ORIENTED_EDGE('',*,*,#32843,.T.);
#47953=ORIENTED_EDGE('',*,*,#32842,.T.);
#47954=ORIENTED_EDGE('',*,*,#32843,.F.);
#47955=ORIENTED_EDGE('',*,*,#32825,.T.);
#47956=ORIENTED_EDGE('',*,*,#32844,.F.);
#47957=ORIENTED_EDGE('',*,*,#32845,.T.);
#47958=ORIENTED_EDGE('',*,*,#32838,.T.);
#47959=ORIENTED_EDGE('',*,*,#32832,.T.);
#47960=ORIENTED_EDGE('',*,*,#32846,.F.);
#47961=ORIENTED_EDGE('',*,*,#32847,.T.);
#47962=ORIENTED_EDGE('',*,*,#32844,.T.);
#47963=ORIENTED_EDGE('',*,*,#32829,.T.);
#47964=ORIENTED_EDGE('',*,*,#32835,.F.);
#47965=ORIENTED_EDGE('',*,*,#32848,.T.);
#47966=ORIENTED_EDGE('',*,*,#32846,.T.);
#47967=ORIENTED_EDGE('',*,*,#32831,.T.);
#47968=ORIENTED_EDGE('',*,*,#32839,.F.);
#47969=ORIENTED_EDGE('',*,*,#32845,.F.);
#47970=ORIENTED_EDGE('',*,*,#32847,.F.);
#47971=ORIENTED_EDGE('',*,*,#32848,.F.);
#47972=ORIENTED_EDGE('',*,*,#32834,.F.);
#47973=ORIENTED_EDGE('',*,*,#32837,.F.);
#47974=ORIENTED_EDGE('',*,*,#32840,.T.);
#48322=CONICAL_SURFACE('',#55256,7.09027674973257,1.0071944566367);
#48323=CONICAL_SURFACE('',#55265,3.6,0.785398163397448);
#50920=ADVANCED_FACE('',(#15833),#1233,.T.);
#50921=ADVANCED_FACE('',(#15834),#1234,.T.);
#50922=ADVANCED_FACE('',(#15835),#1235,.T.);
#50923=ADVANCED_FACE('',(#15836),#1236,.T.);
#50924=ADVANCED_FACE('',(#15837),#1237,.T.);
#50925=ADVANCED_FACE('',(#15838),#1238,.T.);
#50926=ADVANCED_FACE('',(#15839),#1239,.T.);
#50927=ADVANCED_FACE('',(#15840),#1240,.T.);
#50928=ADVANCED_FACE('',(#15841),#1241,.T.);
#50929=ADVANCED_FACE('',(#15842),#1242,.T.);
#50930=ADVANCED_FACE('',(#15843),#1243,.T.);
#50931=ADVANCED_FACE('',(#15844),#1244,.T.);
#50932=ADVANCED_FACE('',(#15845),#1245,.T.);
#50933=ADVANCED_FACE('',(#15846),#1246,.T.);
#50934=ADVANCED_FACE('',(#15847),#1247,.T.);
#50935=ADVANCED_FACE('',(#15848),#1248,.T.);
#50936=ADVANCED_FACE('',(#15849),#1249,.T.);
#50937=ADVANCED_FACE('',(#15850),#1250,.T.);
#50938=ADVANCED_FACE('',(#15851),#1251,.T.);
#50939=ADVANCED_FACE('',(#15852),#1252,.T.);
#50940=ADVANCED_FACE('',(#15853),#1253,.T.);
#50941=ADVANCED_FACE('',(#15854),#1254,.T.);
#50942=ADVANCED_FACE('',(#15855),#1255,.T.);
#50943=ADVANCED_FACE('',(#15856),#1256,.T.);
#50944=ADVANCED_FACE('',(#15857),#1257,.T.);
#50945=ADVANCED_FACE('',(#15858),#1258,.T.);
#50946=ADVANCED_FACE('',(#15859),#1259,.T.);
#50947=ADVANCED_FACE('',(#15860),#1260,.T.);
#50948=ADVANCED_FACE('',(#15861),#1261,.T.);
#50949=ADVANCED_FACE('',(#15862),#1262,.T.);
#50950=ADVANCED_FACE('',(#15863),#1263,.T.);
#50951=ADVANCED_FACE('',(#15864),#1264,.T.);
#50952=ADVANCED_FACE('',(#15865),#1265,.T.);
#50953=ADVANCED_FACE('',(#15866),#1266,.T.);
#50954=ADVANCED_FACE('',(#15867),#1267,.T.);
#50955=ADVANCED_FACE('',(#15868),#1268,.T.);
#50956=ADVANCED_FACE('',(#15869),#1269,.T.);
#50957=ADVANCED_FACE('',(#15870),#1270,.T.);
#50958=ADVANCED_FACE('',(#15871),#1271,.T.);
#50959=ADVANCED_FACE('',(#15872),#1272,.T.);
#50960=ADVANCED_FACE('',(#15873),#1273,.T.);
#50961=ADVANCED_FACE('',(#15874),#1274,.T.);
#50962=ADVANCED_FACE('',(#15875),#1275,.T.);
#50963=ADVANCED_FACE('',(#15876),#1276,.T.);
#50964=ADVANCED_FACE('',(#15877),#1277,.T.);
#50965=ADVANCED_FACE('',(#15878),#1278,.T.);
#50966=ADVANCED_FACE('',(#15879),#13223,.F.);
#50967=ADVANCED_FACE('',(#15880),#889,.F.);
#50968=ADVANCED_FACE('',(#15881),#13224,.T.);
#50969=ADVANCED_FACE('',(#15882),#1279,.T.);
#50970=ADVANCED_FACE('',(#15883),#890,.F.);
#50971=ADVANCED_FACE('',(#15884),#958,.F.);
#50972=ADVANCED_FACE('',(#15885),#1280,.T.);
#50973=ADVANCED_FACE('',(#15886,#1038),#13225,.T.);
#50974=ADVANCED_FACE('',(#15887),#48322,.T.);
#50975=ADVANCED_FACE('',(#15888),#13226,.T.);
#50976=ADVANCED_FACE('',(#15889),#13227,.T.);
#50977=ADVANCED_FACE('',(#15890),#13228,.T.);
#50978=ADVANCED_FACE('',(#15891),#1281,.T.);
#50979=ADVANCED_FACE('',(#15892),#13229,.T.);
#50980=ADVANCED_FACE('',(#15893),#48323,.T.);
#50981=ADVANCED_FACE('',(#15894),#13230,.T.);
#50982=ADVANCED_FACE('',(#15895),#13231,.T.);
#50983=ADVANCED_FACE('',(#15896),#13232,.T.);
#50984=ADVANCED_FACE('',(#15897),#13233,.T.);
#50985=ADVANCED_FACE('',(#15898,#1039),#13234,.F.);
#51028=CLOSED_SHELL('',(#50920,#50921,#50922,#50923,#50924,#50925,#50926,
#50927,#50928,#50929,#50930,#50931,#50932,#50933,#50934,#50935,#50936,#50937,
#50938,#50939,#50940,#50941,#50942,#50943,#50944,#50945,#50946,#50947,#50948,
#50949,#50950,#50951,#50952,#50953,#50954,#50955,#50956,#50957,#50958,#50959,
#50960,#50961,#50962,#50963,#50964,#50965,#50966,#50967,#50968,#50969,#50970,
#50971,#50972,#50973,#50974,#50975,#50976,#50977,#50978,#50979,#50980,#50981,
#50982,#50983,#50984,#50985));
#55192=AXIS2_PLACEMENT_3D('',#90630,#67823,#67824);
#55193=AXIS2_PLACEMENT_3D('',#90631,#67825,#67826);
#55194=AXIS2_PLACEMENT_3D('',#90647,#67828,#67829);
#55195=AXIS2_PLACEMENT_3D('',#90655,#67830,#67831);
#55196=AXIS2_PLACEMENT_3D('',#90703,#67833,#67834);
#55197=AXIS2_PLACEMENT_3D('',#90751,#67836,#67837);
#55198=AXIS2_PLACEMENT_3D('',#90805,#67839,#67840);
#55199=AXIS2_PLACEMENT_3D('',#90853,#67842,#67843);
#55200=AXIS2_PLACEMENT_3D('',#90901,#67845,#67846);
#55201=AXIS2_PLACEMENT_3D('',#90955,#67848,#67849);
#55202=AXIS2_PLACEMENT_3D('',#91003,#67851,#67852);
#55203=AXIS2_PLACEMENT_3D('',#91051,#67854,#67855);
#55204=AXIS2_PLACEMENT_3D('',#91099,#67857,#67858);
#55205=AXIS2_PLACEMENT_3D('',#91153,#67860,#67861);
#55206=AXIS2_PLACEMENT_3D('',#91201,#67863,#67864);
#55207=AXIS2_PLACEMENT_3D('',#91249,#67866,#67867);
#55208=AXIS2_PLACEMENT_3D('',#91303,#67869,#67870);
#55209=AXIS2_PLACEMENT_3D('',#91351,#67872,#67873);
#55210=AXIS2_PLACEMENT_3D('',#91399,#67875,#67876);
#55211=AXIS2_PLACEMENT_3D('',#91453,#67878,#67879);
#55212=AXIS2_PLACEMENT_3D('',#91501,#67881,#67882);
#55213=AXIS2_PLACEMENT_3D('',#91549,#67884,#67885);
#55214=AXIS2_PLACEMENT_3D('',#91603,#67887,#67888);
#55215=AXIS2_PLACEMENT_3D('',#91651,#67890,#67891);
#55216=AXIS2_PLACEMENT_3D('',#91699,#67893,#67894);
#55217=AXIS2_PLACEMENT_3D('',#91753,#67896,#67897);
#55218=AXIS2_PLACEMENT_3D('',#91765,#67899,#67900);
#55219=AXIS2_PLACEMENT_3D('',#91771,#67901,#67902);
#55220=AXIS2_PLACEMENT_3D('',#91796,#67904,#67905);
#55221=AXIS2_PLACEMENT_3D('',#91821,#67907,#67908);
#55222=AXIS2_PLACEMENT_3D('',#91845,#67910,#67911);
#55223=AXIS2_PLACEMENT_3D('',#91870,#67913,#67914);
#55224=AXIS2_PLACEMENT_3D('',#91895,#67916,#67917);
#55225=AXIS2_PLACEMENT_3D('',#91919,#67919,#67920);
#55226=AXIS2_PLACEMENT_3D('',#91944,#67922,#67923);
#55227=AXIS2_PLACEMENT_3D('',#91969,#67925,#67926);
#55228=AXIS2_PLACEMENT_3D('',#91993,#67928,#67929);
#55229=AXIS2_PLACEMENT_3D('',#92018,#67931,#67932);
#55230=AXIS2_PLACEMENT_3D('',#92043,#67934,#67935);
#55231=AXIS2_PLACEMENT_3D('',#92067,#67937,#67938);
#55232=AXIS2_PLACEMENT_3D('',#92092,#67940,#67941);
#55233=AXIS2_PLACEMENT_3D('',#92117,#67943,#67944);
#55234=AXIS2_PLACEMENT_3D('',#92141,#67946,#67947);
#55235=AXIS2_PLACEMENT_3D('',#92165,#67949,#67950);
#55236=AXIS2_PLACEMENT_3D('',#92190,#67952,#67953);
#55237=AXIS2_PLACEMENT_3D('',#92215,#67955,#67956);
#55238=AXIS2_PLACEMENT_3D('',#92239,#67958,#67959);
#55239=AXIS2_PLACEMENT_3D('',#92264,#67961,#67962);
#55240=AXIS2_PLACEMENT_3D('',#92289,#67964,#67965);
#55241=AXIS2_PLACEMENT_3D('',#92313,#67967,#67968);
#55242=AXIS2_PLACEMENT_3D('',#92413,#67969,#67970);
#55243=AXIS2_PLACEMENT_3D('',#92415,#67971,#67972);
#55244=AXIS2_PLACEMENT_3D('',#93243,#67973,#67974);
#55245=AXIS2_PLACEMENT_3D('',#93245,#67975,#67976);
#55246=AXIS2_PLACEMENT_3D('',#93246,#67977,#67978);
#55247=AXIS2_PLACEMENT_3D('',#93345,#67979,#67980);
#55248=AXIS2_PLACEMENT_3D('',#93346,#67981,#67982);
#55249=AXIS2_PLACEMENT_3D('',#93975,#67983,#67984);
#55250=AXIS2_PLACEMENT_3D('',#93977,#67985,#67986);
#55251=AXIS2_PLACEMENT_3D('',#93978,#67987,#67988);
#55252=AXIS2_PLACEMENT_3D('',#93979,#67989,#67990);
#55253=AXIS2_PLACEMENT_3D('',#93980,#67991,#67992);
#55254=AXIS2_PLACEMENT_3D('',#93981,#67993,#67994);
#55255=AXIS2_PLACEMENT_3D('',#93983,#67995,#67996);
#55256=AXIS2_PLACEMENT_3D('',#93984,#67997,#67998);
#55257=AXIS2_PLACEMENT_3D('',#94008,#68000,#68001);
#55258=AXIS2_PLACEMENT_3D('',#94012,#68002,#68003);
#55259=AXIS2_PLACEMENT_3D('',#94018,#68007,#68008);
#55260=AXIS2_PLACEMENT_3D('',#94022,#68011,#68012);
#55261=AXIS2_PLACEMENT_3D('',#94026,#68015,#68016);
#55262=AXIS2_PLACEMENT_3D('',#94028,#68017,#68018);
#55263=AXIS2_PLACEMENT_3D('',#94030,#68020,#68021);
#55264=AXIS2_PLACEMENT_3D('',#94032,#68022,#68023);
#55265=AXIS2_PLACEMENT_3D('',#94033,#68024,#68025);
#55266=AXIS2_PLACEMENT_3D('',#94035,#68027,#68028);
#55267=AXIS2_PLACEMENT_3D('',#94039,#68031,#68032);
#55268=AXIS2_PLACEMENT_3D('',#94043,#68035,#68036);
#55269=AXIS2_PLACEMENT_3D('',#94045,#68038,#68039);
#55270=AXIS2_PLACEMENT_3D('',#94046,#68040,#68041);
#67823=DIRECTION('axis',(0.,0.,1.));
#67824=DIRECTION('refdir',(1.,0.,0.));
#67825=DIRECTION('center_axis',(1.,0.,0.));
#67826=DIRECTION('ref_axis',(0.,1.,0.));
#67827=DIRECTION('',(-1.,0.,0.));
#67828=DIRECTION('center_axis',(1.,0.,0.));
#67829=DIRECTION('ref_axis',(0.,1.,0.));
#67830=DIRECTION('center_axis',(1.,0.,0.));
#67831=DIRECTION('ref_axis',(0.,1.,0.));
#67832=DIRECTION('',(-1.,0.,0.));
#67833=DIRECTION('center_axis',(1.,0.,0.));
#67834=DIRECTION('ref_axis',(0.,1.,0.));
#67835=DIRECTION('',(-1.,0.,0.));
#67836=DIRECTION('center_axis',(1.,0.,0.));
#67837=DIRECTION('ref_axis',(0.,1.,0.));
#67838=DIRECTION('',(-1.,0.,0.));
#67839=DIRECTION('center_axis',(1.,0.,0.));
#67840=DIRECTION('ref_axis',(0.,1.,0.));
#67841=DIRECTION('',(-1.,0.,0.));
#67842=DIRECTION('center_axis',(1.,0.,0.));
#67843=DIRECTION('ref_axis',(0.,1.,0.));
#67844=DIRECTION('',(-1.,0.,0.));
#67845=DIRECTION('center_axis',(1.,0.,0.));
#67846=DIRECTION('ref_axis',(0.,1.,0.));
#67847=DIRECTION('',(-1.,0.,0.));
#67848=DIRECTION('center_axis',(1.,0.,0.));
#67849=DIRECTION('ref_axis',(0.,1.,0.));
#67850=DIRECTION('',(-1.,0.,0.));
#67851=DIRECTION('center_axis',(1.,0.,0.));
#67852=DIRECTION('ref_axis',(0.,1.,0.));
#67853=DIRECTION('',(-1.,0.,0.));
#67854=DIRECTION('center_axis',(1.,0.,0.));
#67855=DIRECTION('ref_axis',(0.,1.,0.));
#67856=DIRECTION('',(-1.,0.,0.));
#67857=DIRECTION('center_axis',(1.,0.,0.));
#67858=DIRECTION('ref_axis',(0.,1.,0.));
#67859=DIRECTION('',(-1.,0.,0.));
#67860=DIRECTION('center_axis',(1.,0.,0.));
#67861=DIRECTION('ref_axis',(0.,1.,0.));
#67862=DIRECTION('',(-1.,0.,0.));
#67863=DIRECTION('center_axis',(1.,0.,0.));
#67864=DIRECTION('ref_axis',(0.,1.,0.));
#67865=DIRECTION('',(-1.,0.,0.));
#67866=DIRECTION('center_axis',(1.,0.,0.));
#67867=DIRECTION('ref_axis',(0.,1.,0.));
#67868=DIRECTION('',(-1.,0.,0.));
#67869=DIRECTION('center_axis',(1.,0.,0.));
#67870=DIRECTION('ref_axis',(0.,1.,0.));
#67871=DIRECTION('',(-1.,0.,0.));
#67872=DIRECTION('center_axis',(1.,0.,0.));
#67873=DIRECTION('ref_axis',(0.,1.,0.));
#67874=DIRECTION('',(-1.,0.,0.));
#67875=DIRECTION('center_axis',(1.,0.,0.));
#67876=DIRECTION('ref_axis',(0.,1.,0.));
#67877=DIRECTION('',(-1.,0.,0.));
#67878=DIRECTION('center_axis',(1.,0.,0.));
#67879=DIRECTION('ref_axis',(0.,1.,0.));
#67880=DIRECTION('',(-1.,0.,0.));
#67881=DIRECTION('center_axis',(1.,0.,0.));
#67882=DIRECTION('ref_axis',(0.,1.,0.));
#67883=DIRECTION('',(-1.,0.,0.));
#67884=DIRECTION('center_axis',(1.,0.,0.));
#67885=DIRECTION('ref_axis',(0.,1.,0.));
#67886=DIRECTION('',(-1.,0.,0.));
#67887=DIRECTION('center_axis',(1.,0.,0.));
#67888=DIRECTION('ref_axis',(0.,1.,0.));
#67889=DIRECTION('',(-1.,0.,0.));
#67890=DIRECTION('center_axis',(1.,0.,0.));
#67891=DIRECTION('ref_axis',(0.,1.,0.));
#67892=DIRECTION('',(-1.,0.,0.));
#67893=DIRECTION('center_axis',(1.,0.,0.));
#67894=DIRECTION('ref_axis',(0.,1.,0.));
#67895=DIRECTION('',(-1.,0.,0.));
#67896=DIRECTION('center_axis',(1.,0.,0.));
#67897=DIRECTION('ref_axis',(0.,-0.18069699119509,-0.983538813353617));
#67898=DIRECTION('',(1.,0.,0.));
#67899=DIRECTION('center_axis',(1.,0.,0.));
#67900=DIRECTION('ref_axis',(0.,1.,4.63459159752748E-15));
#67901=DIRECTION('center_axis',(1.,0.,0.));
#67902=DIRECTION('ref_axis',(0.,1.,4.63459159752748E-15));
#67903=DIRECTION('',(1.,0.,0.));
#67904=DIRECTION('center_axis',(1.,0.,0.));
#67905=DIRECTION('ref_axis',(0.,1.,4.63459159752748E-15));
#67906=DIRECTION('',(1.,0.,0.));
#67907=DIRECTION('center_axis',(1.,0.,0.));
#67908=DIRECTION('ref_axis',(0.,1.,4.63459159752748E-15));
#67909=DIRECTION('',(1.,0.,0.));
#67910=DIRECTION('center_axis',(1.,0.,0.));
#67911=DIRECTION('ref_axis',(0.,1.,4.63459159752748E-15));
#67912=DIRECTION('',(1.,0.,0.));
#67913=DIRECTION('center_axis',(1.,0.,0.));
#67914=DIRECTION('ref_axis',(0.,1.,4.63459159752748E-15));
#67915=DIRECTION('',(1.,0.,0.));
#67916=DIRECTION('center_axis',(1.,0.,0.));
#67917=DIRECTION('ref_axis',(0.,1.,4.63459159752748E-15));
#67918=DIRECTION('',(1.,0.,0.));
#67919=DIRECTION('center_axis',(1.,0.,0.));
#67920=DIRECTION('ref_axis',(0.,1.,4.63459159752748E-15));
#67921=DIRECTION('',(1.,0.,0.));
#67922=DIRECTION('center_axis',(1.,0.,0.));
#67923=DIRECTION('ref_axis',(0.,1.,4.63459159752748E-15));
#67924=DIRECTION('',(1.,0.,0.));
#67925=DIRECTION('center_axis',(1.,0.,0.));
#67926=DIRECTION('ref_axis',(0.,1.,4.63459159752748E-15));
#67927=DIRECTION('',(1.,0.,0.));
#67928=DIRECTION('center_axis',(1.,0.,0.));
#67929=DIRECTION('ref_axis',(0.,1.,4.63459159752748E-15));
#67930=DIRECTION('',(1.,0.,0.));
#67931=DIRECTION('center_axis',(1.,0.,0.));
#67932=DIRECTION('ref_axis',(0.,1.,4.63459159752748E-15));
#67933=DIRECTION('',(1.,0.,0.));
#67934=DIRECTION('center_axis',(1.,0.,0.));
#67935=DIRECTION('ref_axis',(0.,1.,4.63459159752748E-15));
#67936=DIRECTION('',(1.,0.,0.));
#67937=DIRECTION('center_axis',(1.,0.,0.));
#67938=DIRECTION('ref_axis',(0.,1.,4.63459159752748E-15));
#67939=DIRECTION('',(1.,0.,0.));
#67940=DIRECTION('center_axis',(1.,0.,0.));
#67941=DIRECTION('ref_axis',(0.,1.,4.63459159752748E-15));
#67942=DIRECTION('',(1.,0.,0.));
#67943=DIRECTION('center_axis',(1.,0.,0.));
#67944=DIRECTION('ref_axis',(0.,1.,4.63459159752748E-15));
#67945=DIRECTION('',(1.,0.,0.));
#67946=DIRECTION('center_axis',(1.,0.,0.));
#67947=DIRECTION('ref_axis',(0.,1.,4.63459159752748E-15));
#67948=DIRECTION('',(1.,0.,0.));
#67949=DIRECTION('center_axis',(1.,0.,0.));
#67950=DIRECTION('ref_axis',(0.,1.,4.63459159752748E-15));
#67951=DIRECTION('',(1.,0.,0.));
#67952=DIRECTION('center_axis',(1.,0.,0.));
#67953=DIRECTION('ref_axis',(0.,1.,4.63459159752748E-15));
#67954=DIRECTION('',(1.,0.,0.));
#67955=DIRECTION('center_axis',(1.,0.,0.));
#67956=DIRECTION('ref_axis',(0.,1.,4.63459159752748E-15));
#67957=DIRECTION('',(1.,0.,0.));
#67958=DIRECTION('center_axis',(1.,0.,0.));
#67959=DIRECTION('ref_axis',(0.,1.,4.63459159752748E-15));
#67960=DIRECTION('',(1.,0.,0.));
#67961=DIRECTION('center_axis',(1.,0.,0.));
#67962=DIRECTION('ref_axis',(0.,1.,4.63459159752748E-15));
#67963=DIRECTION('',(1.,0.,0.));
#67964=DIRECTION('center_axis',(1.,0.,0.));
#67965=DIRECTION('ref_axis',(0.,1.,4.63459159752748E-15));
#67966=DIRECTION('',(1.,0.,0.));
#67967=DIRECTION('center_axis',(1.,0.,0.));
#67968=DIRECTION('ref_axis',(0.,0.,-1.));
#67969=DIRECTION('center_axis',(1.,0.,0.));
#67970=DIRECTION('ref_axis',(0.,1.,0.));
#67971=DIRECTION('center_axis',(1.,0.,0.));
#67972=DIRECTION('ref_axis',(0.,1.,0.));
#67973=DIRECTION('center_axis',(1.,0.,0.));
#67974=DIRECTION('ref_axis',(0.,0.,-1.));
#67975=DIRECTION('center_axis',(1.,0.,0.));
#67976=DIRECTION('ref_axis',(0.,1.,0.));
#67977=DIRECTION('center_axis',(1.,0.,0.));
#67978=DIRECTION('ref_axis',(0.,1.,0.));
#67979=DIRECTION('center_axis',(-1.,0.,0.));
#67980=DIRECTION('ref_axis',(0.,1.,4.63459159752748E-15));
#67981=DIRECTION('center_axis',(1.,0.,0.));
#67982=DIRECTION('ref_axis',(0.,1.,4.63459159752748E-15));
#67983=DIRECTION('center_axis',(1.,0.,0.));
#67984=DIRECTION('ref_axis',(0.,0.,-1.));
#67985=DIRECTION('center_axis',(0.,-1.,-1.22464679914735E-16));
#67986=DIRECTION('ref_axis',(0.,-1.22464679914735E-16,1.));
#67987=DIRECTION('center_axis',(-1.,0.,0.));
#67988=DIRECTION('ref_axis',(0.,1.,0.));
#67989=DIRECTION('center_axis',(1.,0.,0.));
#67990=DIRECTION('ref_axis',(0.,1.,0.));
#67991=DIRECTION('center_axis',(1.,0.,0.));
#67992=DIRECTION('ref_axis',(0.,0.966096391796101,-0.258181644890869));
#67993=DIRECTION('center_axis',(-1.,0.,0.));
#67994=DIRECTION('ref_axis',(0.,0.,1.));
#67995=DIRECTION('center_axis',(1.,0.,0.));
#67996=DIRECTION('ref_axis',(0.,0.,-1.));
#67997=DIRECTION('center_axis',(-1.,0.,0.));
#67998=DIRECTION('ref_axis',(0.,1.,0.));
#67999=DIRECTION('',(0.534234448563085,0.845336355522757,1.03523846199383E-16));
#68000=DIRECTION('center_axis',(1.,0.,0.));
#68001=DIRECTION('ref_axis',(0.,1.,0.));
#68002=DIRECTION('center_axis',(0.,1.4792020664489E-16,1.));
#68003=DIRECTION('ref_axis',(0.,-1.,1.4792020664489E-16));
#68004=DIRECTION('',(1.,0.,0.));
#68005=DIRECTION('',(0.,-1.,1.4792020664489E-16));
#68006=DIRECTION('',(1.,0.,0.));
#68007=DIRECTION('center_axis',(0.,0.866025403784439,0.5));
#68008=DIRECTION('ref_axis',(0.,-0.5,0.866025403784439));
#68009=DIRECTION('',(1.,0.,0.));
#68010=DIRECTION('',(0.,-0.5,0.866025403784439));
#68011=DIRECTION('center_axis',(0.,0.866025403784439,-0.5));
#68012=DIRECTION('ref_axis',(0.,0.5,0.866025403784439));
#68013=DIRECTION('',(1.,0.,0.));
#68014=DIRECTION('',(0.,0.5,0.866025403784439));
#68015=DIRECTION('center_axis',(1.,0.,0.));
#68016=DIRECTION('ref_axis',(0.,1.,0.));
#68017=DIRECTION('center_axis',(1.,0.,0.));
#68018=DIRECTION('ref_axis',(0.,1.,0.));
#68019=DIRECTION('',(-1.,0.,0.));
#68020=DIRECTION('center_axis',(-1.,0.,0.));
#68021=DIRECTION('ref_axis',(0.,0.,1.));
#68022=DIRECTION('center_axis',(1.,0.,0.));
#68023=DIRECTION('ref_axis',(0.,0.,-1.));
#68024=DIRECTION('center_axis',(1.,0.,0.));
#68025=DIRECTION('ref_axis',(0.,1.,0.));
#68026=DIRECTION('',(-0.707106781186548,0.707106781186547,8.65956056235493E-17));
#68027=DIRECTION('center_axis',(0.,-2.95840413289779E-16,-1.));
#68028=DIRECTION('ref_axis',(0.,1.,-2.95840413289779E-16));
#68029=DIRECTION('',(1.,0.,0.));
#68030=DIRECTION('',(0.,1.,-2.95840413289779E-16));
#68031=DIRECTION('center_axis',(0.,-0.866025403784439,-0.5));
#68032=DIRECTION('ref_axis',(0.,0.5,-0.866025403784439));
#68033=DIRECTION('',(1.,0.,0.));
#68034=DIRECTION('',(0.,0.5,-0.866025403784439));
#68035=DIRECTION('center_axis',(0.,-0.866025403784439,0.5));
#68036=DIRECTION('ref_axis',(0.,-0.5,-0.866025403784439));
#68037=DIRECTION('',(0.,-0.5,-0.866025403784439));
#68038=DIRECTION('center_axis',(1.,0.,0.));
#68039=DIRECTION('ref_axis',(0.,0.,-1.));
#68040=DIRECTION('center_axis',(1.,0.,0.));
#68041=DIRECTION('ref_axis',(0.,0.,-1.));
#90630=CARTESIAN_POINT('',(0.,0.,0.));
#90631=CARTESIAN_POINT('Origin',(-14.6,0.,0.));
#90632=CARTESIAN_POINT('',(-28.862836477965,-3.93726360443606,0.0027323502637925));
#90633=CARTESIAN_POINT('',(-29.046163522035,-3.93671054810784,0.00404045690675457));
#90634=CARTESIAN_POINT('',(-14.6,-3.933,-4.81653586104654E-16));
#90635=CARTESIAN_POINT('',(-29.267,1.75074643530109,3.52538993219839));
#90636=CARTESIAN_POINT('Ctrl Pts',(-28.862836477965,-3.93726360443606,0.0027323502637925));
#90637=CARTESIAN_POINT('Ctrl Pts',(-28.8704880036245,-3.93837525323034,
0.153518646252777));
#90638=CARTESIAN_POINT('Ctrl Pts',(-28.878139529284,-3.93046040114638,0.304180408115829));
#90639=CARTESIAN_POINT('Ctrl Pts',(-28.8857910549435,-3.91312829588934,
0.453742202611319));
#90640=CARTESIAN_POINT('Ctrl Pts',(-28.9517303860892,-3.76376364903901,
1.74263609552425));
#90641=CARTESIAN_POINT('Ctrl Pts',(-29.0176697172349,-2.91501250501241,
2.94983925441235));
#90642=CARTESIAN_POINT('Ctrl Pts',(-29.0836090483806,-1.75273691390075,
3.52758749070468));
#90643=CARTESIAN_POINT('Ctrl Pts',(-29.1447393655871,-0.675227113126593,
4.06320003539346));
#90644=CARTESIAN_POINT('Ctrl Pts',(-29.2058696827935,0.671743512076998,
4.0578230529153));
#90645=CARTESIAN_POINT('Ctrl Pts',(-29.267,1.75279839527107,3.52791786994589));
#90646=CARTESIAN_POINT('',(-29.267,-1.74869447533113,3.52286199445087));
#90647=CARTESIAN_POINT('Origin',(-29.267,0.,0.));
#90648=CARTESIAN_POINT('Ctrl Pts',(-29.267,-1.74869447533113,3.52286199445087));
#90649=CARTESIAN_POINT('Ctrl Pts',(-29.2010606688543,-2.91633732258385,
2.94326205571725));
#90650=CARTESIAN_POINT('Ctrl Pts',(-29.1351213377086,-3.76336534893867,
1.7427628349399));
#90651=CARTESIAN_POINT('Ctrl Pts',(-29.0691820065629,-3.91257791995379,
0.455813760205835));
#90652=CARTESIAN_POINT('Ctrl Pts',(-29.0615091783869,-3.92994058346889,
0.306061875403748));
#90653=CARTESIAN_POINT('Ctrl Pts',(-29.053836350211,-3.9378547559674,0.15513945093785));
#90654=CARTESIAN_POINT('Ctrl Pts',(-29.046163522035,-3.93671054810784,0.00404045690675457));
#90655=CARTESIAN_POINT('Origin',(-14.6,0.,0.));
#90656=CARTESIAN_POINT('',(-27.612836477965,-3.92708773793745,0.00134795691750567));
#90657=CARTESIAN_POINT('',(-27.796163522035,-3.92707419464339,0.00136457270431441));
#90658=CARTESIAN_POINT('',(-14.6,-3.933,-4.81653586104654E-16));
#90659=CARTESIAN_POINT('Ctrl Pts',(-27.612836477965,-3.92708773793745,0.00134795691750567));
#90660=CARTESIAN_POINT('Ctrl Pts',(-27.641518683417,-3.92884446881095,0.570375667339846));
#90661=CARTESIAN_POINT('Ctrl Pts',(-27.6702008888689,-3.81320567258203,
1.13872220665575));
#90662=CARTESIAN_POINT('Ctrl Pts',(-27.6988830943208,-3.57659994969859,
1.65121917528487));
#90663=CARTESIAN_POINT('Ctrl Pts',(-27.7648224254665,-3.03265213026327,
2.82943078046378));
#90664=CARTESIAN_POINT('Ctrl Pts',(-27.8307617566123,-1.84936613535815,
3.71246449188963));
#90665=CARTESIAN_POINT('Ctrl Pts',(-27.896701087758,-0.56506653815142,3.89861757445132));
#90666=CARTESIAN_POINT('Ctrl Pts',(-27.9626404189037,0.719233059055312,
4.08477065701301));
#90667=CARTESIAN_POINT('Ctrl Pts',(-28.0285797500494,2.10454625856366,3.57404311071053));
#90668=CARTESIAN_POINT('Ctrl Pts',(-28.0945190811951,2.960621034551,2.59873220565746));
#90669=CARTESIAN_POINT('Ctrl Pts',(-28.1604584123408,3.81669581053835,1.62342130060439));
#90670=CARTESIAN_POINT('Ctrl Pts',(-28.2263977434865,4.1435321630047,0.183527036800713));
#90671=CARTESIAN_POINT('Ctrl Pts',(-28.2923370746322,3.79245785029125,-1.06577113364283));
#90672=CARTESIAN_POINT('Ctrl Pts',(-28.3582764057779,3.4413835375778,-2.31506930408637));
#90673=CARTESIAN_POINT('Ctrl Pts',(-28.4242157369236,2.41239855968456,-3.37377138116979));
#90674=CARTESIAN_POINT('Ctrl Pts',(-28.4901550680693,1.17359560009141,-3.76043033403215));
#90675=CARTESIAN_POINT('Ctrl Pts',(-28.556094399215,-0.0652073595017287,
-4.14708928689451));
#90676=CARTESIAN_POINT('Ctrl Pts',(-28.6220337303607,-1.51382830079477,
-3.86170511553583));
#90677=CARTESIAN_POINT('Ctrl Pts',(-28.6879730615064,-2.51314969660425,
-3.0337207163876));
#90678=CARTESIAN_POINT('Ctrl Pts',(-28.7462608669926,-3.39651096407671,
-2.30181469361449));
#90679=CARTESIAN_POINT('Ctrl Pts',(-28.8045486724788,-3.92879528431619,
-1.14592775776201));
#90680=CARTESIAN_POINT('Ctrl Pts',(-28.862836477965,-3.93726360443606,0.0027323502637925));
#90681=CARTESIAN_POINT('Ctrl Pts',(-29.046163522035,-3.93671054810784,0.00404045690675457));
#90682=CARTESIAN_POINT('Ctrl Pts',(-28.9878970190653,-3.9280215759169,-1.14338651298282));
#90683=CARTESIAN_POINT('Ctrl Pts',(-28.9296305160955,-3.3969634616774,-2.30099571067004));
#90684=CARTESIAN_POINT('Ctrl Pts',(-28.8713640131258,-2.51437175851888,
-3.0335120984736));
#90685=CARTESIAN_POINT('Ctrl Pts',(-28.8054246819801,-1.51555591039341,
-3.86248995372817));
#90686=CARTESIAN_POINT('Ctrl Pts',(-28.7394853508344,-0.0665270984670233,
-4.14704673554652));
#90687=CARTESIAN_POINT('Ctrl Pts',(-28.6735460196887,1.17251990448456,-3.7604723075278));
#90688=CARTESIAN_POINT('Ctrl Pts',(-28.607606688543,2.41156690743614,-3.37389787950909));
#90689=CARTESIAN_POINT('Ctrl Pts',(-28.5416673573973,3.44063210141293,-2.31619224165332));
#90690=CARTESIAN_POINT('Ctrl Pts',(-28.4757280262516,3.79204558724253,-1.06716650818582));
#90691=CARTESIAN_POINT('Ctrl Pts',(-28.4097886951059,4.14345907307213,0.18185922528169));
#90692=CARTESIAN_POINT('Ctrl Pts',(-28.3438493639602,3.81722085075455,1.62220505436093));
#90693=CARTESIAN_POINT('Ctrl Pts',(-28.2779100328145,2.9614918507157,2.59787371676636));
#90694=CARTESIAN_POINT('Ctrl Pts',(-28.2119707016688,2.10576285067685,3.57354237917179));
#90695=CARTESIAN_POINT('Ctrl Pts',(-28.146031370523,0.720543072916747,4.08453387490342));
#90696=CARTESIAN_POINT('Ctrl Pts',(-28.0800920393773,-0.563833091052422,
3.89875014065244));
#90697=CARTESIAN_POINT('Ctrl Pts',(-28.0141527082316,-1.84820925502159,
3.71296640640145));
#90698=CARTESIAN_POINT('Ctrl Pts',(-27.9482133770859,-3.03174180519982,
2.83040744216786));
#90699=CARTESIAN_POINT('Ctrl Pts',(-27.8822740459403,-3.57605921681971,
1.65239327736364));
#90700=CARTESIAN_POINT('Ctrl Pts',(-27.8535705379718,-3.81300155290831,
1.13960161904887));
#90701=CARTESIAN_POINT('Ctrl Pts',(-27.8248670300034,-3.92882052327039,
0.570824853129742));
#90702=CARTESIAN_POINT('Ctrl Pts',(-27.796163522035,-3.92707419464339,0.00136457270431441));
#90703=CARTESIAN_POINT('Origin',(-14.6,0.,0.));
#90704=CARTESIAN_POINT('',(-26.362836477965,-3.9324910341208,-0.00353437058449479));
#90705=CARTESIAN_POINT('',(-26.546163522035,-3.93250329400039,-0.00353456554338567));
#90706=CARTESIAN_POINT('',(-14.6,-3.933,-4.81653586104654E-16));
#90707=CARTESIAN_POINT('Ctrl Pts',(-26.362836477965,-3.9324910341208,-0.0035343705844948));
#90708=CARTESIAN_POINT('Ctrl Pts',(-26.4125493632094,-3.92366140675108,
0.979300462816973));
#90709=CARTESIAN_POINT('Ctrl Pts',(-26.4622622484538,-3.5499695151475,1.96812479991632));
#90710=CARTESIAN_POINT('Ctrl Pts',(-26.5119751336982,-2.88332081962348,
2.68422145640243));
#90711=CARTESIAN_POINT('Ctrl Pts',(-26.5779144648439,-1.99907584217135,
3.63405436857873));
#90712=CARTESIAN_POINT('Ctrl Pts',(-26.6438537959896,-0.599418628171099,
4.10406506139591));
#90713=CARTESIAN_POINT('Ctrl Pts',(-26.7097931271353,0.678883795085354,
3.8804250807624));
#90714=CARTESIAN_POINT('Ctrl Pts',(-26.775732458281,1.95718621834181,3.65678510012889));
#90715=CARTESIAN_POINT('Ctrl Pts',(-26.8416717894267,3.11413385085448,2.7394944460447));
#90716=CARTESIAN_POINT('Ctrl Pts',(-26.9076111205724,3.62337886308066,1.54586884290443));
#90717=CARTESIAN_POINT('Ctrl Pts',(-26.9735504517181,4.13262387530683,0.352243239764167));
#90718=CARTESIAN_POINT('Ctrl Pts',(-27.0394897828638,3.99416626724652,-1.11771731243217));
#90719=CARTESIAN_POINT('Ctrl Pts',(-27.1054291140095,3.27099705696224,-2.19525935283343));
#90720=CARTESIAN_POINT('Ctrl Pts',(-27.1713684451552,2.54782784667795,-3.27280139323469));
#90721=CARTESIAN_POINT('Ctrl Pts',(-27.2373077763009,1.23994703416969,-3.95792492184086));
#90722=CARTESIAN_POINT('Ctrl Pts',(-27.3032471074466,-0.0576322518721723,
-3.93894051569577));
#90723=CARTESIAN_POINT('Ctrl Pts',(-27.3691864385923,-1.35521153791403,
-3.91995610955068));
#90724=CARTESIAN_POINT('Ctrl Pts',(-27.4351257697381,-2.64248929748948,
-3.19686376865435));
#90725=CARTESIAN_POINT('Ctrl Pts',(-27.5010651008838,-3.33382335529445,
-2.0986228487402));
#90726=CARTESIAN_POINT('Ctrl Pts',(-27.5383222265775,-3.72444181381511,
-1.47809335163534));
#90727=CARTESIAN_POINT('Ctrl Pts',(-27.5755793522713,-3.92480580940606,
-0.737798025631152));
#90728=CARTESIAN_POINT('Ctrl Pts',(-27.612836477965,-3.92708773793745,0.00134795691750567));
#90729=CARTESIAN_POINT('Ctrl Pts',(-27.796163522035,-3.92707419464339,0.00136457270431441));
#90730=CARTESIAN_POINT('Ctrl Pts',(-27.7589276988577,-3.92480875781817,
-0.737371693668906));
#90731=CARTESIAN_POINT('Ctrl Pts',(-27.7216918756804,-3.72469557009487,
-1.4772582297981));
#90732=CARTESIAN_POINT('Ctrl Pts',(-27.6844560525031,-3.33450232419475,
-2.0975649274865));
#90733=CARTESIAN_POINT('Ctrl Pts',(-27.6185167213574,-2.64352574688834,
-3.19603960215757));
#90734=CARTESIAN_POINT('Ctrl Pts',(-27.5525773902117,-1.35647031921396,
-3.91951958612487));
#90735=CARTESIAN_POINT('Ctrl Pts',(-27.486638059066,-0.0588948626118422,
-3.93891465672187));
#90736=CARTESIAN_POINT('Ctrl Pts',(-27.4206987279203,1.23868059399027,-3.95830972731887));
#90737=CARTESIAN_POINT('Ctrl Pts',(-27.3547593967746,2.54677607952012,-3.27361988454557));
#90738=CARTESIAN_POINT('Ctrl Pts',(-27.2888200656289,3.2702900962885,-2.19631348578418));
#90739=CARTESIAN_POINT('Ctrl Pts',(-27.2228807344832,3.99380411305689,-1.11900708702278));
#90740=CARTESIAN_POINT('Ctrl Pts',(-27.1569414033375,4.1327366610638,0.350915867726706));
#90741=CARTESIAN_POINT('Ctrl Pts',(-27.0910020721918,3.62387579505931,1.54470660957893));
#90742=CARTESIAN_POINT('Ctrl Pts',(-27.0250627410461,3.11501492905483,2.73849735143115));
#90743=CARTESIAN_POINT('Ctrl Pts',(-26.9591234099004,1.95836064903894,3.65615588038611));
#90744=CARTESIAN_POINT('Ctrl Pts',(-26.8931840787547,0.680129861679127,
3.8802055933119));
#90745=CARTESIAN_POINT('Ctrl Pts',(-26.827244747609,-0.598100925680689,
4.10425530623768));
#90746=CARTESIAN_POINT('Ctrl Pts',(-26.7613054164633,-1.99790822038444,
3.6346962031343));
#90747=CARTESIAN_POINT('Ctrl Pts',(-26.6953660853176,-2.88245804158793,
2.68514790245118));
#90748=CARTESIAN_POINT('Ctrl Pts',(-26.6456318975567,-3.54962232923244,
1.96895905652796));
#90749=CARTESIAN_POINT('Ctrl Pts',(-26.5958977097959,-3.92366673042445,
0.979713755669241));
#90750=CARTESIAN_POINT('Ctrl Pts',(-26.546163522035,-3.93250329400039,-0.00353456554338567));
#90751=CARTESIAN_POINT('Origin',(-14.6,0.,0.));
#90752=CARTESIAN_POINT('',(-25.112836477965,-3.93848364963218,0.00166216559900585));
#90753=CARTESIAN_POINT('',(-25.296163522035,-3.93847615505153,0.0016688492094424));
#90754=CARTESIAN_POINT('',(-14.6,-3.933,-4.81653586104654E-16));
#90755=CARTESIAN_POINT('Ctrl Pts',(-25.112836477965,-3.93848364963218,0.00166216559900585));
#90756=CARTESIAN_POINT('Ctrl Pts',(-25.1176407118562,-3.93898935420615,
0.0962682400339248));
#90757=CARTESIAN_POINT('Ctrl Pts',(-25.1224449457473,-3.93587384866819,
0.190840450324815));
#90758=CARTESIAN_POINT('Ctrl Pts',(-25.1272491796384,-3.92903008168484,
0.2851420889527));
#90759=CARTESIAN_POINT('Ctrl Pts',(-25.1931885107842,-3.83509764050396,
1.57945604575908));
#90760=CARTESIAN_POINT('Ctrl Pts',(-25.2591278419299,-3.0388256093705,2.82279900881076));
#90761=CARTESIAN_POINT('Ctrl Pts',(-25.3250671730756,-1.90247401912017,
3.44951822876883));
#90762=CARTESIAN_POINT('Ctrl Pts',(-25.3910065042213,-0.76612242886986,
4.0762374487269));
#90763=CARTESIAN_POINT('Ctrl Pts',(-25.456945835367,0.710308720497307,4.08633292559138));
#90764=CARTESIAN_POINT('Ctrl Pts',(-25.5228851665127,1.85512436849494,3.47521178397906));
#90765=CARTESIAN_POINT('Ctrl Pts',(-25.5888244976584,2.99994001649258,2.86409064236673));
#90766=CARTESIAN_POINT('Ctrl Pts',(-25.6547638288041,3.81314016312069,1.63175288227759));
#90767=CARTESIAN_POINT('Ctrl Pts',(-25.7207031599498,3.92476341178622,0.338844461100057));
#90768=CARTESIAN_POINT('Ctrl Pts',(-25.7866424910955,4.03638666045175,-0.954063960077469));
#90769=CARTESIAN_POINT('Ctrl Pts',(-25.8525818222412,3.44643301115472,-2.3075430423434));
#90770=CARTESIAN_POINT('Ctrl Pts',(-25.9185211533869,2.42329897262029,-3.10583411496569));
#90771=CARTESIAN_POINT('Ctrl Pts',(-25.9844604845326,1.40016493408586,-3.90412518758798));
#90772=CARTESIAN_POINT('Ctrl Pts',(-26.0503998156783,-0.0561494936859615,
-4.14722825056663));
#90773=CARTESIAN_POINT('Ctrl Pts',(-26.116339146824,-1.28310126714286,-3.72454484960586));
#90774=CARTESIAN_POINT('Ctrl Pts',(-26.1822784779697,-2.51005304059976,
-3.30186144864509));
#90775=CARTESIAN_POINT('Ctrl Pts',(-26.2482178091154,-3.50764215974172,
-2.21339158374489));
#90776=CARTESIAN_POINT('Ctrl Pts',(-26.3141571402611,-3.82202034886068,
-0.95432908552708));
#90777=CARTESIAN_POINT('Ctrl Pts',(-26.3303835861624,-3.8993829879663,-0.644497166417136));
#90778=CARTESIAN_POINT('Ctrl Pts',(-26.3466100320637,-3.93537305294025,
-0.32433482655703));
#90779=CARTESIAN_POINT('Ctrl Pts',(-26.362836477965,-3.9324910341208,-0.0035343705844948));
#90780=CARTESIAN_POINT('Ctrl Pts',(-26.546163522035,-3.93250329400039,-0.00353456554338567));
#90781=CARTESIAN_POINT('Ctrl Pts',(-26.5299583786502,-3.93538255645996,
-0.32391136760875));
#90782=CARTESIAN_POINT('Ctrl Pts',(-26.5137532352653,-3.89948824923301,
-0.643651479317923));
#90783=CARTESIAN_POINT('Ctrl Pts',(-26.4975480918805,-3.82232660328557,
-0.953101486990109));
#90784=CARTESIAN_POINT('Ctrl Pts',(-26.4316087607348,-3.50835299607651,
-2.21226507748542));
#90785=CARTESIAN_POINT('Ctrl Pts',(-26.3656694295891,-2.51111343395517,
-3.30105476021319));
#90786=CARTESIAN_POINT('Ctrl Pts',(-26.2997300984434,-1.28429752491345,
-3.72413212926964));
#90787=CARTESIAN_POINT('Ctrl Pts',(-26.2337907672977,-0.0574816158717277,
-4.14720949832609));
#90788=CARTESIAN_POINT('Ctrl Pts',(-26.167851436152,1.39891064009036,-3.90457455371123));
#90789=CARTESIAN_POINT('Ctrl Pts',(-26.1019121050063,2.42230098071725,-3.10661229877343));
#90790=CARTESIAN_POINT('Ctrl Pts',(-26.0359727738606,3.44569132134414,-2.30865004383564));
#90791=CARTESIAN_POINT('Ctrl Pts',(-25.9700334427149,4.03607974663582,-0.955360478574905));
#90792=CARTESIAN_POINT('Ctrl Pts',(-25.9040941115692,3.92487185002737,0.33758369389623));
#90793=CARTESIAN_POINT('Ctrl Pts',(-25.8381547804235,3.81366395341891,1.63052786636736));
#90794=CARTESIAN_POINT('Ctrl Pts',(-25.7722154492778,3.00085973491032,2.86312664604889));
#90795=CARTESIAN_POINT('Ctrl Pts',(-25.7062761181321,1.85624051708109,3.47461545772335));
#90796=CARTESIAN_POINT('Ctrl Pts',(-25.6403367869864,0.71162129925185,4.08610426939782));
#90797=CARTESIAN_POINT('Ctrl Pts',(-25.5743974558406,-0.764812917898037,
4.07648311306521));
#90798=CARTESIAN_POINT('Ctrl Pts',(-25.5084581246949,-1.90136570512696,
3.45012900550375));
#90799=CARTESIAN_POINT('Ctrl Pts',(-25.4425187935492,-3.03791849235588,
2.82377489794229));
#90800=CARTESIAN_POINT('Ctrl Pts',(-25.3765794624036,-3.83458984966384,
1.58068783915199));
#90801=CARTESIAN_POINT('Ctrl Pts',(-25.3106401312579,-3.92893806068268,
0.286404192041365));
#90802=CARTESIAN_POINT('Ctrl Pts',(-25.3058145948502,-3.93584260034595,
0.191686627389066));
#90803=CARTESIAN_POINT('Ctrl Pts',(-25.3009890584426,-3.93898583025972,
0.0966948780857186));
#90804=CARTESIAN_POINT('Ctrl Pts',(-25.296163522035,-3.93847615505153,0.0016688492094424));
#90805=CARTESIAN_POINT('Origin',(-14.6,0.,0.));
#90806=CARTESIAN_POINT('',(-23.862836477965,-3.92784938859273,0.00213917922607304));
#90807=CARTESIAN_POINT('',(-24.046163522035,-3.92784218437645,0.00213368844150495));
#90808=CARTESIAN_POINT('',(-14.6,-3.933,-4.81653586104654E-16));
#90809=CARTESIAN_POINT('Ctrl Pts',(-23.862836477965,-3.92784938859273,0.00213917922607304));
#90810=CARTESIAN_POINT('Ctrl Pts',(-23.8886713916486,-3.93039759682621,
0.514429414290928));
#90811=CARTESIAN_POINT('Ctrl Pts',(-23.9145063053322,-3.83728702899802,
1.02582969131807));
#90812=CARTESIAN_POINT('Ctrl Pts',(-23.9403412190158,-3.6441795653241,1.4961746851344));
#90813=CARTESIAN_POINT('Ctrl Pts',(-24.0062805501615,-3.15130480097032,
2.69665225126127));
#90814=CARTESIAN_POINT('Ctrl Pts',(-24.0722198813072,-2.00700932293093,
3.62967889640143));
#90815=CARTESIAN_POINT('Ctrl Pts',(-24.1381592124529,-0.731884709970319,
3.8707787542536));
#90816=CARTESIAN_POINT('Ctrl Pts',(-24.2040985435986,0.543239902990295,
4.11187861210578));
#90817=CARTESIAN_POINT('Ctrl Pts',(-24.2700378747443,1.94919365087213,3.66105168266996));
#90818=CARTESIAN_POINT('Ctrl Pts',(-24.33597720589,2.84634481683359,2.72339945215828));
#90819=CARTESIAN_POINT('Ctrl Pts',(-24.4019165370357,3.74349598279505,1.7857472216466));
#90820=CARTESIAN_POINT('Ctrl Pts',(-24.4678558681814,4.13184456683614,0.361269690059079));
#90821=CARTESIAN_POINT('Ctrl Pts',(-24.5337951993271,3.83471329770221,-0.901974122230396));
#90822=CARTESIAN_POINT('Ctrl Pts',(-24.5997345304728,3.53758202856828,-2.16521793451989));
#90823=CARTESIAN_POINT('Ctrl Pts',(-24.6656738616185,2.55497090625931,-3.26722802751132));
#90824=CARTESIAN_POINT('Ctrl Pts',(-24.7316131927642,1.33391401022604,-3.70665034875255));
#90825=CARTESIAN_POINT('Ctrl Pts',(-24.7975525239099,0.112857114192773,
-4.14607266999378));
#90826=CARTESIAN_POINT('Ctrl Pts',(-24.8634918550556,-1.3466455555648,-3.9229072194848));
#90827=CARTESIAN_POINT('Ctrl Pts',(-24.9294311862013,-2.38060046482942,
-3.13868201894977));
#90828=CARTESIAN_POINT('Ctrl Pts',(-24.9905662834559,-3.33922307801683,
-2.41159420851614));
#90829=CARTESIAN_POINT('Ctrl Pts',(-25.0517013807105,-3.93204843040415,
-1.20222417559595));
#90830=CARTESIAN_POINT('Ctrl Pts',(-25.112836477965,-3.93848364963218,0.00166216559900585));
#90831=CARTESIAN_POINT('Ctrl Pts',(-25.296163522035,-3.93847615505153,0.0016688492094424));
#90832=CARTESIAN_POINT('Ctrl Pts',(-25.2350497272969,-3.9320212900531,-1.20180382884279));
#90833=CARTESIAN_POINT('Ctrl Pts',(-25.1739359325588,-3.33966345243659,
-2.41077473447204));
#90834=CARTESIAN_POINT('Ctrl Pts',(-25.1128221378207,-2.3816084582775,-3.13791694536259));
#90835=CARTESIAN_POINT('Ctrl Pts',(-25.046882806675,-1.34790558012376,-3.92247420022496));
#90836=CARTESIAN_POINT('Ctrl Pts',(-24.9809434755293,0.111525240913435,
-4.14610847451873));
#90837=CARTESIAN_POINT('Ctrl Pts',(-24.9150041443836,1.33272316167415,-3.70707844764346));
#90838=CARTESIAN_POINT('Ctrl Pts',(-24.8490648132379,2.55392108243488,-3.26804842076819));
#90839=CARTESIAN_POINT('Ctrl Pts',(-24.7831254820922,3.53688610291912,-2.16635409272388));
#90840=CARTESIAN_POINT('Ctrl Pts',(-24.7171861509465,3.83442313744424,-0.903205865383198));
#90841=CARTESIAN_POINT('Ctrl Pts',(-24.6512468198008,4.13196017196935,0.359942361957476));
#90842=CARTESIAN_POINT('Ctrl Pts',(-24.5853074886551,3.74406922053537,1.78454448859452));
#90843=CARTESIAN_POINT('Ctrl Pts',(-24.5193681575094,2.84721935774838,2.72248481292816));
#90844=CARTESIAN_POINT('Ctrl Pts',(-24.4534288263637,1.9503694949614,3.66042513726181));
#90845=CARTESIAN_POINT('Ctrl Pts',(-24.387489495218,0.544560720821429,4.11170365929207));
#90846=CARTESIAN_POINT('Ctrl Pts',(-24.3215501640723,-0.73064120346497,
3.87101344158701));
#90847=CARTESIAN_POINT('Ctrl Pts',(-24.2556108329266,-2.00584312775137,
3.63032322388195));
#90848=CARTESIAN_POINT('Ctrl Pts',(-24.1896715017809,-3.1504382021842,2.69766426644156));
#90849=CARTESIAN_POINT('Ctrl Pts',(-24.1237321706352,-3.64369854781322,
1.49734515859372));
#90850=CARTESIAN_POINT('Ctrl Pts',(-24.0978759544351,-3.83711643540636,
1.02667447051812));
#90851=CARTESIAN_POINT('Ctrl Pts',(-24.072019738235,-3.93038567262406,0.514848595044744));
#90852=CARTESIAN_POINT('Ctrl Pts',(-24.046163522035,-3.92784218437645,0.00213368844150495));
#90853=CARTESIAN_POINT('Origin',(-14.6,0.,0.));
#90854=CARTESIAN_POINT('',(-22.612836477965,-3.93087436129151,-0.00338089423011334));
#90855=CARTESIAN_POINT('',(-22.796163522035,-3.93088572622165,-0.00338294474049346));
#90856=CARTESIAN_POINT('',(-14.6,-3.933,-4.81653586104654E-16));
#90857=CARTESIAN_POINT('Ctrl Pts',(-22.612836477965,-3.93087436129151,-0.00338089423011334));
#90858=CARTESIAN_POINT('Ctrl Pts',(-22.6597020714411,-3.92317635965085,
0.924132377966204));
#90859=CARTESIAN_POINT('Ctrl Pts',(-22.7065676649171,-3.59478909080291,
1.85655093763582));
#90860=CARTESIAN_POINT('Ctrl Pts',(-22.7534332583932,-2.99587824469287,
2.55798689124243));
#90861=CARTESIAN_POINT('Ctrl Pts',(-22.8193725895389,-2.15321782626481,
3.54489891329993));
#90862=CARTESIAN_POINT('Ctrl Pts',(-22.8853119206846,-0.77502475658801,
4.07455420132641));
#90863=CARTESIAN_POINT('Ctrl Pts',(-22.9512512518303,0.511698830953477,
3.90598869675791));
#90864=CARTESIAN_POINT('Ctrl Pts',(-23.017190582976,1.79842241849496,3.7374231921894));
#90865=CARTESIAN_POINT('Ctrl Pts',(-23.0831299141217,2.99367652390115,2.87063689502596));
#90866=CARTESIAN_POINT('Ctrl Pts',(-23.1490692452674,3.55368619247757,1.69996995214067));
#90867=CARTESIAN_POINT('Ctrl Pts',(-23.2150085764131,4.11369586105398,0.529303009255378));
#90868=CARTESIAN_POINT('Ctrl Pts',(-23.2809479075588,4.03846109280059,-0.945244579351747));
#90869=CARTESIAN_POINT('Ctrl Pts',(-23.3468872387045,3.36220957412427,-2.05283466758846));
#90870=CARTESIAN_POINT('Ctrl Pts',(-23.4128265698502,2.68595805544795,-3.16042475582517));
#90871=CARTESIAN_POINT('Ctrl Pts',(-23.4787659009959,1.40868978634868,-3.90105734369146));
#90872=CARTESIAN_POINT('Ctrl Pts',(-23.5447052321416,0.111491660421779,
-3.93778529156826));
#90873=CARTESIAN_POINT('Ctrl Pts',(-23.6106445632873,-1.18570646550513,
-3.97451323944505));
#90874=CARTESIAN_POINT('Ctrl Pts',(-23.676583894433,-2.50283444825967,-3.30733654733236));
#90875=CARTESIAN_POINT('Ctrl Pts',(-23.7425232255787,-3.24067141430286,
-2.23978395771922));
#90876=CARTESIAN_POINT('Ctrl Pts',(-23.7826276430408,-3.68942515794924,
-1.59049659048769));
#90877=CARTESIAN_POINT('Ctrl Pts',(-23.8227320605029,-3.92389371805991,
-0.793106421375654));
#90878=CARTESIAN_POINT('Ctrl Pts',(-23.862836477965,-3.92784938859273,0.00213917922607304));
#90879=CARTESIAN_POINT('Ctrl Pts',(-24.046163522035,-3.92784218437645,0.00213368844150495));
#90880=CARTESIAN_POINT('Ctrl Pts',(-24.0060804070893,-3.92389918935342,
-0.792692993726209));
#90881=CARTESIAN_POINT('Ctrl Pts',(-23.9659972921437,-3.68969742380163,
-1.58965621061758));
#90882=CARTESIAN_POINT('Ctrl Pts',(-23.9259141771981,-3.24139055871715,
-2.23874269998632));
#90883=CARTESIAN_POINT('Ctrl Pts',(-23.8599748460524,-2.50389660716684,
-3.30653219246322));
#90884=CARTESIAN_POINT('Ctrl Pts',(-23.7940355149067,-1.18698308724101,
-3.97413191916171));
#90885=CARTESIAN_POINT('Ctrl Pts',(-23.728096183761,0.110226696404494,-3.93782067989699));
#90886=CARTESIAN_POINT('Ctrl Pts',(-23.6621568526153,1.40743648004999,-3.90150944063227));
#90887=CARTESIAN_POINT('Ctrl Pts',(-23.5962175214696,2.68494252741516,-3.16128723540433));
#90888=CARTESIAN_POINT('Ctrl Pts',(-23.5302781903239,3.36154976881573,-2.05391450238099));
#90889=CARTESIAN_POINT('Ctrl Pts',(-23.4643388591782,4.03815701021631,-0.946541769357638));
#90890=CARTESIAN_POINT('Ctrl Pts',(-23.3983995280325,4.1138654456523,0.52798149146113));
#90891=CARTESIAN_POINT('Ctrl Pts',(-23.3324601968868,3.55423189619171,1.69882820184466));
#90892=CARTESIAN_POINT('Ctrl Pts',(-23.2665208657411,2.99459834673113,2.8696749122282));
#90893=CARTESIAN_POINT('Ctrl Pts',(-23.2005815345954,1.79962281237397,3.73684507217651));
#90894=CARTESIAN_POINT('Ctrl Pts',(-23.1346422034497,0.512953513280088,
3.90582389830908));
#90895=CARTESIAN_POINT('Ctrl Pts',(-23.068702872304,-0.773715785813794,
4.07480272444165));
#90896=CARTESIAN_POINT('Ctrl Pts',(-23.0027635411583,-2.15207884964439,
3.54559021675848));
#90897=CARTESIAN_POINT('Ctrl Pts',(-22.9368242100126,-2.99505620682083,
2.55894899310702));
#90898=CARTESIAN_POINT('Ctrl Pts',(-22.88993731402,-3.59446464762908,1.8573867595887));
#90899=CARTESIAN_POINT('Ctrl Pts',(-22.8430504180275,-3.92317782141207,
0.92454493291896));
#90900=CARTESIAN_POINT('Ctrl Pts',(-22.796163522035,-3.93088572622165,-0.00338294474049346));
#90901=CARTESIAN_POINT('Origin',(-14.6,0.,0.));
#90902=CARTESIAN_POINT('',(-21.362836477965,-3.9392053084022,0.000704079325613109));
#90903=CARTESIAN_POINT('',(-21.546163522035,-3.9392017186225,0.000711618128540299));
#90904=CARTESIAN_POINT('',(-14.6,-3.933,-4.81653586104654E-16));
#90905=CARTESIAN_POINT('Ctrl Pts',(-21.362836477965,-3.9392053084022,0.000704079325613109));
#90906=CARTESIAN_POINT('Ctrl Pts',(-21.3647934200878,-3.93930094846521,
0.0392218073737966));
#90907=CARTESIAN_POINT('Ctrl Pts',(-21.3667503622106,-3.93878454105988,
0.0777369080014598));
#90908=CARTESIAN_POINT('Ctrl Pts',(-21.3687073043334,-3.93764817090949,
0.116233708220938));
#90909=CARTESIAN_POINT('Ctrl Pts',(-21.4346466354791,-3.89935808211342,
1.41338666341404));
#90910=CARTESIAN_POINT('Ctrl Pts',(-21.5005859666248,-3.1571878645482,2.68976209000154));
#90911=CARTESIAN_POINT('Ctrl Pts',(-21.5665252977705,-2.04878419485562,
3.36467928868465));
#90912=CARTESIAN_POINT('Ctrl Pts',(-21.6324646289162,-0.940380525163057,
4.03959648736776));
#90913=CARTESIAN_POINT('Ctrl Pts',(-21.6984039600619,0.534256596656856,
4.1130554581465));
#90914=CARTESIAN_POINT('Ctrl Pts',(-21.7643432912076,1.70424829180925,3.55163640490676));
#90915=CARTESIAN_POINT('Ctrl Pts',(-21.8302826223533,2.87423998696165,2.99021735166702));
#90916=CARTESIAN_POINT('Ctrl Pts',(-21.896221953499,3.73958625544654,1.7939202744088));
#90917=CARTESIAN_POINT('Ctrl Pts',(-21.9621612846447,3.90660208433412,0.506994622722924));
#90918=CARTESIAN_POINT('Ctrl Pts',(-22.0281006157904,4.07361791322169,-0.77993102896295));
#90919=CARTESIAN_POINT('Ctrl Pts',(-22.0940399469361,3.54230330251196,-2.15748525507647));
#90920=CARTESIAN_POINT('Ctrl Pts',(-22.1599792780818,2.55437721142949,-2.99895656095968));
#90921=CARTESIAN_POINT('Ctrl Pts',(-22.2259186092275,1.56645112034702,-3.84042786684288));
#90922=CARTESIAN_POINT('Ctrl Pts',(-22.2918579403732,0.121913548891806,
-4.14581625249578));
#90923=CARTESIAN_POINT('Ctrl Pts',(-22.357797271519,-1.1220502659885,-3.7761867794628));
#90924=CARTESIAN_POINT('Ctrl Pts',(-22.4237366026647,-2.36601408086881,
-3.40655730642983));
#90925=CARTESIAN_POINT('Ctrl Pts',(-22.4896759338103,-3.40940413917422,
-2.36190997471099));
#90926=CARTESIAN_POINT('Ctrl Pts',(-22.555615264956,-3.77753528473724,-1.1175019308073));
#90927=CARTESIAN_POINT('Ctrl Pts',(-22.5746890026257,-3.88402160749027,
-0.757542068142264));
#90928=CARTESIAN_POINT('Ctrl Pts',(-22.5937627402954,-3.93400735616011,
-0.380867735361056));
#90929=CARTESIAN_POINT('Ctrl Pts',(-22.612836477965,-3.93087436129151,-0.00338089423011334));
#90930=CARTESIAN_POINT('Ctrl Pts',(-22.796163522035,-3.93088572622165,-0.00338294474049346));
#90931=CARTESIAN_POINT('Ctrl Pts',(-22.7771110868818,-3.93401782429389,
-0.380445348674258));
#90932=CARTESIAN_POINT('Ctrl Pts',(-22.7580586517286,-3.88414573503703,
-0.756696364450129));
#90933=CARTESIAN_POINT('Ctrl Pts',(-22.7390062165754,-3.77789385546023,
-1.11628833560879));
#90934=CARTESIAN_POINT('Ctrl Pts',(-22.6730668854297,-3.41016249640089,
-2.36081450105337));
#90935=CARTESIAN_POINT('Ctrl Pts',(-22.6071275542841,-2.36710812775992,
-3.40579689232276));
#90936=CARTESIAN_POINT('Ctrl Pts',(-22.5411882231384,-1.12326318534757,
-3.77582592922345));
#90937=CARTESIAN_POINT('Ctrl Pts',(-22.4752488919926,0.120581757064785,
-4.14585496612414));
#90938=CARTESIAN_POINT('Ctrl Pts',(-22.4093095608469,1.56521727324854,-3.84093064865612));
#90939=CARTESIAN_POINT('Ctrl Pts',(-22.3433702297012,2.55341356678447,-2.99977678974731));
#90940=CARTESIAN_POINT('Ctrl Pts',(-22.2774308985555,3.54160986032041,-2.1586229308385));
#90941=CARTESIAN_POINT('Ctrl Pts',(-22.2114915674098,4.07336693120854,-0.781239530488878));
#90942=CARTESIAN_POINT('Ctrl Pts',(-22.1455522362641,3.90676452515084,0.505739632982661));
#90943=CARTESIAN_POINT('Ctrl Pts',(-22.0796129051184,3.74016211909313,1.79271879645421));
#90944=CARTESIAN_POINT('Ctrl Pts',(-22.0136735739727,2.87520023608961,2.98929372304766));
#90945=CARTESIAN_POINT('Ctrl Pts',(-21.947734242827,1.70538901479264,3.55108855698822));
#90946=CARTESIAN_POINT('Ctrl Pts',(-21.8817949116813,0.535577793495685,
4.11288339092877));
#90947=CARTESIAN_POINT('Ctrl Pts',(-21.8158555805356,-0.939082766094701,
4.03989813221641));
#90948=CARTESIAN_POINT('Ctrl Pts',(-21.7499162493899,-2.04770312228556,
3.36533706399953));
#90949=CARTESIAN_POINT('Ctrl Pts',(-21.6839769182442,-3.15632347847641,
2.69077599578264));
#90950=CARTESIAN_POINT('Ctrl Pts',(-21.6180375870985,-3.89890363126774,
1.41463911806121));
#90951=CARTESIAN_POINT('Ctrl Pts',(-21.5520982559528,-3.93761040601042,
0.117498603504866));
#90952=CARTESIAN_POINT('Ctrl Pts',(-21.5501200113135,-3.93877164723486,
0.0785831152110228));
#90953=CARTESIAN_POINT('Ctrl Pts',(-21.5481417666742,-3.93929936097659,
0.0396487224073827));
#90954=CARTESIAN_POINT('Ctrl Pts',(-21.546163522035,-3.9392017186225,0.000711618128540299));
#90955=CARTESIAN_POINT('Origin',(-14.6,0.,0.));
#90956=CARTESIAN_POINT('',(-20.112836477965,-3.9289412454305,0.00279384190022436));
#90957=CARTESIAN_POINT('',(-20.296163522035,-3.92893175430004,0.00278958524027692));
#90958=CARTESIAN_POINT('',(-14.6,-3.933,-4.81653586104654E-16));
#90959=CARTESIAN_POINT('Ctrl Pts',(-20.112836477965,-3.9289412454305,0.00279384190022436));
#90960=CARTESIAN_POINT('Ctrl Pts',(-20.1358240998803,-3.93195496054311,
0.458305859925948));
#90961=CARTESIAN_POINT('Ctrl Pts',(-20.1588117217955,-3.85874422505227,
0.912879494791886));
#90962=CARTESIAN_POINT('Ctrl Pts',(-20.1817993437108,-3.70504127758559,
1.33837682443348));
#90963=CARTESIAN_POINT('Ctrl Pts',(-20.2477386748565,-3.26414880125882,
2.55890365510319));
#90964=CARTESIAN_POINT('Ctrl Pts',(-20.3136780060022,-2.16095618577067,
3.54018695495582));
#90965=CARTESIAN_POINT('Ctrl Pts',(-20.3796173371479,-0.897355465454369,
3.83579673098208));
#90966=CARTESIAN_POINT('Ctrl Pts',(-20.4455566682936,0.366245254861932,
4.13140650700835));
#90967=CARTESIAN_POINT('Ctrl Pts',(-20.5114959994393,1.79025408000638,3.7413427592083));
#90968=CARTESIAN_POINT('Ctrl Pts',(-20.577435330585,2.72682522482214,2.84306306403276));
#90969=CARTESIAN_POINT('Ctrl Pts',(-20.6433746617307,3.66339636963791,1.94478336885722));
#90970=CARTESIAN_POINT('Ctrl Pts',(-20.7093139928764,4.11252983412497,0.538287726306191));
#90971=CARTESIAN_POINT('Ctrl Pts',(-20.7752533240221,3.86989456583263,-0.736545614427758));
#90972=CARTESIAN_POINT('Ctrl Pts',(-20.8411926551678,3.62725929754029,-2.0113789551617));
#90973=CARTESIAN_POINT('Ctrl Pts',(-20.9071319863135,2.69285529646856,-3.15454999407856));
#90974=CARTESIAN_POINT('Ctrl Pts',(-20.9730713174592,1.49178505007331,-3.64597871046602));
#90975=CARTESIAN_POINT('Ctrl Pts',(-21.0390106486049,0.290714803678051,
-4.13740742685348));
#90976=CARTESIAN_POINT('Ctrl Pts',(-21.1049499797506,-1.17702168804074,
-3.97709382071151));
#90977=CARTESIAN_POINT('Ctrl Pts',(-21.1708893108963,-2.24368495388664,
-3.23797177574116));
#90978=CARTESIAN_POINT('Ctrl Pts',(-21.2348716999192,-3.27869187382335,
-2.52078533488684));
#90979=CARTESIAN_POINT('Ctrl Pts',(-21.2988540889421,-3.93607834841387,
-1.25863631278614));
#90980=CARTESIAN_POINT('Ctrl Pts',(-21.362836477965,-3.9392053084022,0.000704079325613109));
#90981=CARTESIAN_POINT('Ctrl Pts',(-21.546163522035,-3.9392017186225,0.000711618128540299));
#90982=CARTESIAN_POINT('Ctrl Pts',(-21.4822024355285,-3.93604472229705,
-1.25821230141494));
#90983=CARTESIAN_POINT('Ctrl Pts',(-21.4182413490221,-3.27915675941927,
-2.51997072647733));
#90984=CARTESIAN_POINT('Ctrl Pts',(-21.3542802625157,-2.24472485856745,
-3.23725067621843));
#90985=CARTESIAN_POINT('Ctrl Pts',(-21.28834093137,-1.17829913968773,-3.97671528999414));
#90986=CARTESIAN_POINT('Ctrl Pts',(-21.2224016002243,0.289385694765753,
-4.13750036615427));
#90987=CARTESIAN_POINT('Ctrl Pts',(-21.1564622690786,1.49061367481441,-3.64645752804053));
#90988=CARTESIAN_POINT('Ctrl Pts',(-21.0905229379329,2.69184165486307,-3.15541468992679));
#90989=CARTESIAN_POINT('Ctrl Pts',(-21.0245836067872,3.6266127805069,-2.0125439375392));
#90990=CARTESIAN_POINT('Ctrl Pts',(-20.9586442756415,3.86965754277835,-0.737788677715975));
#90991=CARTESIAN_POINT('Ctrl Pts',(-20.8927049444958,4.11270230504979,0.536966582107239));
#90992=CARTESIAN_POINT('Ctrl Pts',(-20.8267656133501,3.66402070394882,1.94360634936608));
#90993=CARTESIAN_POINT('Ctrl Pts',(-20.7608262822044,2.72773821890935,2.84218680604363));
#90994=CARTESIAN_POINT('Ctrl Pts',(-20.6948869510587,1.79145573386986,3.74076726272119));
#90995=CARTESIAN_POINT('Ctrl Pts',(-20.628947619913,0.367572364891867,4.13128840881747));
#90996=CARTESIAN_POINT('Ctrl Pts',(-20.5630082887673,-0.89612317853138,
3.83608457678478));
#90997=CARTESIAN_POINT('Ctrl Pts',(-20.4970689576216,-2.15981872195464,
3.54088074475208));
#90998=CARTESIAN_POINT('Ctrl Pts',(-20.4311296264759,-3.26332643982314,
2.55995193459039));
#90999=CARTESIAN_POINT('Ctrl Pts',(-20.3651902953302,-3.70461094353127,
1.33956686597407));
#91000=CARTESIAN_POINT('Ctrl Pts',(-20.3421813708984,-3.85859312112231,
0.913724696611549));
#91001=CARTESIAN_POINT('Ctrl Pts',(-20.3191724464667,-3.93194320050247,
0.458726405663346));
#91002=CARTESIAN_POINT('Ctrl Pts',(-20.296163522035,-3.92893175430004,0.00278958524027692));
#91003=CARTESIAN_POINT('Origin',(-14.6,0.,0.));
#91004=CARTESIAN_POINT('',(-18.862836477965,-3.92942440079457,-0.0029931669997546));
#91005=CARTESIAN_POINT('',(-19.046163522035,-3.92943419637598,-0.00299686489160711));
#91006=CARTESIAN_POINT('',(-14.6,-3.933,-4.81653586104654E-16));
#91007=CARTESIAN_POINT('Ctrl Pts',(-18.862836477965,-3.92942440079457,-0.0029931669997546));
#91008=CARTESIAN_POINT('Ctrl Pts',(-18.9068547796727,-3.92319085932645,
0.868982802255619));
#91009=CARTESIAN_POINT('Ctrl Pts',(-18.9508730813804,-3.63664096818252,
1.74467880622105));
#91010=CARTESIAN_POINT('Ctrl Pts',(-18.9948913830881,-3.10291356106906,
2.42703745857526));
#91011=CARTESIAN_POINT('Ctrl Pts',(-19.0608307142338,-2.30339093357437,
3.44920940506477));
#91012=CARTESIAN_POINT('Ctrl Pts',(-19.1267700453795,-0.949202398378664,
4.03753267723891));
#91013=CARTESIAN_POINT('Ctrl Pts',(-19.1927093765252,0.343570655594563,
3.92435250677204));
#91014=CARTESIAN_POINT('Ctrl Pts',(-19.2586487076709,1.63634370956779,3.81117233630516));
#91015=CARTESIAN_POINT('Ctrl Pts',(-19.3245880388166,2.86770128231855,2.99648872319727));
#91016=CARTESIAN_POINT('Ctrl Pts',(-19.3905273699623,3.47744332491339,1.85093795541854));
#91017=CARTESIAN_POINT('Ctrl Pts',(-19.456466701108,4.08718536750824,0.7053871876398));
#91018=CARTESIAN_POINT('Ctrl Pts',(-19.5224060322537,4.07531187994718,-0.771030734809761));
#91019=CARTESIAN_POINT('Ctrl Pts',(-19.5883453633994,3.44722464678077,-1.90662676668006));
#91020=CARTESIAN_POINT('Ctrl Pts',(-19.6542846945451,2.81913741361437,-3.04222279855036));
#91021=CARTESIAN_POINT('Ctrl Pts',(-19.7202240256909,1.57483643484262,-3.83699693984138));
#91022=CARTESIAN_POINT('Ctrl Pts',(-19.7861633568366,0.280410298071069,
-3.92937061849978));
#91023=CARTESIAN_POINT('Ctrl Pts',(-19.8521026879823,-1.01401583870047,
-4.02174429715819));
#91024=CARTESIAN_POINT('Ctrl Pts',(-19.9180420191279,-2.35856713347181,
-3.411717513184));
#91025=CARTESIAN_POINT('Ctrl Pts',(-19.9839813502736,-3.14154661227478,
-2.37681894045351));
#91026=CARTESIAN_POINT('Ctrl Pts',(-20.0269330595041,-3.6515655391069,-1.70270438990228));
#91027=CARTESIAN_POINT('Ctrl Pts',(-20.0698847687346,-3.92331020557359,
-0.848317239591968));
#91028=CARTESIAN_POINT('Ctrl Pts',(-20.112836477965,-3.9289412454305,0.00279384190022436));
#91029=CARTESIAN_POINT('Ctrl Pts',(-20.296163522035,-3.92893175430004,0.00278958524027692));
#91030=CARTESIAN_POINT('Ctrl Pts',(-20.253233115321,-3.9233129514459,-0.847904378952598));
#91031=CARTESIAN_POINT('Ctrl Pts',(-20.210302708607,-3.6518592668377,-1.70186561511352));
#91032=CARTESIAN_POINT('Ctrl Pts',(-20.167372301893,-3.14230978779631,-2.37580951022315));
#91033=CARTESIAN_POINT('Ctrl Pts',(-20.1014329707473,-2.35966283880543,
-3.41095949073314));
#91034=CARTESIAN_POINT('Ctrl Pts',(-20.0354936396016,-1.01530765127591,
-4.02141812468219));
#91035=CARTESIAN_POINT('Ctrl Pts',(-19.9695543084559,0.279148018845661,
-3.92946027017984));
#91036=CARTESIAN_POINT('Ctrl Pts',(-19.9036149773102,1.57360368896723,-3.83750241567748));
#91037=CARTESIAN_POINT('Ctrl Pts',(-19.8376756461645,2.81815984168083,-3.04312807272373));
#91038=CARTESIAN_POINT('Ctrl Pts',(-19.7717363150188,3.4466117992558,-1.90773392709203));
#91039=CARTESIAN_POINT('Ctrl Pts',(-19.7057969838731,4.07506375683076,-0.772339781460326));
#91040=CARTESIAN_POINT('Ctrl Pts',(-19.6398576527274,4.08741151926708,0.704074166849339));
#91041=CARTESIAN_POINT('Ctrl Pts',(-19.5739183215817,3.47803753300102,1.84982068060216));
#91042=CARTESIAN_POINT('Ctrl Pts',(-19.507978990436,2.86866354673495,2.99556719435499));
#91043=CARTESIAN_POINT('Ctrl Pts',(-19.4420396592903,1.63756781176651,3.81064627355099));
#91044=CARTESIAN_POINT('Ctrl Pts',(-19.3761003281446,0.34483125522266,3.92424171487547));
#91045=CARTESIAN_POINT('Ctrl Pts',(-19.3101609969989,-0.947905301321183,
4.03783715619996));
#91046=CARTESIAN_POINT('Ctrl Pts',(-19.2442216658532,-2.30228267944042,
3.44994895965294));
#91047=CARTESIAN_POINT('Ctrl Pts',(-19.1782823347075,-3.10213357705578,
2.42803395805132));
#91048=CARTESIAN_POINT('Ctrl Pts',(-19.1342427304833,-3.63633852510867,
1.7455166889295));
#91049=CARTESIAN_POINT('Ctrl Pts',(-19.0902031262592,-3.92318885129781,
0.869395435115258));
#91050=CARTESIAN_POINT('Ctrl Pts',(-19.046163522035,-3.92943419637598,-0.00299686489160711));
#91051=CARTESIAN_POINT('Origin',(-14.6,0.,0.));
#91052=CARTESIAN_POINT('',(-17.612836477965,-3.93932967304405,-0.000322413107344821));
#91053=CARTESIAN_POINT('',(-17.796163522035,-3.93933102250188,-0.000314724560625571));
#91054=CARTESIAN_POINT('',(-14.6,-3.933,-4.81653586104654E-16));
#91055=CARTESIAN_POINT('Ctrl Pts',(-17.612836477965,-3.93932967304405,-0.000322413107344821));
#91056=CARTESIAN_POINT('Ctrl Pts',(-17.6778854594652,-3.93781527033072,
1.27990257303665));
#91057=CARTESIAN_POINT('Ctrl Pts',(-17.7429344409653,-3.25516936666837,
2.56151443250391));
#91058=CARTESIAN_POINT('Ctrl Pts',(-17.8079834224655,-2.19131799049156,
3.27363847383026));
#91059=CARTESIAN_POINT('Ctrl Pts',(-17.8739227536112,-1.11290528416235,
3.99550962223137));
#91060=CARTESIAN_POINT('Ctrl Pts',(-17.9398620847569,0.357219713964903,
4.13219667838001));
#91061=CARTESIAN_POINT('Ctrl Pts',(-18.0058014159026,1.5502308934945,3.62151454085841));
#91062=CARTESIAN_POINT('Ctrl Pts',(-18.0717407470483,2.74324207302409,3.11083240333683));
#91063=CARTESIAN_POINT('Ctrl Pts',(-18.137680078194,3.65913943395602,1.95278107214503));
#91064=CARTESIAN_POINT('Ctrl Pts',(-18.2036194093397,3.88123999340509,0.674210283506955));
#91065=CARTESIAN_POINT('Ctrl Pts',(-18.2695587404854,4.10334055285416,-0.604360505131115));
#91066=CARTESIAN_POINT('Ctrl Pts',(-18.3354980716311,3.63164431082037,-2.00345075121548));
#91067=CARTESIAN_POINT('Ctrl Pts',(-18.4014374027768,2.68074714401463,-2.88655125411816));
#91068=CARTESIAN_POINT('Ctrl Pts',(-18.4673767339225,1.72984997720887,-3.76965175702084));
#91069=CARTESIAN_POINT('Ctrl Pts',(-18.5333160650682,0.299751885631159,
-4.13676251674186));
#91070=CARTESIAN_POINT('Ctrl Pts',(-18.5992553962139,-0.958931063858458,
-3.82086830544589));
#91071=CARTESIAN_POINT('Ctrl Pts',(-18.6651947273596,-2.21761401334808,
-3.50497409414993));
#91072=CARTESIAN_POINT('Ctrl Pts',(-18.7311340585053,-3.30488182074959,
-2.50607491183698));
#91073=CARTESIAN_POINT('Ctrl Pts',(-18.797073389651,-3.72608736455351,-1.27861501027807));
#91074=CARTESIAN_POINT('Ctrl Pts',(-18.818994419089,-3.86611394602996,-0.870555295862867));
#91075=CARTESIAN_POINT('Ctrl Pts',(-18.840915448527,-3.9325286924352,-0.437235519605974));
#91076=CARTESIAN_POINT('Ctrl Pts',(-18.862836477965,-3.92942440079457,-0.0029931669997546));
#91077=CARTESIAN_POINT('Ctrl Pts',(-19.046163522035,-3.92943419637598,-0.00299686489160711));
#91078=CARTESIAN_POINT('Ctrl Pts',(-19.0242637951135,-3.93253984081017,
-0.436814413326903));
#91079=CARTESIAN_POINT('Ctrl Pts',(-19.0023640681919,-3.86625723115108,
-0.869709862684471));
#91080=CARTESIAN_POINT('Ctrl Pts',(-18.9804643412704,-3.72649769590772,
-1.27741792446391));
#91081=CARTESIAN_POINT('Ctrl Pts',(-18.9145250101247,-3.30568650003283,
-2.50501299872126));
#91082=CARTESIAN_POINT('Ctrl Pts',(-18.848585678979,-2.2187396911716,-3.50426134057971));
#91083=CARTESIAN_POINT('Ctrl Pts',(-18.7826463478333,-0.960158354132277,
-3.82055984985672));
#91084=CARTESIAN_POINT('Ctrl Pts',(-18.7167070166876,0.298422982907047,
-4.13685835913373));
#91085=CARTESIAN_POINT('Ctrl Pts',(-18.6507676855419,1.72863884812446,-3.7702070358293));
#91086=CARTESIAN_POINT('Ctrl Pts',(-18.5848283543962,2.67981959412393,-2.88741208944908));
#91087=CARTESIAN_POINT('Ctrl Pts',(-18.5188890232505,3.6310003401234,-2.00461714306886));
#91088=CARTESIAN_POINT('Ctrl Pts',(-18.4529496921048,4.10314596690491,-0.605678573612871));
#91089=CARTESIAN_POINT('Ctrl Pts',(-18.3870103609591,3.88145615238507,0.67296342282425));
#91090=CARTESIAN_POINT('Ctrl Pts',(-18.3210710298134,3.65976633786522,1.95160541926137));
#91091=CARTESIAN_POINT('Ctrl Pts',(-18.2551316986677,2.74424108204401,3.10995084267962));
#91092=CARTESIAN_POINT('Ctrl Pts',(-18.189192367522,1.55139408042348,3.62101616104847));
#91093=CARTESIAN_POINT('Ctrl Pts',(-18.1232530363763,0.35854707880295,4.13208147941732));
#91094=CARTESIAN_POINT('Ctrl Pts',(-18.0573137052306,-1.11162166861691,
3.99586669273678));
#91095=CARTESIAN_POINT('Ctrl Pts',(-17.9913743740849,-2.19026614791571,
3.27434204576152));
#91096=CARTESIAN_POINT('Ctrl Pts',(-17.9263040900682,-3.25469463697409,
2.56232672974422));
#91097=CARTESIAN_POINT('Ctrl Pts',(-17.8612338060516,-3.93785103528598,
1.28032806316714));
#91098=CARTESIAN_POINT('Ctrl Pts',(-17.796163522035,-3.93933102250188,-0.000314724560625571));
#91099=CARTESIAN_POINT('Origin',(-14.6,0.,0.));
#91100=CARTESIAN_POINT('',(-16.362836477965,-3.93030695978332,0.00326161695698352));
#91101=CARTESIAN_POINT('',(-16.546163522035,-3.93029567594467,0.0032589082896274));
#91102=CARTESIAN_POINT('',(-14.6,-3.933,-4.81653586104654E-16));
#91103=CARTESIAN_POINT('Ctrl Pts',(-16.362836477965,-3.93030695978332,0.00326161695698352));
#91104=CARTESIAN_POINT('Ctrl Pts',(-16.3829768081119,-3.93346431809964,
0.402003105813639));
#91105=CARTESIAN_POINT('Ctrl Pts',(-16.4031171382588,-3.87761320067396,
0.799880981706207));
#91106=CARTESIAN_POINT('Ctrl Pts',(-16.4232574684057,-3.75907374795352,
1.17811202788205));
#91107=CARTESIAN_POINT('Ctrl Pts',(-16.4891967995514,-3.37097622573056,
2.41643841188208));
#91108=CARTESIAN_POINT('Ctrl Pts',(-16.5551361306971,-2.31091991010657,
3.44416963605641));
#91109=CARTESIAN_POINT('Ctrl Pts',(-16.6210754618428,-1.06117218874064,
3.79374445352307));
#91110=CARTESIAN_POINT('Ctrl Pts',(-16.6870147929885,0.188575532625281,
4.14331927098974));
#91111=CARTESIAN_POINT('Ctrl Pts',(-16.7529541241342,1.62801465973314,3.81473768174875));
#91112=CARTESIAN_POINT('Ctrl Pts',(-16.8188934552799,2.60227946772191,2.95748625773082));
#91113=CARTESIAN_POINT('Ctrl Pts',(-16.8848327864256,3.57654427571069,2.10023483371288));
#91114=CARTESIAN_POINT('Ctrl Pts',(-16.9507721175713,4.08563476458038,0.714313574917998));
#91115=CARTESIAN_POINT('Ctrl Pts',(-17.016711448717,3.89794272962465,-0.569759483782462));
#91116=CARTESIAN_POINT('Ctrl Pts',(-17.0826507798627,3.71025069466892,-1.85383254248292));
#91117=CARTESIAN_POINT('Ctrl Pts',(-17.1485901110084,2.82577613588777,-3.03605740108896));
#91118=CARTESIAN_POINT('Ctrl Pts',(-17.2145294421541,1.6469063874515,-3.57858669641594));
#91119=CARTESIAN_POINT('Ctrl Pts',(-17.2804687732998,0.468036639015227,
-4.12111599174291));
#91120=CARTESIAN_POINT('Ctrl Pts',(-17.3464081044455,-1.00522829907616,
-4.02394972379083));
#91121=CARTESIAN_POINT('Ctrl Pts',(-17.4123474355913,-2.10263381624111,
-3.33129320648799));
#91122=CARTESIAN_POINT('Ctrl Pts',(-17.478286766737,-3.20003933340606,-2.63863668918514));
#91123=CARTESIAN_POINT('Ctrl Pts',(-17.5442260978827,-3.92158542964458,
-1.35048992253154));
#91124=CARTESIAN_POINT('Ctrl Pts',(-17.6101654290284,-3.93900827049825,
-0.0528889188779602));
#91125=CARTESIAN_POINT('Ctrl Pts',(-17.6110557786739,-3.939243523418,-0.035367986020451));
#91126=CARTESIAN_POINT('Ctrl Pts',(-17.6119461283195,-3.93935040123822,
-0.0178453294752127));
#91127=CARTESIAN_POINT('Ctrl Pts',(-17.612836477965,-3.93932967304405,-0.000322413107344821));
#91128=CARTESIAN_POINT('Ctrl Pts',(-17.796163522035,-3.93933102250188,-0.000314724560625571));
#91129=CARTESIAN_POINT('Ctrl Pts',(-17.7952944749059,-3.93935078849277,
-0.0174183680265255));
#91130=CARTESIAN_POINT('Ctrl Pts',(-17.7944254277768,-3.9392489640186,-0.0345217696446254));
#91131=CARTESIAN_POINT('Ctrl Pts',(-17.7935563806478,-3.93902483345017,
-0.0516235683591434));
#91132=CARTESIAN_POINT('Ctrl Pts',(-17.7276170495021,-3.92201882850808,
-1.34923002823458));
#91133=CARTESIAN_POINT('Ctrl Pts',(-17.6616777183564,-3.20088660744617,
-2.63760844071548));
#91134=CARTESIAN_POINT('Ctrl Pts',(-17.5957383872107,-2.10370371425439,
-3.33061740732549));
#91135=CARTESIAN_POINT('Ctrl Pts',(-17.529799056065,-1.00652082106261,-4.02362637393549));
#91136=CARTESIAN_POINT('Ctrl Pts',(-17.4638597249192,0.466712744259044,
-4.12126589467459));
#91137=CARTESIAN_POINT('Ctrl Pts',(-17.3979203937735,1.64575664401571,-3.57911535159533));
#91138=CARTESIAN_POINT('Ctrl Pts',(-17.3319810626278,2.8248005437724,-3.03696480851606));
#91139=CARTESIAN_POINT('Ctrl Pts',(-17.2660417314821,3.70965477796409,-1.85502420161841));
#91140=CARTESIAN_POINT('Ctrl Pts',(-17.2001024003364,3.8977592809668,-0.571011575175547));
#91141=CARTESIAN_POINT('Ctrl Pts',(-17.1341630691907,4.08586378396949,0.713001051267284));
#91142=CARTESIAN_POINT('Ctrl Pts',(-17.068223738045,3.57721855578324,2.09908569725531));
#91143=CARTESIAN_POINT('Ctrl Pts',(-17.0022844068993,2.60322923196453,2.95664999572026));
#91144=CARTESIAN_POINT('Ctrl Pts',(-16.9363450757536,1.62923990814581,3.81421429418521));
#91145=CARTESIAN_POINT('Ctrl Pts',(-16.8704057446079,0.189906488694602,
4.14325824512707));
#91146=CARTESIAN_POINT('Ctrl Pts',(-16.8044664134622,-1.05995339270459,
3.79408492744183));
#91147=CARTESIAN_POINT('Ctrl Pts',(-16.7385270823165,-2.3098132741038,3.44491160975658));
#91148=CARTESIAN_POINT('Ctrl Pts',(-16.6725877511708,-3.37019961745101,
2.41752102344424));
#91149=CARTESIAN_POINT('Ctrl Pts',(-16.6066484200251,-3.75869489060368,
1.17931944387305));
#91150=CARTESIAN_POINT('Ctrl Pts',(-16.5864867873617,-3.87748133949039,
0.800726501288189));
#91151=CARTESIAN_POINT('Ctrl Pts',(-16.5663251546984,-3.93345310289138,
0.40242496779342));
#91152=CARTESIAN_POINT('Ctrl Pts',(-16.546163522035,-3.93029567594467,0.0032589082896274));
#91153=CARTESIAN_POINT('Origin',(-14.6,0.,0.));
#91154=CARTESIAN_POINT('',(-15.112836477965,-3.92822229680268,-0.00240354736792903));
#91155=CARTESIAN_POINT('',(-15.296163522035,-3.92822997878168,-0.00240860774561585));
#91156=CARTESIAN_POINT('',(-14.6,-3.933,-4.81653586104654E-16));
#91157=CARTESIAN_POINT('Ctrl Pts',(-15.112836477965,-3.92822229680268,-0.00240354736792903));
#91158=CARTESIAN_POINT('Ctrl Pts',(-15.1540074879044,-3.92363278539411,
0.813797469098643));
#91159=CARTESIAN_POINT('Ctrl Pts',(-15.1951784978437,-3.67557873714955,
1.63255455559306));
#91160=CARTESIAN_POINT('Ctrl Pts',(-15.2363495077831,-3.20422949520173,
2.29161443852864));
#91161=CARTESIAN_POINT('Ctrl Pts',(-15.3022888389288,-2.44931836244454,
3.34716221182241));
#91162=CARTESIAN_POINT('Ctrl Pts',(-15.3682281700745,-1.12163044217474,
3.99306905325299));
#91163=CARTESIAN_POINT('Ctrl Pts',(-15.4341675012202,0.174809200620274,
3.93548283393184));
#91164=CARTESIAN_POINT('Ctrl Pts',(-15.5001068323659,1.47124884341531,3.87789661461069));
#91165=CARTESIAN_POINT('Ctrl Pts',(-15.5660461635116,2.73644020873557,3.11681733453777));
#91166=CARTESIAN_POINT('Ctrl Pts',(-15.6319854946573,3.39479073074392,1.99849425499521));
#91167=CARTESIAN_POINT('Ctrl Pts',(-15.697924825803,4.05314125275225,0.880171175452675));
#91168=CARTESIAN_POINT('Ctrl Pts',(-15.7638641569487,4.1046509314487,-0.595395703559483));
#91169=CARTESIAN_POINT('Ctrl Pts',(-15.8298034880944,3.52588569279593,-1.75690451480171));
#91170=CARTESIAN_POINT('Ctrl Pts',(-15.8957428192401,2.94712045414315,-2.91841332604395));
#91171=CARTESIAN_POINT('Ctrl Pts',(-15.9616821503858,1.73808029814112,-3.76586406951625));
#91172=CARTESIAN_POINT('Ctrl Pts',(-16.0276214815315,0.448812075146874,
-3.91371321304922));
#91173=CARTESIAN_POINT('Ctrl Pts',(-16.0935608126772,-0.840456147847376,
-4.06156235658218));
#91174=CARTESIAN_POINT('Ctrl Pts',(-16.1595001438229,-2.20995243783385,
-3.50980990017581));
#91175=CARTESIAN_POINT('Ctrl Pts',(-16.2254394749686,-3.03663121841612,
-2.50947290005976));
#91176=CARTESIAN_POINT('Ctrl Pts',(-16.2712384759674,-3.61081147835717,
-1.81467611532709));
#91177=CARTESIAN_POINT('Ctrl Pts',(-16.3170374769662,-3.92312714417811,
-0.903474355751184));
#91178=CARTESIAN_POINT('Ctrl Pts',(-16.362836477965,-3.93030695978332,0.00326161695698352));
#91179=CARTESIAN_POINT('Ctrl Pts',(-16.546163522035,-3.93029567594467,0.0032589082896274));
#91180=CARTESIAN_POINT('Ctrl Pts',(-16.5003858235527,-3.92312662663404,
-0.903061716702896));
#91181=CARTESIAN_POINT('Ctrl Pts',(-16.4546081250703,-3.61112705848366,
-1.81383925900364));
#91182=CARTESIAN_POINT('Ctrl Pts',(-16.408830426588,-3.03743701831446,-2.50849715788562));
#91183=CARTESIAN_POINT('Ctrl Pts',(-16.3428910954423,-2.21107966991449,
-3.50909960724294));
#91184=CARTESIAN_POINT('Ctrl Pts',(-16.2769517642966,-0.841760770156474,
-4.0612919331276));
#91185=CARTESIAN_POINT('Ctrl Pts',(-16.2110124331509,0.447554807371917,
-3.91385696286228));
#91186=CARTESIAN_POINT('Ctrl Pts',(-16.1450731020052,1.73687038490033,-3.76642199259695));
#91187=CARTESIAN_POINT('Ctrl Pts',(-16.0791337708595,2.9461826401991,-2.91935972618162));
#91188=CARTESIAN_POINT('Ctrl Pts',(-16.0131944397138,3.52532093267943,-1.75803696006639));
#91189=CARTESIAN_POINT('Ctrl Pts',(-15.9472551085681,4.10445922515975,-0.596714193951166));
#91190=CARTESIAN_POINT('Ctrl Pts',(-15.8813157774224,4.05342355482162,0.878869071863958));
#91191=CARTESIAN_POINT('Ctrl Pts',(-15.8153764462767,3.39543234793979,1.9974035150443));
#91192=CARTESIAN_POINT('Ctrl Pts',(-15.749437115131,2.73744114105796,3.11593795822463));
#91193=CARTESIAN_POINT('Ctrl Pts',(-15.6834977839853,1.47249439763243,3.87742357877017));
#91194=CARTESIAN_POINT('Ctrl Pts',(-15.6175584528396,0.176073393976921,
3.93542625280676));
#91195=CARTESIAN_POINT('Ctrl Pts',(-15.5516191216939,-1.12034760967857,
3.99342892684335));
#91196=CARTESIAN_POINT('Ctrl Pts',(-15.4856797905482,-2.44824287356404,
3.34794865437101));
#91197=CARTESIAN_POINT('Ctrl Pts',(-15.4197404594025,-3.20349300273775,
2.29264349883656));
#91198=CARTESIAN_POINT('Ctrl Pts',(-15.3785481469467,-3.67529789918852,
1.63339417149699));
#91199=CARTESIAN_POINT('Ctrl Pts',(-15.3373558344908,-3.92362784693915,
0.814210551230189));
#91200=CARTESIAN_POINT('Ctrl Pts',(-15.296163522035,-3.92822997878168,-0.00240860774561585));
#91201=CARTESIAN_POINT('Origin',(-14.6,0.,0.));
#91202=CARTESIAN_POINT('',(-13.862836477965,-3.93881447356001,-0.00131697643526163));
#91203=CARTESIAN_POINT('',(-14.046163522035,-3.93882016358904,-0.0013098913562943));
#91204=CARTESIAN_POINT('',(-14.6,-3.933,-4.81653586104654E-16));
#91205=CARTESIAN_POINT('Ctrl Pts',(-13.862836477965,-3.93881447356001,-0.00131697643526163));
#91206=CARTESIAN_POINT('Ctrl Pts',(-13.9250381676968,-3.93345678725095,
1.2232994368523));
#91207=CARTESIAN_POINT('Ctrl Pts',(-13.9872398574286,-3.31693161062816,
2.45257298663125));
#91208=CARTESIAN_POINT('Ctrl Pts',(-14.0494415471604,-2.32981268385847,
3.17656359151299));
#91209=CARTESIAN_POINT('Ctrl Pts',(-14.1153808783061,-1.28337870315618,
3.94405811533566));
#91210=CARTESIAN_POINT('Ctrl Pts',(-14.1813202094518,0.179524393308559,
4.143721311221));
#91211=CARTESIAN_POINT('Ctrl Pts',(-14.2472595405975,1.39335606364934,3.68471739386962));
#91212=CARTESIAN_POINT('Ctrl Pts',(-14.3131988717432,2.60718773399009,3.22571347651824));
#91213=CARTESIAN_POINT('Ctrl Pts',(-14.3791382028889,3.57194797820692,2.10804244593017));
#91214=CARTESIAN_POINT('Ctrl Pts',(-14.4450775340346,3.84872388588344,0.840183219913357));
#91215=CARTESIAN_POINT('Ctrl Pts',(-14.5110168651803,4.12549979355995,-0.427676006103479));
#91216=CARTESIAN_POINT('Ctrl Pts',(-14.576956196326,3.71429136469616,-1.84572342754904));
#91217=CARTESIAN_POINT('Ctrl Pts',(-14.6428955274717,2.80217584400881,-2.76882537044993));
#91218=CARTESIAN_POINT('Ctrl Pts',(-14.7088348586174,1.89006032332144,-3.69192731335084));
#91219=CARTESIAN_POINT('Ctrl Pts',(-14.7747741897631,0.477037710810491,
-4.12008377770702));
#91220=CARTESIAN_POINT('Ctrl Pts',(-14.8407135209088,-0.794044331569596,
-3.85850709372108));
#91221=CARTESIAN_POINT('Ctrl Pts',(-14.9066528520546,-2.06512637394967,
-3.59693040973513));
#91222=CARTESIAN_POINT('Ctrl Pts',(-14.9725921832003,-3.19426784619889,
-2.64562057740708));
#91223=CARTESIAN_POINT('Ctrl Pts',(-15.038531514346,-3.6677714097012,-1.43737130866458));
#91224=CARTESIAN_POINT('Ctrl Pts',(-15.0632998355523,-3.84563018001938,
-0.983525243416702));
#91225=CARTESIAN_POINT('Ctrl Pts',(-15.0880681567587,-3.93098332921153,
-0.493426939181124));
#91226=CARTESIAN_POINT('Ctrl Pts',(-15.112836477965,-3.92822229680268,-0.00240354736792903));
#91227=CARTESIAN_POINT('Ctrl Pts',(-15.296163522035,-3.92822997878168,-0.00240860774561585));
#91228=CARTESIAN_POINT('Ctrl Pts',(-15.2714165033451,-3.93099479182398,
-0.49300717783927));
#91229=CARTESIAN_POINT('Ctrl Pts',(-15.2466694846552,-3.84579285967439,
-0.982680177283143));
#91230=CARTESIAN_POINT('Ctrl Pts',(-15.2219224659653,-3.66823274535127,
-1.43619293873765));
#91231=CARTESIAN_POINT('Ctrl Pts',(-15.1559831348196,-3.19511736432913,
-2.64459418218073));
#91232=CARTESIAN_POINT('Ctrl Pts',(-15.090043803674,-2.06628160782294,-3.59626663047032));
#91233=CARTESIAN_POINT('Ctrl Pts',(-15.0241044725283,-0.795283730580655,
-3.85825160133719));
#91234=CARTESIAN_POINT('Ctrl Pts',(-14.9581651413826,0.475714146661664,
-4.12023657220405));
#91235=CARTESIAN_POINT('Ctrl Pts',(-14.8922258102368,1.88887414464008,-3.69253406564815));
#91236=CARTESIAN_POINT('Ctrl Pts',(-14.8262864790911,2.80128609855997,-2.76972522560667));
#91237=CARTESIAN_POINT('Ctrl Pts',(-14.7603471479454,3.71369805247985,-1.84691638556519));
#91238=CARTESIAN_POINT('Ctrl Pts',(-14.6944078167997,4.1253619623412,-0.429001212038141));
#91239=CARTESIAN_POINT('Ctrl Pts',(-14.628468485654,3.84899336459595,0.838946786538663));
#91240=CARTESIAN_POINT('Ctrl Pts',(-14.5625291545083,3.57262476685072,2.10689478511543));
#91241=CARTESIAN_POINT('Ctrl Pts',(-14.4965898233626,2.60822366149893,3.22487560874196));
#91242=CARTESIAN_POINT('Ctrl Pts',(-14.4306504922169,1.39453957050327,3.68426940079682));
#91243=CARTESIAN_POINT('Ctrl Pts',(-14.3647111610712,0.180855479507593,
4.14366319285169));
#91244=CARTESIAN_POINT('Ctrl Pts',(-14.2987718299255,-1.28211159713196,
3.94446995333486));
#91245=CARTESIAN_POINT('Ctrl Pts',(-14.2328324987798,-2.32879201006434,
3.17731166321589));
#91246=CARTESIAN_POINT('Ctrl Pts',(-14.1706095065316,-3.3164815435904,2.45339039331705));
#91247=CARTESIAN_POINT('Ctrl Pts',(-14.1083865142833,-3.93348591101852,
1.22372095160461));
#91248=CARTESIAN_POINT('Ctrl Pts',(-14.046163522035,-3.93882016358904,-0.0013098913562943));
#91249=CARTESIAN_POINT('Origin',(-14.6,0.,0.));
#91250=CARTESIAN_POINT('',(-12.612836477965,-3.9318717373109,0.00350585034690487));
#91251=CARTESIAN_POINT('',(-12.796163522035,-3.93185928339207,0.00350492153532546));
#91252=CARTESIAN_POINT('',(-14.6,-3.933,-4.81653586104654E-16));
#91253=CARTESIAN_POINT('Ctrl Pts',(-12.612836477965,-3.9318717373109,0.00350585034690487));
#91254=CARTESIAN_POINT('Ctrl Pts',(-12.6301295163436,-3.93487740264675,
0.345530407337765));
#91255=CARTESIAN_POINT('Ctrl Pts',(-12.6474225547221,-3.89392515658943,
0.686846730394007));
#91256=CARTESIAN_POINT('Ctrl Pts',(-12.6647155931007,-3.80617738217334,
1.01567570032258));
#91257=CARTESIAN_POINT('Ctrl Pts',(-12.7306549242464,-3.47159016691004,
2.26951911775896));
#91258=CARTESIAN_POINT('Ctrl Pts',(-12.7965942553921,-2.45662407837034,
3.34180392160147));
#91259=CARTESIAN_POINT('Ctrl Pts',(-12.8625335865378,-1.2230329279963,3.74469943384385));
#91260=CARTESIAN_POINT('Ctrl Pts',(-12.9284729176835,0.0105582223777351,
4.14759494608623));
#91261=CARTESIAN_POINT('Ctrl Pts',(-12.9944122488292,1.46277443458609,3.88110116672849));
#91262=CARTESIAN_POINT('Ctrl Pts',(-13.0603515799749,2.47293711197736,3.06645812510113));
#91263=CARTESIAN_POINT('Ctrl Pts',(-13.1262909111206,3.48309978936863,2.25181508347378));
#91264=CARTESIAN_POINT('Ctrl Pts',(-13.1922302422663,4.05120893194283,0.889022779576799));
#91265=CARTESIAN_POINT('Ctrl Pts',(-13.258169573412,3.91880608984557,-0.401923155569485));
#91266=CARTESIAN_POINT('Ctrl Pts',(-13.3241089045577,3.78640324774831,-1.69286909071581));
#91267=CARTESIAN_POINT('Ctrl Pts',(-13.3900482357034,2.95348842097959,-2.91196865711145));
#91268=CARTESIAN_POINT('Ctrl Pts',(-13.4559875668491,1.79899209816333,-3.50459852530066));
#91269=CARTESIAN_POINT('Ctrl Pts',(-13.5219268979948,0.644495775347081,
-4.09722839348988));
#91270=CARTESIAN_POINT('Ctrl Pts',(-13.5878662291405,-0.831582043516668,
-4.06338856347267));
#91271=CARTESIAN_POINT('Ctrl Pts',(-13.6538055602862,-1.95770704162521,
-3.41847429885976));
#91272=CARTESIAN_POINT('Ctrl Pts',(-13.7197448914319,-3.08383203973376,
-2.77356003424685));
#91273=CARTESIAN_POINT('Ctrl Pts',(-13.7856842225776,-3.86000421708709,
-1.51757133503824));
#91274=CARTESIAN_POINT('Ctrl Pts',(-13.8516235537233,-3.93310787329384,
-0.221914059553938));
#91275=CARTESIAN_POINT('Ctrl Pts',(-13.8553611951372,-3.93725161039578,
-0.148472272885356));
#91276=CARTESIAN_POINT('Ctrl Pts',(-13.8590988365511,-3.93913641192402,
-0.0749030324119008));
#91277=CARTESIAN_POINT('Ctrl Pts',(-13.862836477965,-3.93881447356001,-0.00131697643526163));
#91278=CARTESIAN_POINT('Ctrl Pts',(-14.046163522035,-3.93882016358904,-0.0013098913562943));
#91279=CARTESIAN_POINT('Ctrl Pts',(-14.0424471831376,-3.93913875788354,
-0.074476250088611));
#91280=CARTESIAN_POINT('Ctrl Pts',(-14.0387308442401,-3.9372753956192,-0.147626061958944));
#91281=CARTESIAN_POINT('Ctrl Pts',(-14.0350145053427,-3.9331787335674,-0.220650586131847));
#91282=CARTESIAN_POINT('Ctrl Pts',(-13.969075174197,-3.8604912949129,-1.51633120463951));
#91283=CARTESIAN_POINT('Ctrl Pts',(-13.9031358430513,-3.08472266837869,
-2.77256910093373));
#91284=CARTESIAN_POINT('Ctrl Pts',(-13.8371965119056,-1.95880496090319,
-3.41784504571058));
#91285=CARTESIAN_POINT('Ctrl Pts',(-13.7712571807599,-0.832887253427681,
-4.06312099048742));
#91286=CARTESIAN_POINT('Ctrl Pts',(-13.7053178496142,0.64317953498912,-4.0974349837469));
#91287=CARTESIAN_POINT('Ctrl Pts',(-13.6393785184685,1.79786610579188,-3.50517604365201));
#91288=CARTESIAN_POINT('Ctrl Pts',(-13.5734391873228,2.95255267659464,-2.91291710355713));
#91289=CARTESIAN_POINT('Ctrl Pts',(-13.5074998561771,3.78585902978335,-1.69408523010788));
#91290=CARTESIAN_POINT('Ctrl Pts',(-13.4415605250314,3.91867655372215,-0.403181967175553));
#91291=CARTESIAN_POINT('Ctrl Pts',(-13.3756211938857,4.05149407766094,0.88772129575677));
#91292=CARTESIAN_POINT('Ctrl Pts',(-13.30968186274,3.48382277234982,2.25069594817216));
#91293=CARTESIAN_POINT('Ctrl Pts',(-13.2437425315943,2.47392189574176,3.06566340049209));
#91294=CARTESIAN_POINT('Ctrl Pts',(-13.1778032004486,1.46402101913371,3.88063085281201));
#91295=CARTESIAN_POINT('Ctrl Pts',(-13.1118638693029,0.0118905712287158,
4.14759110503647));
#91296=CARTESIAN_POINT('Ctrl Pts',(-13.0459245381572,-1.22182986936823,
3.74509190830704));
#91297=CARTESIAN_POINT('Ctrl Pts',(-12.9799852070115,-2.45555030996515,
3.34259271157761));
#91298=CARTESIAN_POINT('Ctrl Pts',(-12.9140458758658,-3.47086074325403,
2.27063406589432));
#91299=CARTESIAN_POINT('Ctrl Pts',(-12.8481065447201,-3.80585069984909,
1.01689826521902));
#91300=CARTESIAN_POINT('Ctrl Pts',(-12.830792203825,-3.89381231856922,0.687692483661536));
#91301=CARTESIAN_POINT('Ctrl Pts',(-12.81347786293,-3.93486707364353,0.345953496776215));
#91302=CARTESIAN_POINT('Ctrl Pts',(-12.796163522035,-3.93185928339207,0.00350492153532546));
#91303=CARTESIAN_POINT('Origin',(-14.6,0.,0.));
#91304=CARTESIAN_POINT('',(-11.362836477965,-3.92733190008639,-0.00165504447000753));
#91305=CARTESIAN_POINT('',(-11.546163522035,-3.92733705745214,-0.0016611125421626));
#91306=CARTESIAN_POINT('',(-14.6,-3.933,-4.81653586104654E-16));
#91307=CARTESIAN_POINT('Ctrl Pts',(-11.362836477965,-3.92733190008639,-0.00165504447000753));
#91308=CARTESIAN_POINT('Ctrl Pts',(-11.401160196136,-3.92443034344515,0.758531279775249));
#91309=CARTESIAN_POINT('Ctrl Pts',(-11.439483914307,-3.71165434622295,1.52021948759287));
#91310=CARTESIAN_POINT('Ctrl Pts',(-11.477807632478,-3.29963929855811,2.15196744682735));
#91311=CARTESIAN_POINT('Ctrl Pts',(-11.5437469636237,-2.59073113511326,
3.23894542998406));
#91312=CARTESIAN_POINT('Ctrl Pts',(-11.6096862947694,-1.2919910634956,3.94124528603681));
#91313=CARTESIAN_POINT('Ctrl Pts',(-11.6756256259151,0.0057255321462002,
3.93935916248764));
#91314=CARTESIAN_POINT('Ctrl Pts',(-11.7415649570608,1.303442127788,3.93747303893847));
#91315=CARTESIAN_POINT('Ctrl Pts',(-11.8075042882065,2.60013524745393,3.23140093578738));
#91316=CARTESIAN_POINT('Ctrl Pts',(-11.8734436193522,3.30588075768066,2.14236687072743));
#91317=CARTESIAN_POINT('Ctrl Pts',(-11.9393829504979,4.01162626790739,1.05333280566748));
#91318=CARTESIAN_POINT('Ctrl Pts',(-12.0053222816437,4.12642416869491,-0.418663221301322));
#91319=CARTESIAN_POINT('Ctrl Pts',(-12.0712616127894,3.59804772179776,-1.60394388444846));
#91320=CARTESIAN_POINT('Ctrl Pts',(-12.1372009439351,3.06967127490061,-2.7892245475956));
#91321=CARTESIAN_POINT('Ctrl Pts',(-12.2031402750808,1.89812048031879,-3.68778984692108));
#91322=CARTESIAN_POINT('Ctrl Pts',(-12.2690796062265,0.616386588503315,
-3.8908419354051));
#91323=CARTESIAN_POINT('Ctrl Pts',(-12.3350189373722,-0.665347303312165,
-4.09389402388912));
#91324=CARTESIAN_POINT('Ctrl Pts',(-12.4009582685179,-2.0572642923613,-3.60143290153169));
#91325=CARTESIAN_POINT('Ctrl Pts',(-12.4668975996636,-2.92611861589242,
-2.63750132483786));
#91326=CARTESIAN_POINT('Ctrl Pts',(-12.5155438924307,-3.56710997962201,
-1.92636736468688));
#91327=CARTESIAN_POINT('Ctrl Pts',(-12.5641901851979,-3.92341663111804,
-0.958628528165194));
#91328=CARTESIAN_POINT('Ctrl Pts',(-12.612836477965,-3.9318717373109,0.00350585034690487));
#91329=CARTESIAN_POINT('Ctrl Pts',(-12.796163522035,-3.93185928339207,0.00350492153532546));
#91330=CARTESIAN_POINT('Ctrl Pts',(-12.7475385317843,-3.92341231029966,
-0.958215696846525));
#91331=CARTESIAN_POINT('Ctrl Pts',(-12.6989135415336,-3.56744781444277,
-1.92553277784049));
#91332=CARTESIAN_POINT('Ctrl Pts',(-12.650288551283,-2.92696555489341,-2.63656106923674));
#91333=CARTESIAN_POINT('Ctrl Pts',(-12.5843492201373,-2.0584209734415,-3.60077164734977));
#91334=CARTESIAN_POINT('Ctrl Pts',(-12.5184098889916,-0.666662330636484,
-4.09367984790849));
#91335=CARTESIAN_POINT('Ctrl Pts',(-12.4524705578459,0.615136649612009,
-3.89103951838726));
#91336=CARTESIAN_POINT('Ctrl Pts',(-12.3865312267001,1.89693562986052,-3.68839918886602));
#91337=CARTESIAN_POINT('Ctrl Pts',(-12.3205918955544,3.06877494755251,-2.7902103292648));
#91338=CARTESIAN_POINT('Ctrl Pts',(-12.2546525644087,3.59753209007232,-1.60509952720919));
#91339=CARTESIAN_POINT('Ctrl Pts',(-12.188713233263,4.12628923259211,-0.419988725153615));
#91340=CARTESIAN_POINT('Ctrl Pts',(-12.1227739021173,4.01196419993977,1.05204401935632));
#91341=CARTESIAN_POINT('Ctrl Pts',(-12.0568345709716,3.30656860133704,2.14130467612604));
#91342=CARTESIAN_POINT('Ctrl Pts',(-11.9908952398259,2.6011730027343,3.23056533289578));
#91343=CARTESIAN_POINT('Ctrl Pts',(-11.9249559086802,1.30470683818116,3.93705390192528));
#91344=CARTESIAN_POINT('Ctrl Pts',(-11.8590165775345,0.0069909890327869,
3.93935689642606));
#91345=CARTESIAN_POINT('Ctrl Pts',(-11.7930772463888,-1.29072486011559,
3.94165989092684));
#91346=CARTESIAN_POINT('Ctrl Pts',(-11.7271379152431,-2.58969039385919,
3.23977731089889));
#91347=CARTESIAN_POINT('Ctrl Pts',(-11.6611985840974,-3.29894765516817,
2.15302717117264));
#91348=CARTESIAN_POINT('Ctrl Pts',(-11.6228535634099,-3.71139473167168,
1.52106054570216));
#91349=CARTESIAN_POINT('Ctrl Pts',(-11.5845085427225,-3.92442300853275,
0.758945115536301));
#91350=CARTESIAN_POINT('Ctrl Pts',(-11.546163522035,-3.92733705745214,-0.0016611125421626));
#91351=CARTESIAN_POINT('Origin',(-14.6,0.,0.));
#91352=CARTESIAN_POINT('',(-10.112836477965,-3.93779509892002,-0.00218943587030118));
#91353=CARTESIAN_POINT('',(-10.296163522035,-3.93780400755292,-0.00218353918451927));
#91354=CARTESIAN_POINT('',(-14.6,-3.933,-4.81653586104654E-16));
#91355=CARTESIAN_POINT('Ctrl Pts',(-10.112836477965,-3.93779509892002,-0.00218943587030118));
#91356=CARTESIAN_POINT('Ctrl Pts',(-10.1721908759285,-3.9299575440291,1.167171333214));
#91357=CARTESIAN_POINT('Ctrl Pts',(-10.2315452738919,-3.37542498846826,
2.34298987769126));
#91358=CARTESIAN_POINT('Ctrl Pts',(-10.2908996718554,-2.46401299743278,
3.07363357303306));
#91359=CARTESIAN_POINT('Ctrl Pts',(-10.3568390030011,-1.45148656048612,
3.88533680362308));
#91360=CARTESIAN_POINT('Ctrl Pts',(-10.4227783341468,0.00149816796940136,
4.14760811412465));
#91361=CARTESIAN_POINT('Ctrl Pts',(-10.4887176652925,1.23391295860962,3.74112846656847));
#91362=CARTESIAN_POINT('Ctrl Pts',(-10.5546569964382,2.46632774924983,3.33464881901229));
#91363=CARTESIAN_POINT('Ctrl Pts',(-10.6205963275839,3.47817260207474,2.2594182133984));
#91364=CARTESIAN_POINT('Ctrl Pts',(-10.6865356587296,3.80911369642228,1.00460750570652));
#91365=CARTESIAN_POINT('Ctrl Pts',(-10.7524749898753,4.14005479076982,-0.25020320198539));
#91366=CARTESIAN_POINT('Ctrl Pts',(-10.818414321021,3.79009212663995,-1.68459401175529));
#91367=CARTESIAN_POINT('Ctrl Pts',(-10.8843536521667,2.91843949043304,-2.64599590579325));
#91368=CARTESIAN_POINT('Ctrl Pts',(-10.9502929833124,2.04678685422614,-3.60739779983119));
#91369=CARTESIAN_POINT('Ctrl Pts',(-11.0162323144581,0.653444245942222,
-4.0958107781372));
#91370=CARTESIAN_POINT('Ctrl Pts',(-11.0821716456038,-0.627693993233959,
-3.88903376735812));
#91371=CARTESIAN_POINT('Ctrl Pts',(-11.1481109767495,-1.90883223241014,
-3.68225675657904));
#91372=CARTESIAN_POINT('Ctrl Pts',(-11.2140503078952,-3.07776610247859,
-2.78028975671487));
#91373=CARTESIAN_POINT('Ctrl Pts',(-11.2799896390409,-3.6026949098768,-1.59347820165245));
#91374=CARTESIAN_POINT('Ctrl Pts',(-11.3076052520156,-3.82253685447201,
-1.09643754307974));
#91375=CARTESIAN_POINT('Ctrl Pts',(-11.3352208649903,-3.92942272710039,
-0.549436218137531));
#91376=CARTESIAN_POINT('Ctrl Pts',(-11.362836477965,-3.92733190008639,-0.00165504447000753));
#91377=CARTESIAN_POINT('Ctrl Pts',(-11.546163522035,-3.92733705745214,-0.0016611125421626));
#91378=CARTESIAN_POINT('Ctrl Pts',(-11.5185692115768,-3.92943410080041,
-0.549017823211577));
#91379=CARTESIAN_POINT('Ctrl Pts',(-11.4909749011185,-3.82271919215505,
-1.09559296270092));
#91380=CARTESIAN_POINT('Ctrl Pts',(-11.4633805906603,-3.60320639947517,
-1.59232071961913));
#91381=CARTESIAN_POINT('Ctrl Pts',(-11.3974412595146,-3.07865889359882,
-2.77930077126006));
#91382=CARTESIAN_POINT('Ctrl Pts',(-11.3315019283689,-1.91001489297174,
-3.68164317511733));
#91383=CARTESIAN_POINT('Ctrl Pts',(-11.2655625972232,-0.628943216485102,
-3.88883170911067));
#91384=CARTESIAN_POINT('Ctrl Pts',(-11.1996232660775,0.652128460001497,
-4.096020243104));
#91385=CARTESIAN_POINT('Ctrl Pts',(-11.1336839349318,2.04562781234766,-3.60805490723346));
#91386=CARTESIAN_POINT('Ctrl Pts',(-11.0677446037861,2.91758918943131,-2.64693312213603));
#91387=CARTESIAN_POINT('Ctrl Pts',(-11.0018052726404,3.78955056651497,-1.68581133703858));
#91388=CARTESIAN_POINT('Ctrl Pts',(-10.9358659414947,4.13997396833612,-0.251533102714276));
#91389=CARTESIAN_POINT('Ctrl Pts',(-10.869926610349,3.80943599815624,1.00338377867027));
#91390=CARTESIAN_POINT('Ctrl Pts',(-10.8039872792033,3.47889802797636,2.25830066005483));
#91391=CARTESIAN_POINT('Ctrl Pts',(-10.7380479480576,2.4673986857954,3.33385618849958));
#91392=CARTESIAN_POINT('Ctrl Pts',(-10.6721086169119,1.23511460391369,3.7407316859869));
#91393=CARTESIAN_POINT('Ctrl Pts',(-10.6061692857662,0.0028305220320006,
4.1476071834742));
#91394=CARTESIAN_POINT('Ctrl Pts',(-10.5402299546205,-1.45023829955045,
3.88580265000409));
#91395=CARTESIAN_POINT('Ctrl Pts',(-10.4742906234748,-2.46302537375653,
3.07442476563971));
#91396=CARTESIAN_POINT('Ctrl Pts',(-10.4149149229948,-3.37499916729004,
2.34381180064602));
#91397=CARTESIAN_POINT('Ctrl Pts',(-10.3555392225149,-3.92998045545785,
1.16758970334765));
#91398=CARTESIAN_POINT('Ctrl Pts',(-10.296163522035,-3.93780400755292,-0.00218353918451927));
#91399=CARTESIAN_POINT('Origin',(-14.6,0.,0.));
#91400=CARTESIAN_POINT('',(-8.86283647796501,-3.93354422253028,0.0035021652868221));
#91401=CARTESIAN_POINT('',(-9.04616352203496,-3.93353134025131,0.00350314687873205));
#91402=CARTESIAN_POINT('',(-14.6,-3.933,-4.81653586104654E-16));
#91403=CARTESIAN_POINT('Ctrl Pts',(-8.86283647796501,-3.93354422253028,
0.0035021652868221));
#91404=CARTESIAN_POINT('Ctrl Pts',(-8.87728222457522,-3.93615140491192,
0.288902068067195));
#91405=CARTESIAN_POINT('Ctrl Pts',(-8.89172797118542,-3.9077075457056,0.573786733317711));
#91406=CARTESIAN_POINT('Ctrl Pts',(-8.90617371779562,-3.84626535743036,
0.851367249208478));
#91407=CARTESIAN_POINT('Ctrl Pts',(-8.97211304894133,-3.56580517019878,
2.11841657873129));
#91408=CARTESIAN_POINT('Ctrl Pts',(-9.03805238008703,-2.59780012432051,
3.23327849510991));
#91409=CARTESIAN_POINT('Ctrl Pts',(-9.10399171123273,-1.38263933670938,
3.68875207317834));
#91410=CARTESIAN_POINT('Ctrl Pts',(-9.16993104237844,-0.16747854909823,
4.14422565124678));
#91411=CARTESIAN_POINT('Ctrl Pts',(-9.23587037352414,1.29483798024581,3.94031089100503));
#91412=CARTESIAN_POINT('Ctrl Pts',(-9.30180970466984,2.33903656525223,3.16977780596791));
#91413=CARTESIAN_POINT('Ctrl Pts',(-9.36774903581554,3.38323515025861,2.39924472093081));
#91414=CARTESIAN_POINT('Ctrl Pts',(-9.43368836696125,4.00931579092741,1.06209331109839));
#91415=CARTESIAN_POINT('Ctrl Pts',(-9.49962769810695,3.93244619053149,-0.233345990683485));
#91416=CARTESIAN_POINT('Ctrl Pts',(-9.56556702925265,3.85557659013557,-1.52878529246538));
#91417=CARTESIAN_POINT('Ctrl Pts',(-9.63150636039835,3.07575674867495,-2.78251248619667));
#91418=CARTESIAN_POINT('Ctrl Pts',(-9.69744569154406,1.94776185331931,-3.42415057431005));
#91419=CARTESIAN_POINT('Ctrl Pts',(-9.76338502268976,0.819766957963639,
-4.06578866242344));
#91420=CARTESIAN_POINT('Ctrl Pts',(-9.82932435383547,-0.656402991287067,
-4.09533764491883));
#91421=CARTESIAN_POINT('Ctrl Pts',(-9.89526368498117,-1.80917176336531,
-3.49935435808312));
#91422=CARTESIAN_POINT('Ctrl Pts',(-9.96120301612687,-2.96194053544351,
-2.90337107124743));
#91423=CARTESIAN_POINT('Ctrl Pts',(-10.0271423472726,-3.79130813034929,
-1.68185551508067));
#91424=CARTESIAN_POINT('Ctrl Pts',(-10.0930816784183,-3.91995785508327,
-0.390530161658051));
#91425=CARTESIAN_POINT('Ctrl Pts',(-10.0996666116005,-3.93280526840349,
-0.261573876826474));
#91426=CARTESIAN_POINT('Ctrl Pts',(-10.1062515447828,-3.93866461789486,
-0.131921398362811));
#91427=CARTESIAN_POINT('Ctrl Pts',(-10.112836477965,-3.93779509892002,-0.00218943587030118));
#91428=CARTESIAN_POINT('Ctrl Pts',(-10.296163522035,-3.93780400755292,-0.00218353918451927));
#91429=CARTESIAN_POINT('Ctrl Pts',(-10.2895998913692,-3.93866885472156,
-0.131495016179637));
#91430=CARTESIAN_POINT('Ctrl Pts',(-10.2830362607034,-3.93284744093761,
-0.26072768824709));
#91431=CARTESIAN_POINT('Ctrl Pts',(-10.2764726300377,-3.92008288206673,
-0.389270894204289));
#91432=CARTESIAN_POINT('Ctrl Pts',(-10.210533298892,-3.79184798934113,-1.68063743442522));
#91433=CARTESIAN_POINT('Ctrl Pts',(-10.1445939677463,-2.96287287706023,
-2.90241927960841));
#91434=CARTESIAN_POINT('Ctrl Pts',(-10.0786546366006,-1.81029568019072,
-3.49877281080525));
#91435=CARTESIAN_POINT('Ctrl Pts',(-10.0127153054549,-0.657718483321177,
-4.09512634200211));
#91436=CARTESIAN_POINT('Ctrl Pts',(-9.94677597430915,0.818460798136971,
-4.06605155921256));
#91437=CARTESIAN_POINT('Ctrl Pts',(-9.88083664316344,1.94666168747457,-3.42477589133448));
#91438=CARTESIAN_POINT('Ctrl Pts',(-9.81489731201774,3.07486257681215,-2.78350022345642));
#91439=CARTESIAN_POINT('Ctrl Pts',(-9.74895798087205,3.85508507402917,-1.53002367048987));
#91440=CARTESIAN_POINT('Ctrl Pts',(-9.68301864972635,3.93237080570732,-0.234609202223619));
#91441=CARTESIAN_POINT('Ctrl Pts',(-9.61707931858065,4.00965653738547,1.06080526604262));
#91442=CARTESIAN_POINT('Ctrl Pts',(-9.55113998743494,3.38400550352473,2.39815764960857));
#91443=CARTESIAN_POINT('Ctrl Pts',(-9.48520065628923,2.34005455335575,3.16902608362037));
#91444=CARTESIAN_POINT('Ctrl Pts',(-9.41926132514353,1.29610360318675,3.93989451763218));
#91445=CARTESIAN_POINT('Ctrl Pts',(-9.35332199399783,-0.166147263290487,
4.14427900208985));
#91446=CARTESIAN_POINT('Ctrl Pts',(-9.28738266285213,-1.3814542330026,3.6891958247654));
#91447=CARTESIAN_POINT('Ctrl Pts',(-9.22144333170643,-2.59676120271469,
3.23411264744095));
#91448=CARTESIAN_POINT('Ctrl Pts',(-9.15550400056072,-3.56512427566165,
2.11956180833439));
#91449=CARTESIAN_POINT('Ctrl Pts',(-9.08956466941502,-3.84599145228225,
0.852602709542451));
#91450=CARTESIAN_POINT('Ctrl Pts',(-9.07509762028834,-3.90761353991406,
0.574632654262041));
#91451=CARTESIAN_POINT('Ctrl Pts',(-9.06063057116165,-3.93614226116156,
0.289326260823524));
#91452=CARTESIAN_POINT('Ctrl Pts',(-9.04616352203496,-3.93353134025131,
0.00350314687873205));
#91453=CARTESIAN_POINT('Origin',(-14.6,0.,0.));
#91454=CARTESIAN_POINT('',(-7.61283647796501,-3.92679881921828,-0.000798651706886422));
#91455=CARTESIAN_POINT('',(-7.79616352203497,-3.92680118028447,-0.000805323033976586));
#91456=CARTESIAN_POINT('',(-14.6,-3.933,-4.81653586104654E-16));
#91457=CARTESIAN_POINT('Ctrl Pts',(-7.61283647796501,-3.92679881921828,
-0.000798651706886422));
#91458=CARTESIAN_POINT('Ctrl Pts',(-7.64831290436767,-3.92551283842261,
0.703147926407711));
#91459=CARTESIAN_POINT('Ctrl Pts',(-7.68378933077033,-3.74491780739553,
1.40771013463382));
#91460=CARTESIAN_POINT('Ctrl Pts',(-7.71926575717298,-3.38896710896084,
2.00835388494562));
#91461=CARTESIAN_POINT('Ctrl Pts',(-7.78520508831869,-2.72736859536671,
3.12475852792963));
#91462=CARTESIAN_POINT('Ctrl Pts',(-7.85114441946439,-1.45997024859465,
3.88215689869411));
#91463=CARTESIAN_POINT('Ctrl Pts',(-7.91708375061009,-0.163368689798379,
3.93597434747573));
#91464=CARTESIAN_POINT('Ctrl Pts',(-7.98302308175579,1.1332328689979,3.98979179625734));
#91465=CARTESIAN_POINT('Ctrl Pts',(-8.04896241290149,2.45903763981833,3.34002832305605));
#91466=CARTESIAN_POINT('Ctrl Pts',(-8.11490174404719,3.21087728722124,2.2822906123455));
#91467=CARTESIAN_POINT('Ctrl Pts',(-8.1808410751929,3.96271693462414,1.22455290163496));
#91468=CARTESIAN_POINT('Ctrl Pts',(-8.24678040633861,4.14059145860952,-0.241159046584857));
#91469=CARTESIAN_POINT('Ctrl Pts',(-8.31271973748431,3.66357772259559,-1.44802681718783));
#91470=CARTESIAN_POINT('Ctrl Pts',(-8.37865906863001,3.18656398658166,-2.6548945877908));
#91471=CARTESIAN_POINT('Ctrl Pts',(-8.44459839977571,2.05466199056844,-3.60291818077695));
#91472=CARTESIAN_POINT('Ctrl Pts',(-8.51053773092141,0.782824959830684,
-3.86079894258426));
#91473=CARTESIAN_POINT('Ctrl Pts',(-8.57647706206711,-0.489012070907112,
-4.11867970439156));
#91474=CARTESIAN_POINT('Ctrl Pts',(-8.64241639321282,-1.90078413636944,
-3.68641763501997));
#91475=CARTESIAN_POINT('Ctrl Pts',(-8.70835572435852,-2.81021250480815,
-2.76066822900065));
#91476=CARTESIAN_POINT('Ctrl Pts',(-8.75984930889402,-3.52040664471687,
-2.03772860451146));
#91477=CARTESIAN_POINT('Ctrl Pts',(-8.81134289342952,-3.92425061036948,
-1.01383978434024));
#91478=CARTESIAN_POINT('Ctrl Pts',(-8.86283647796501,-3.93354422253028,
0.0035021652868221));
#91479=CARTESIAN_POINT('Ctrl Pts',(-9.04616352203496,-3.93353134025131,
0.00350314687873205));
#91480=CARTESIAN_POINT('Ctrl Pts',(-8.99469124001595,-3.92424195053232,
-1.01342627664713));
#91481=CARTESIAN_POINT('Ctrl Pts',(-8.94321895799693,-3.52076714574602,
-2.03689667730455));
#91482=CARTESIAN_POINT('Ctrl Pts',(-8.89174667597791,-2.81109902180865,
-2.75976519307961));
#91483=CARTESIAN_POINT('Ctrl Pts',(-8.82580734483221,-1.90196813442025,
-3.68580663843232));
#91484=CARTESIAN_POINT('Ctrl Pts',(-8.75986801368651,-0.490335079349264,
-4.11852217066041));
#91485=CARTESIAN_POINT('Ctrl Pts',(-8.69392868254081,0.781584653747444,
-3.86104999454471));
#91486=CARTESIAN_POINT('Ctrl Pts',(-8.6279893513951,2.05350438684415,-3.60357781842901));
#91487=CARTESIAN_POINT('Ctrl Pts',(-8.5620500202494,3.18571079796658,-2.65591793396953));
#91488=CARTESIAN_POINT('Ctrl Pts',(-8.4961106891037,3.66311216968885,-1.44920352732965));
#91489=CARTESIAN_POINT('Ctrl Pts',(-8.430171357958,4.14051354141113,-0.242489120689763));
#91490=CARTESIAN_POINT('Ctrl Pts',(-8.36423202681229,3.96310987373324,1.22327980813051));
#91491=CARTESIAN_POINT('Ctrl Pts',(-8.29829269566659,3.21161008948428,2.28125892096229));
#91492=CARTESIAN_POINT('Ctrl Pts',(-8.23235336452089,2.46011030523531,3.33923803379406));
#91493=CARTESIAN_POINT('Ctrl Pts',(-8.16641403337519,1.13451440441526,3.98942733063732));
#91494=CARTESIAN_POINT('Ctrl Pts',(-8.10047470222949,-0.16210430190959,
3.93602640065455));
#91495=CARTESIAN_POINT('Ctrl Pts',(-8.03453537108379,-1.45872300823444,
3.88262547067178));
#91496=CARTESIAN_POINT('Ctrl Pts',(-7.96859603993807,-2.7263645200641,3.12563431386297));
#91497=CARTESIAN_POINT('Ctrl Pts',(-7.90265670879237,-3.38832158950249,
2.00944232001286));
#91498=CARTESIAN_POINT('Ctrl Pts',(-7.86715897987324,-3.74467905019782,
1.4085523787447));
#91499=CARTESIAN_POINT('Ctrl Pts',(-7.8316612509541,-3.92550363005813,0.703562755676425));
#91500=CARTESIAN_POINT('Ctrl Pts',(-7.79616352203497,-3.92680118028447,
-0.000805323033976586));
#91501=CARTESIAN_POINT('Origin',(-14.6,0.,0.));
#91502=CARTESIAN_POINT('',(-6.36283647796501,-3.93641844162456,-0.00287374819983588));
#91503=CARTESIAN_POINT('',(-6.54616352203497,-3.93642949564762,-0.0028694466954664));
#91504=CARTESIAN_POINT('',(-14.6,-3.933,-4.81653586104654E-16));
#91505=CARTESIAN_POINT('Ctrl Pts',(-6.36283647796501,-3.93641844162456,
-0.00287374819983588));
#91506=CARTESIAN_POINT('Ctrl Pts',(-6.41934358416012,-3.92725780126381,
1.11141212263338));
#91507=CARTESIAN_POINT('Ctrl Pts',(-6.47585069035523,-3.43070555928188,
2.23284140174591));
#91508=CARTESIAN_POINT('Ctrl Pts',(-6.53235779655034,-2.59367156922317,
2.96503814205455));
#91509=CARTESIAN_POINT('Ctrl Pts',(-6.59829712769604,-1.616918994775,3.81945392396189));
#91510=CARTESIAN_POINT('Ctrl Pts',(-6.66423645884175,-0.176530818837051,
4.14384992282044));
#91511=CARTESIAN_POINT('Ctrl Pts',(-6.73017578998745,1.07219546863473,3.79064378039207));
#91512=CARTESIAN_POINT('Ctrl Pts',(-6.79611512113315,2.32092175610655,3.43743763796369));
#91513=CARTESIAN_POINT('Ctrl Pts',(-6.86205445227885,3.37798615511219,2.40662935424836));
#91514=CARTESIAN_POINT('Ctrl Pts',(-6.92799378342455,3.76248243569573,1.16718006917013));
#91515=CARTESIAN_POINT('Ctrl Pts',(-6.99393311457025,4.14697871627925,-0.0722692159080598));
#91516=CARTESIAN_POINT('Ctrl Pts',(-7.05987244571596,3.85890687844073,-1.52035950234914));
#91517=CARTESIAN_POINT('Ctrl Pts',(-7.12581177686166,3.02932378268899,-2.51828926305827));
#91518=CARTESIAN_POINT('Ctrl Pts',(-7.19175110800737,2.19974068693724,-3.51621902376742));
#91519=CARTESIAN_POINT('Ctrl Pts',(-7.25769043915306,0.828646333272257,
-4.06398825874461));
#91520=CARTESIAN_POINT('Ctrl Pts',(-7.32362977029876,-0.46018667072598,
-3.91239205868715));
#91521=CARTESIAN_POINT('Ctrl Pts',(-7.38956910144447,-1.74901967472424,
-3.76079585862969));
#91522=CARTESIAN_POINT('Ctrl Pts',(-7.45550843259018,-2.95559132905574,
-2.90983422353755));
#91523=CARTESIAN_POINT('Ctrl Pts',(-7.52144776373588,-3.53097781601342,
-1.74664794838972));
#91524=CARTESIAN_POINT('Ctrl Pts',(-7.55191066847893,-3.7967970689248,-1.209274698122));
#91525=CARTESIAN_POINT('Ctrl Pts',(-7.58237357322197,-3.92790306545872,
-0.605263636705807));
#91526=CARTESIAN_POINT('Ctrl Pts',(-7.61283647796501,-3.92679881921828,
-0.000798651706886422));
#91527=CARTESIAN_POINT('Ctrl Pts',(-7.79616352203497,-3.92680118028447,
-0.000805323033976586));
#91528=CARTESIAN_POINT('Ctrl Pts',(-7.7657219198084,-3.92791391366382,-0.604846582181445));
#91529=CARTESIAN_POINT('Ctrl Pts',(-7.73528031758184,-3.79699935314037,
-1.2084307468191));
#91530=CARTESIAN_POINT('Ctrl Pts',(-7.70483871535528,-3.5315385167675,-1.74551348775504));
#91531=CARTESIAN_POINT('Ctrl Pts',(-7.63889938420957,-2.95652574754698,
-2.90888447078147));
#91532=CARTESIAN_POINT('Ctrl Pts',(-7.57296005306386,-1.75022758205879,
-3.76023360594288));
#91533=CARTESIAN_POINT('Ctrl Pts',(-7.50702072191815,-0.461443415611824,
-3.91224380701605));
#91534=CARTESIAN_POINT('Ctrl Pts',(-7.44108139077245,0.827340750835101,
-4.06425400808922));
#91535=CARTESIAN_POINT('Ctrl Pts',(-7.37514205962676,2.1986109182408,-3.5169252750742));
#91536=CARTESIAN_POINT('Ctrl Pts',(-7.30920272848106,3.02851449343374,-2.5192621130819));
#91537=CARTESIAN_POINT('Ctrl Pts',(-7.24326339733536,3.85841806862672,-1.52159895108955));
#91538=CARTESIAN_POINT('Ctrl Pts',(-7.17732406618965,4.1469550516069,-0.0736013601199095));
#91539=CARTESIAN_POINT('Ctrl Pts',(-7.11138473504394,3.76285696637598,1.16597130408181));
#91540=CARTESIAN_POINT('Ctrl Pts',(-7.04544540389824,3.37875888114507,2.40554396828349));
#91541=CARTESIAN_POINT('Ctrl Pts',(-6.97950607275254,2.32202572770306,3.43669170571723));
#91542=CARTESIAN_POINT('Ctrl Pts',(-6.91356674160684,1.07341303747873,3.79029894366082));
#91543=CARTESIAN_POINT('Ctrl Pts',(-6.84762741046114,-0.175199652745603,
4.14390618160442));
#91544=CARTESIAN_POINT('Ctrl Pts',(-6.78168807931544,-1.61569187975229,
3.81997292005788));
#91545=CARTESIAN_POINT('Ctrl Pts',(-6.71574874816973,-2.59271881607825,
2.96587099721264));
#91546=CARTESIAN_POINT('Ctrl Pts',(-6.65922033945814,-3.43030356283321,
2.23366729212402));
#91547=CARTESIAN_POINT('Ctrl Pts',(-6.60269193074656,-3.92727496395024,
1.11182810600055));
#91548=CARTESIAN_POINT('Ctrl Pts',(-6.54616352203497,-3.93642949564762,
-0.0028694466954664));
#91549=CARTESIAN_POINT('Origin',(-14.6,0.,0.));
#91550=CARTESIAN_POINT('',(-5.11283647796501,-3.93521788455812,0.00324097164884296));
#91551=CARTESIAN_POINT('',(-5.29616352203496,-3.93520542350542,0.00324387462324732));
#91552=CARTESIAN_POINT('',(-14.6,-3.933,-4.81653586104654E-16));
#91553=CARTESIAN_POINT('Ctrl Pts',(-5.11283647796501,-3.93521788455812,
0.00324097164884296));
#91554=CARTESIAN_POINT('Ctrl Pts',(-5.12443493280686,-3.937249357363,0.23213678076217));
#91555=CARTESIAN_POINT('Ctrl Pts',(-5.13603338764872,-3.91898391613797,
0.460708744038742));
#91556=CARTESIAN_POINT('Ctrl Pts',(-5.14763184249057,-3.87926378197342,
0.685489532446667));
#91557=CARTESIAN_POINT('Ctrl Pts',(-5.21357117363628,-3.65344757494068,
1.96340931091013));
#91558=CARTESIAN_POINT('Ctrl Pts',(-5.27951050478199,-2.73418782810802,
3.11879339388157));
#91559=CARTESIAN_POINT('Ctrl Pts',(-5.3454498359277,-1.53969722382919,3.62600549551672));
#91560=CARTESIAN_POINT('Ctrl Pts',(-5.4113891670734,-0.345206619550455,
4.13321759715182));
#91561=CARTESIAN_POINT('Ctrl Pts',(-5.47732849821909,1.12451484217442,3.99225771745075));
#91562=CARTESIAN_POINT('Ctrl Pts',(-5.54326782936479,2.20082463711376,3.26725485835136));
#91563=CARTESIAN_POINT('Ctrl Pts',(-5.60920716051049,3.27713443205317,2.54225199925191));
#91564=CARTESIAN_POINT('Ctrl Pts',(-5.6751464916562,3.96003256020699,1.2332061607541));
#91565=CARTESIAN_POINT('Ctrl Pts',(-5.74108582280191,3.93883788978656,-0.0643387155085294));
#91566=CARTESIAN_POINT('Ctrl Pts',(-5.80702515394761,3.91764321936612,-1.3618835917711));
#91567=CARTESIAN_POINT('Ctrl Pts',(-5.87296448509331,3.19235575037146,-2.64792750579845));
#91568=CARTESIAN_POINT('Ctrl Pts',(-5.93890381623901,2.09294143612736,-3.33739112751421));
#91569=CARTESIAN_POINT('Ctrl Pts',(-6.00484314738471,0.993527121883229,
-4.02685474922998));
#91570=CARTESIAN_POINT('Ctrl Pts',(-6.07078247853041,-0.480014037610387,
-4.11973807863413));
#91571=CARTESIAN_POINT('Ctrl Pts',(-6.13672180967612,-1.65730176610455,
-3.57378430362403));
#91572=CARTESIAN_POINT('Ctrl Pts',(-6.20266114082182,-2.83458949459872,
-3.02783052861393));
#91573=CARTESIAN_POINT('Ctrl Pts',(-6.26860047196753,-3.71562379209344,
-1.84303964918957));
#91574=CARTESIAN_POINT('Ctrl Pts',(-6.33453980311323,-3.89958245436161,
-0.55842642699929));
#91575=CARTESIAN_POINT('Ctrl Pts',(-6.34397202806382,-3.92589663519989,
-0.374670227540233));
#91576=CARTESIAN_POINT('Ctrl Pts',(-6.35340425301442,-3.93794754524342,
-0.188871504954147));
#91577=CARTESIAN_POINT('Ctrl Pts',(-6.36283647796501,-3.93641844162456,
-0.00287374819983588));
#91578=CARTESIAN_POINT('Ctrl Pts',(-6.54616352203497,-3.93642949564762,
-0.0028694466954664));
#91579=CARTESIAN_POINT('Ctrl Pts',(-6.53675259960086,-3.93795355389883,
-0.188445733822925));
#91580=CARTESIAN_POINT('Ctrl Pts',(-6.52734167716674,-3.92595726999319,
-0.373824083294776));
#91581=CARTESIAN_POINT('Ctrl Pts',(-6.51793075473263,-3.89976141760876,
-0.557173686627855));
#91582=CARTESIAN_POINT('Ctrl Pts',(-6.45199142358692,-3.71621543716804,
-1.84184586347916));
#91583=CARTESIAN_POINT('Ctrl Pts',(-6.38605209244122,-2.83556183064135,
-3.02691963303782));
#91584=CARTESIAN_POINT('Ctrl Pts',(-6.32011276129552,-1.65844960882676,
-3.5732515341523));
#91585=CARTESIAN_POINT('Ctrl Pts',(-6.25417343014981,-0.481337387012155,
-4.1195834352668));
#91586=CARTESIAN_POINT('Ctrl Pts',(-6.18823409900411,0.992233450090349,
-4.02717346793708));
#91587=CARTESIAN_POINT('Ctrl Pts',(-6.12229476785841,2.09186912464122,-3.33806309059033));
#91588=CARTESIAN_POINT('Ctrl Pts',(-6.05635543671271,3.1915047991921,-2.64895271324358));
#91589=CARTESIAN_POINT('Ctrl Pts',(-5.990416105567,3.91720531119132,-1.3631419258798));
#91590=CARTESIAN_POINT('Ctrl Pts',(-5.9244767744213,3.93881679526393,-0.0656039986291013));
#91591=CARTESIAN_POINT('Ctrl Pts',(-5.85853744327559,3.96042827933653,1.23193392862154));
#91592=CARTESIAN_POINT('Ctrl Pts',(-5.79259811212989,3.27795073548254,2.54119899575913));
#91593=CARTESIAN_POINT('Ctrl Pts',(-5.72665878098419,2.20187395307353,3.26654752392988));
#91594=CARTESIAN_POINT('Ctrl Pts',(-5.66071944983849,1.12579717066446,3.99189605210066));
#91595=CARTESIAN_POINT('Ctrl Pts',(-5.59478011869279,-0.34387885029961,
4.13332804130459));
#91596=CARTESIAN_POINT('Ctrl Pts',(-5.52884078754709,-1.53853225927603,
3.6264997061618));
#91597=CARTESIAN_POINT('Ctrl Pts',(-5.46290145640139,-2.73318566825241,
3.11967137101902));
#91598=CARTESIAN_POINT('Ctrl Pts',(-5.39696212525568,-3.65281646524112,
1.96458271152948));
#91599=CARTESIAN_POINT('Ctrl Pts',(-5.33102279410998,-3.8790431592278,0.686735611229462));
#91600=CARTESIAN_POINT('Ctrl Pts',(-5.31940303675164,-3.91890858167644,
0.461554782298517));
#91601=CARTESIAN_POINT('Ctrl Pts',(-5.3077832793933,-3.93724165312964,0.232561922513211));
#91602=CARTESIAN_POINT('Ctrl Pts',(-5.29616352203496,-3.93520542350542,
0.00324387462324732));
#91603=CARTESIAN_POINT('Origin',(-14.6,0.,0.));
#91604=CARTESIAN_POINT('',(-3.86283647796501,-3.9266497763299,0.000109410655622921));
#91605=CARTESIAN_POINT('',(-4.04616352203497,-3.92664918805101,0.000102552286748496));
#91606=CARTESIAN_POINT('',(-14.6,-3.933,-4.81653586104654E-16));
#91607=CARTESIAN_POINT('Ctrl Pts',(-3.86283647796501,-3.9266497763299,0.000109410655622921));
#91608=CARTESIAN_POINT('Ctrl Pts',(-3.89546561259932,-3.92681141280058,
0.647619536085308));
#91609=CARTESIAN_POINT('Ctrl Pts',(-3.92809474723363,-3.77541687798498,
1.29505849841556));
#91610=CARTESIAN_POINT('Ctrl Pts',(-3.96072388186793,-3.47204825468472,
1.86103845086822));
#91611=CARTESIAN_POINT('Ctrl Pts',(-4.02666321301364,-2.858978851061,3.00481195037645));
#91612=CARTESIAN_POINT('Ctrl Pts',(-4.09260254415934,-1.62525837440169,
3.81591280553418));
#91613=CARTESIAN_POINT('Ctrl Pts',(-4.15854187530505,-0.332161796206972,
3.92533463561106));
#91614=CARTESIAN_POINT('Ctrl Pts',(-4.22448120645075,0.960934781987714,
4.03475646568794));
#91615=CARTESIAN_POINT('Ctrl Pts',(-4.29042053759645,2.31340746171779,3.44249927068401));
#91616=CARTESIAN_POINT('Ctrl Pts',(-4.35635986874215,3.10995543804893,2.41800756422801));
#91617=CARTESIAN_POINT('Ctrl Pts',(-4.42229919988785,3.90650341438011,1.39351585777196));
#91618=CARTESIAN_POINT('Ctrl Pts',(-4.48823853103356,4.14712668731228,-0.0632103601362513));
#91619=CARTESIAN_POINT('Ctrl Pts',(-4.55417786217927,3.72235490549252,-1.28944070187289));
#91620=CARTESIAN_POINT('Ctrl Pts',(-4.62011719332497,3.29758312367278,-2.51567104360945));
#91621=CARTESIAN_POINT('Ctrl Pts',(-4.68605652447066,2.20741628710125,-3.51140550917451));
#91622=CARTESIAN_POINT('Ctrl Pts',(-4.75199585561636,0.947820406481901,
-3.82363961182173));
#91623=CARTESIAN_POINT('Ctrl Pts',(-4.81793518676207,-0.311775474137514,
-4.13587371446897));
#91624=CARTESIAN_POINT('Ctrl Pts',(-4.88387451790777,-1.74080039880474,
-3.76460745419828));
#91625=CARTESIAN_POINT('Ctrl Pts',(-4.94981384905348,-2.68912652752191,
-2.8787465870852));
#91626=CARTESIAN_POINT('Ctrl Pts',(-5.00415472535732,-3.47064602371538,
-2.1487049720764));
#91627=CARTESIAN_POINT('Ctrl Pts',(-5.05849560166116,-3.92570006395965,
-1.06917764092437));
#91628=CARTESIAN_POINT('Ctrl Pts',(-5.11283647796501,-3.93521788455812,
0.00324097164884296));
#91629=CARTESIAN_POINT('Ctrl Pts',(-5.29616352203496,-3.93520542350542,
0.00324387462324732));
#91630=CARTESIAN_POINT('Ctrl Pts',(-5.2418439482476,-3.92568653925424,-1.06876290133542));
#91631=CARTESIAN_POINT('Ctrl Pts',(-5.18752437446023,-3.47102960783475,
-2.14787613604391));
#91632=CARTESIAN_POINT('Ctrl Pts',(-5.13320480067287,-2.69005098778536,
-2.87788243582242));
#91633=CARTESIAN_POINT('Ctrl Pts',(-5.06726546952716,-1.74200953137151,
-3.76404784146379));
#91634=CARTESIAN_POINT('Ctrl Pts',(-5.00132613838146,-0.313104027559104,
-4.13577311163589));
#91635=CARTESIAN_POINT('Ctrl Pts',(-4.93538680723576,0.946592018069592,
-3.82394366910327));
#91636=CARTESIAN_POINT('Ctrl Pts',(-4.86944747609006,2.20628806369818,-3.51211422657067));
#91637=CARTESIAN_POINT('Ctrl Pts',(-4.80350814494435,3.29677465114311,-2.51673007133348));
#91638=CARTESIAN_POINT('Ctrl Pts',(-4.73756881379865,3.72194029202664,-1.29063631219266));
#91639=CARTESIAN_POINT('Ctrl Pts',(-4.67162948265295,4.1471059329102,-0.0645425530517454));
#91640=CARTESIAN_POINT('Ctrl Pts',(-4.60569015150725,3.90695062723229,1.3922608099928));
#91641=CARTESIAN_POINT('Ctrl Pts',(-4.53975082036155,3.11073184340648,2.41700828104648));
#91642=CARTESIAN_POINT('Ctrl Pts',(-4.47381148921585,2.31451305958069,3.44175575210011));
#91643=CARTESIAN_POINT('Ctrl Pts',(-4.40787215807014,0.962230797607039,
4.03444733116288));
#91644=CARTESIAN_POINT('Ctrl Pts',(-4.34193282692444,-0.330900798702454,
3.92544090568989));
#91645=CARTESIAN_POINT('Ctrl Pts',(-4.27599349577874,-1.62403239501198,
3.8164344802169));
#91646=CARTESIAN_POINT('Ctrl Pts',(-4.21005416463304,-2.85801332565737,
3.00573005020813));
#91647=CARTESIAN_POINT('Ctrl Pts',(-4.14411483348733,-3.4714500665587,1.86215360266608));
#91648=CARTESIAN_POINT('Ctrl Pts',(-4.11146439633654,-3.77519863978166,
1.29590171204423));
#91649=CARTESIAN_POINT('Ctrl Pts',(-4.07881395918575,-3.92680082759742,
0.648035530114968));
#91650=CARTESIAN_POINT('Ctrl Pts',(-4.04616352203497,-3.92664918805101,
0.000102552286748496));
#91651=CARTESIAN_POINT('Origin',(-14.6,0.,0.));
#91652=CARTESIAN_POINT('',(-2.61283647796502,-3.93482597683023,-0.00332506251532583));
#91653=CARTESIAN_POINT('',(-2.79616352203497,-3.93483613066414,-0.00332402043238414));
#91654=CARTESIAN_POINT('',(-14.6,-3.933,-4.81653586104654E-16));
#91655=CARTESIAN_POINT('Ctrl Pts',(-2.61283647796502,-3.93482597683023,
-0.00332506251532583));
#91656=CARTESIAN_POINT('Ctrl Pts',(-2.66649629239178,-3.92529592795581,
1.05592713778507));
#91657=CARTESIAN_POINT('Ctrl Pts',(-2.72015610681853,-3.48282948623788,
2.12219777834594));
#91658=CARTESIAN_POINT('Ctrl Pts',(-2.77381592124529,-2.718548420221,2.85097673606072));
#91659=CARTESIAN_POINT('Ctrl Pts',(-2.83975525239099,-1.77936920689613,
3.74652953545347));
#91660=CARTESIAN_POINT('Ctrl Pts',(-2.9056945835367,-0.354234475111307,
4.13245370603341));
#91661=CARTESIAN_POINT('Ctrl Pts',(-2.97163391468241,0.90850115995116,3.83317244788512));
#91662=CARTESIAN_POINT('Ctrl Pts',(-3.03757324582811,2.17123679501352,3.53389118973686));
#91663=CARTESIAN_POINT('Ctrl Pts',(-3.1035125769738,3.27157333335356,2.5494045028605));
#91664=CARTESIAN_POINT('Ctrl Pts',(-3.1694519081195,3.70891632543792,1.32760105294568));
#91665=CARTESIAN_POINT('Ctrl Pts',(-3.23539123926521,4.1462593175223,0.10579760303079));
#91666=CARTESIAN_POINT('Ctrl Pts',(-3.30133057041091,3.92060876335093,-1.35332260992259));
#91667=CARTESIAN_POINT('Ctrl Pts',(-3.36726990155662,3.13462419475558,-2.38594073109377));
#91668=CARTESIAN_POINT('Ctrl Pts',(-3.43320923270232,2.34863962616026,-3.41855885226493));
#91669=CARTESIAN_POINT('Ctrl Pts',(-3.49914856384802,1.00232104314098,-4.02467488165392));
#91670=CARTESIAN_POINT('Ctrl Pts',(-3.56508789499372,-0.291831044969713,
-3.92853896723417));
#91671=CARTESIAN_POINT('Ctrl Pts',(-3.63102722613942,-1.58598313308048,
-3.83240305281441));
#91672=CARTESIAN_POINT('Ctrl Pts',(-3.69696655728513,-2.82796872628265,
-3.03401519458584));
#91673=CARTESIAN_POINT('Ctrl Pts',(-3.76290588843083,-3.45275235758963,
-1.89659819354216));
#91674=CARTESIAN_POINT('Ctrl Pts',(-3.79621608494223,-3.76837074762076,
-1.32201572262741));
#91675=CARTESIAN_POINT('Ctrl Pts',(-3.82952628145362,-3.92648476605112,
-0.660916073560029));
#91676=CARTESIAN_POINT('Ctrl Pts',(-3.86283647796501,-3.9266497763299,0.000109410655622921));
#91677=CARTESIAN_POINT('Ctrl Pts',(-4.04616352203497,-3.92664918805101,
0.000102552286748496));
#91678=CARTESIAN_POINT('Ctrl Pts',(-4.01287462804005,-3.92649458329757,
-0.660500309326387));
#91679=CARTESIAN_POINT('Ctrl Pts',(-3.97958573404514,-3.76859324143987,
-1.32117260467504));
#91680=CARTESIAN_POINT('Ctrl Pts',(-3.94629684005023,-3.45336120237453,
-1.8954888688236));
#91681=CARTESIAN_POINT('Ctrl Pts',(-3.88035750890452,-2.82894304613174,
-3.033106427696));
#91682=CARTESIAN_POINT('Ctrl Pts',(-3.81441817775881,-1.58721418248879,
-3.83189308036553));
#91683=CARTESIAN_POINT('Ctrl Pts',(-3.74847884661311,-0.293093059405651,
-3.92844475050617));
#91684=CARTESIAN_POINT('Ctrl Pts',(-3.68253951546741,1.00102806367751,-4.02499642064681));
#91685=CARTESIAN_POINT('Ctrl Pts',(-3.61660018432172,2.34754144620083,-3.41931310825863));
#91686=CARTESIAN_POINT('Ctrl Pts',(-3.55066085317602,3.13385753223803,-2.38694750757919));
#91687=CARTESIAN_POINT('Ctrl Pts',(-3.48472152203031,3.92017361827524,-1.35458190689974));
#91688=CARTESIAN_POINT('Ctrl Pts',(-3.4187821908846,4.14629240782621,0.104465982070971));
#91689=CARTESIAN_POINT('Ctrl Pts',(-3.3528428597389,3.70934215864998,1.3264096424498));
#91690=CARTESIAN_POINT('Ctrl Pts',(-3.28690352859319,3.27239190947374,2.54835330282863));
#91691=CARTESIAN_POINT('Ctrl Pts',(-3.2209641974475,2.1723726215703,3.53319273461559));
#91692=CARTESIAN_POINT('Ctrl Pts',(-3.15502486630179,0.909732860103698,
3.83287987540983));
#91693=CARTESIAN_POINT('Ctrl Pts',(-3.08908553515609,-0.35290690136287,
4.13256701620405));
#91694=CARTESIAN_POINT('Ctrl Pts',(-3.02314620401039,-1.77816713639261,
3.74710186600559));
#91695=CARTESIAN_POINT('Ctrl Pts',(-2.95720687286468,-2.71763315930033,
2.85185032219934));
#91696=CARTESIAN_POINT('Ctrl Pts',(-2.90352575592145,-3.48245113005701,
2.12302729682641));
#91697=CARTESIAN_POINT('Ctrl Pts',(-2.84984463897821,-3.92530581696798,
1.05634001278133));
#91698=CARTESIAN_POINT('Ctrl Pts',(-2.79616352203497,-3.93483613066414,
-0.00332402043238414));
#91699=CARTESIAN_POINT('Origin',(-14.6,0.,0.));
#91700=CARTESIAN_POINT('',(-1.36283647796502,-3.93682057842306,0.00276514463350926));
#91701=CARTESIAN_POINT('',(-1.54616352203498,-3.93676751258924,0.00274060645320142));
#91702=CARTESIAN_POINT('',(-14.6,-3.933,-4.81653586104654E-16));
#91703=CARTESIAN_POINT('Ctrl Pts',(-1.36283647796502,-3.93682057842306,
0.00276514463350926));
#91704=CARTESIAN_POINT('Ctrl Pts',(-1.37158764103853,-3.93820694651525,
0.175305934189915));
#91705=CARTESIAN_POINT('Ctrl Pts',(-1.38033880411203,-3.92785596749255,
0.347679209261104));
#91706=CARTESIAN_POINT('Ctrl Pts',(-1.38908996718554,-3.90520506174835,
0.518417021592109));
#91707=CARTESIAN_POINT('Ctrl Pts',(-1.45502929833124,-3.73453225379453,
1.8049131195188));
#91708=CARTESIAN_POINT('Ctrl Pts',(-1.52096862947694,-2.86553049728958,
2.99855573940384));
#91709=CARTESIAN_POINT('Ctrl Pts',(-1.58690796062265,-1.69386838589715,
3.55653944458954));
#91710=CARTESIAN_POINT('Ctrl Pts',(-1.65284729176835,-0.522206274504723,
4.11452314977523));
#91711=CARTESIAN_POINT('Ctrl Pts',(-1.71878662291405,0.952116191775279,
4.03684794026153));
#91712=CARTESIAN_POINT('Ctrl Pts',(-1.78472595405975,2.05853064267987,3.35872836780381));
#91713=CARTESIAN_POINT('Ctrl Pts',(-1.85066528520546,3.16494509358447,2.6806087953461));
#91714=CARTESIAN_POINT('Ctrl Pts',(-1.91660461635116,3.90345152911377,1.40204485994436));
#91715=CARTESIAN_POINT('Ctrl Pts',(-1.98254394749686,3.93798269334203,0.104777353878543));
#91716=CARTESIAN_POINT('Ctrl Pts',(-2.04848327864256,3.9725138575703,-1.19249015218735));
#91717=CARTESIAN_POINT('Ctrl Pts',(-2.11442260978827,3.30306975049746,-2.50846122891732));
#91718=CARTESIAN_POINT('Ctrl Pts',(-2.18036194093398,2.2342563079641,-3.24447498598491));
#91719=CARTESIAN_POINT('Ctrl Pts',(-2.24630127207968,1.16544286543083,-3.98048874305243));
#91720=CARTESIAN_POINT('Ctrl Pts',(-2.31224060322537,-0.30273991256285,
-4.13654518045766));
#91721=CARTESIAN_POINT('Ctrl Pts',(-2.37817993437107,-1.50237335701287,
-3.64162961614031));
#91722=CARTESIAN_POINT('Ctrl Pts',(-2.44411926551678,-2.70200680146297,
-3.14671405182294));
#91723=CARTESIAN_POINT('Ctrl Pts',(-2.51005859666248,-3.63309091236934,
-2.00082648578291));
#91724=CARTESIAN_POINT('Ctrl Pts',(-2.57599792780818,-3.87202112039005,
-0.725291988660146));
#91725=CARTESIAN_POINT('Ctrl Pts',(-2.58827744452713,-3.91651577074627,
-0.48775625830218));
#91726=CARTESIAN_POINT('Ctrl Pts',(-2.60055696124607,-3.93700683406457,
-0.245724430499025));
#91727=CARTESIAN_POINT('Ctrl Pts',(-2.61283647796502,-3.93482597683023,
-0.00332506251532583));
#91728=CARTESIAN_POINT('Ctrl Pts',(-2.79616352203497,-3.93483613066414,
-0.00332402043238414));
#91729=CARTESIAN_POINT('Ctrl Pts',(-2.78390530783251,-3.93701240108019,
-0.245300891284708));
#91730=CARTESIAN_POINT('Ctrl Pts',(-2.77164709363004,-3.9165930421361,-0.486911535858293));
#91731=CARTESIAN_POINT('Ctrl Pts',(-2.75938887942757,-3.87225203266108,
-0.724049240203662));
#91732=CARTESIAN_POINT('Ctrl Pts',(-2.69344954828187,-3.63373307232837,
-1.99965932138625));
#91733=CARTESIAN_POINT('Ctrl Pts',(-2.62751021713617,-2.70302334087727,
-3.14584154633738));
#91734=CARTESIAN_POINT('Ctrl Pts',(-2.56157088599047,-1.50354618345133,
-3.64114439342657));
#91735=CARTESIAN_POINT('Ctrl Pts',(-2.49563155484477,-0.304069026025359,
-4.13644724051578));
#91736=CARTESIAN_POINT('Ctrl Pts',(-2.42969222369907,1.16417555737546,-3.98087070974302));
#91737=CARTESIAN_POINT('Ctrl Pts',(-2.36375289255336,2.23321990412611,-3.24519659418834));
#91738=CARTESIAN_POINT('Ctrl Pts',(-2.29781356140766,3.30226425087672,-2.50952247863368));
#91739=CARTESIAN_POINT('Ctrl Pts',(-2.23187423026196,3.97210836097718,-1.19375077829715));
#91740=CARTESIAN_POINT('Ctrl Pts',(-2.16593489911625,3.93800429215139,0.103520445762184));
#91741=CARTESIAN_POINT('Ctrl Pts',(-2.09999556797055,3.90390022332561,1.40079166982155));
#91742=CARTESIAN_POINT('Ctrl Pts',(-2.03405623682485,3.16584797557354,2.67956241760371));
#91743=CARTESIAN_POINT('Ctrl Pts',(-1.96811690567915,2.05963163241508,3.35805118788789));
#91744=CARTESIAN_POINT('Ctrl Pts',(-1.90217757453345,0.953415289256656,
4.03653995817205));
#91745=CARTESIAN_POINT('Ctrl Pts',(-1.83623824338775,-0.520965149308136,
4.11474675095826));
#91746=CARTESIAN_POINT('Ctrl Pts',(-1.77029891224204,-1.69276836578185,
3.5571129497935));
#91747=CARTESIAN_POINT('Ctrl Pts',(-1.70435958109634,-2.8645715822556,2.99947914862873));
#91748=CARTESIAN_POINT('Ctrl Pts',(-1.63842024995063,-3.73379757663826,
1.80600475351295));
#91749=CARTESIAN_POINT('Ctrl Pts',(-1.57248091880493,-3.90495648382779,
0.519614505660644));
#91750=CARTESIAN_POINT('Ctrl Pts',(-1.56370845321495,-3.92772719741634,
0.348475156982074));
#91751=CARTESIAN_POINT('Ctrl Pts',(-1.55493598762496,-3.93814266395565,
0.175691269638936));
#91752=CARTESIAN_POINT('Ctrl Pts',(-1.54616352203498,-3.93676751258924,
0.00274060645320142));
#91753=CARTESIAN_POINT('Origin',(-31.5777734492731,0.,0.));
#91754=CARTESIAN_POINT('',(-0.952773449273097,-3.22588063033637,0.00226579452538821));
#91755=CARTESIAN_POINT('',(-0.7062265507269,-3.21712659271395,0.000156184947003868));
#91756=CARTESIAN_POINT('',(-31.5777734492731,-3.22275,-1.53308031181269E-14));
#91757=CARTESIAN_POINT('',(-0.399999999999999,3.01795629612512,-1.14523995189157));
#91758=CARTESIAN_POINT('Ctrl Pts',(-0.952773449273097,-3.22588063033637,
0.00226579452538841));
#91759=CARTESIAN_POINT('Ctrl Pts',(-0.895585281200896,-3.21845690948414,
-0.921655251058599));
#91760=CARTESIAN_POINT('Ctrl Pts',(-0.772457781982996,-2.31816799471971,
-2.9235001872406));
#91761=CARTESIAN_POINT('Ctrl Pts',(-0.588199965558632,0.985855557350958,
-3.63123937118558));
#91762=CARTESIAN_POINT('Ctrl Pts',(-0.461130317206463,2.66302220805322,
-2.06570245611714));
#91763=CARTESIAN_POINT('Ctrl Pts',(-0.399999999999999,3.01796675574746,
-1.14524144678479));
#91764=CARTESIAN_POINT('',(-0.400000000000005,-0.101608697681796,-3.22114781328883));
#91765=CARTESIAN_POINT('Origin',(-0.4,0.,0.));
#91766=CARTESIAN_POINT('Ctrl Pts',(-0.706226550726901,-3.21712659271395,
0.000156184947003798));
#91767=CARTESIAN_POINT('Ctrl Pts',(-0.670090364963638,-3.21533286770883,
-0.587810425121163));
#91768=CARTESIAN_POINT('Ctrl Pts',(-0.568014848054673,-2.77994359672653,
-2.24993778652945));
#91769=CARTESIAN_POINT('Ctrl Pts',(-0.465939331145708,-1.16924921554908,
-3.18746989196983));
#91770=CARTESIAN_POINT('Ctrl Pts',(-0.400000000000005,-0.101608697681796,
-3.22114781328883));
#91771=CARTESIAN_POINT('Origin',(-31.5777734492731,0.,0.));
#91772=CARTESIAN_POINT('',(-2.20277344927309,-3.22424622853537,-0.00272459832720938));
#91773=CARTESIAN_POINT('',(-1.9562265507269,-3.2258371475202,0.00224568762937409));
#91774=CARTESIAN_POINT('',(-31.5777734492731,-3.22275,-1.53308031181269E-14));
#91775=CARTESIAN_POINT('Ctrl Pts',(-2.20277344927309,-3.22424622853537,
-0.00272459832720937));
#91776=CARTESIAN_POINT('Ctrl Pts',(-2.19049393255415,-3.22603325056741,
-0.201349709735698));
#91777=CARTESIAN_POINT('Ctrl Pts',(-2.1122750846895,-3.11907918299394,-1.4646462045877));
#91778=CARTESIAN_POINT('Ctrl Pts',(-1.96811690567914,-1.45111647622458,
-3.51741211898495));
#91779=CARTESIAN_POINT('Ctrl Pts',(-1.77029891224204,2.15802619942714,-3.13378825655336));
#91780=CARTESIAN_POINT('Ctrl Pts',(-1.57248091880493,3.80367913311811,0.10118183309678));
#91781=CARTESIAN_POINT('Ctrl Pts',(-1.37466292536782,1.98825456019507,3.24419626697628));
#91782=CARTESIAN_POINT('Ctrl Pts',(-1.17684493193072,-1.63598093042552,
3.4351404175943));
#91783=CARTESIAN_POINT('Ctrl Pts',(-1.03621510656581,-3.15462579133896,
1.3491616299952));
#91784=CARTESIAN_POINT('Ctrl Pts',(-0.9615246123466,-3.22701663790542,0.143647902214853));
#91785=CARTESIAN_POINT('Ctrl Pts',(-0.952773449273097,-3.22588063033637,
0.00226579452538841));
#91786=CARTESIAN_POINT('Ctrl Pts',(-1.9562265507269,-3.2258371475202,0.00224568762937397));
#91787=CARTESIAN_POINT('Ctrl Pts',(-1.89905968517118,-3.21849410771212,
-0.921277086382614));
#91788=CARTESIAN_POINT('Ctrl Pts',(-1.77595348846977,-2.31915348223847,
-2.92253791405406));
#91789=CARTESIAN_POINT('Ctrl Pts',(-1.58690796062265,1.07186168277273,-3.65071665635791));
#91790=CARTESIAN_POINT('Ctrl Pts',(-1.38908996718554,3.64542809306271,-1.09141468478898));
#91791=CARTESIAN_POINT('Ctrl Pts',(-1.19127197374844,2.90115349698225,2.46187399806776));
#91792=CARTESIAN_POINT('Ctrl Pts',(-0.993453980311327,-0.481122552182907,
3.77336366075504));
#91793=CARTESIAN_POINT('Ctrl Pts',(-0.831772172637481,-2.89047138994435,
2.04190708737574));
#91794=CARTESIAN_POINT('Ctrl Pts',(-0.736029696109339,-3.21860595878357,
0.485078818306275));
#91795=CARTESIAN_POINT('Ctrl Pts',(-0.706226550726901,-3.21712659271395,
0.000156184947003798));
#91796=CARTESIAN_POINT('Origin',(-31.5777734492731,0.,0.));
#91797=CARTESIAN_POINT('',(-3.45277344927309,-3.21754654631761,8.96524766731527E-5));
#91798=CARTESIAN_POINT('',(-3.20622655072689,-3.22425454871545,-0.00272374443152645));
#91799=CARTESIAN_POINT('',(-31.5777734492731,-3.22275,-1.53308031181269E-14));
#91800=CARTESIAN_POINT('Ctrl Pts',(-3.45277344927309,-3.21754654631761,
8.96524766732035E-5));
#91801=CARTESIAN_POINT('Ctrl Pts',(-3.41946325276169,-3.21741133480582,
-0.541562999253872));
#91802=CARTESIAN_POINT('Ctrl Pts',(-3.32021372510459,-2.8313784513742,-2.15562737063988));
#91803=CARTESIAN_POINT('Ctrl Pts',(-3.15502486630179,-0.281875939904123,
-3.79452870799989));
#91804=CARTESIAN_POINT('Ctrl Pts',(-2.95720687286468,3.02769554249517,-2.30455126046869));
#91805=CARTESIAN_POINT('Ctrl Pts',(-2.75938887942757,3.58239830638208,1.28231347354763));
#91806=CARTESIAN_POINT('Ctrl Pts',(-2.56157088599047,0.877509230153572,
3.70241604420433));
#91807=CARTESIAN_POINT('Ctrl Pts',(-2.37603240927231,-2.40834311719199,
2.81261256561713));
#91808=CARTESIAN_POINT('Ctrl Pts',(-2.25643326369985,-3.21643718581731,
0.865240066945609));
#91809=CARTESIAN_POINT('Ctrl Pts',(-2.20277344927309,-3.22424622853537,
-0.00272459832720937));
#91810=CARTESIAN_POINT('Ctrl Pts',(-3.20622655072689,-3.22425454871545,
-0.00272374443152663));
#91811=CARTESIAN_POINT('Ctrl Pts',(-3.19396833652443,-3.22603781225048,
-0.201002656340778));
#91812=CARTESIAN_POINT('Ctrl Pts',(-3.11577079117626,-3.11930186990163,
-1.46394827087633));
#91813=CARTESIAN_POINT('Ctrl Pts',(-2.9716339146824,-1.45225621275822,-3.51693862418514));
#91814=CARTESIAN_POINT('Ctrl Pts',(-2.7738159212453,2.15703839529281,-3.13449448646742));
#91815=CARTESIAN_POINT('Ctrl Pts',(-2.57599792780818,3.80367463162103,0.0999854885590033));
#91816=CARTESIAN_POINT('Ctrl Pts',(-2.37817993437108,1.98936656034495,3.24350831648798));
#91817=CARTESIAN_POINT('Ctrl Pts',(-2.18036194093398,-1.63501143994855,
3.43575922529938));
#91818=CARTESIAN_POINT('Ctrl Pts',(-2.03971081305258,-3.15427827586105,
1.34975848472338));
#91819=CARTESIAN_POINT('Ctrl Pts',(-1.96499901631689,-3.22696396396214,
0.14396365096069));
#91820=CARTESIAN_POINT('Ctrl Pts',(-1.9562265507269,-3.2258371475202,0.00224568762937397));
#91821=CARTESIAN_POINT('Origin',(-31.5777734492731,0.,0.));
#91822=CARTESIAN_POINT('',(-4.70277344927309,-3.22456736268998,0.00265569320671698));
#91823=CARTESIAN_POINT('',(-4.45622655072689,-3.21754606427445,8.40326422851811E-5));
#91824=CARTESIAN_POINT('',(-31.5777734492731,-3.22275,-1.53308031181269E-14));
#91825=CARTESIAN_POINT('Ctrl Pts',(-4.70277344927309,-3.22456736268998,
0.00265569320671703));
#91826=CARTESIAN_POINT('Ctrl Pts',(-4.64843257296924,-3.21676833997614,
-0.876097696996831));
#91827=CARTESIAN_POINT('Ctrl Pts',(-4.52815236551969,-2.39142780303548,
-2.83405782554972));
#91828=CARTESIAN_POINT('Ctrl Pts',(-4.34193282692443,0.91548834647712,-3.69320756511369));
#91829=CARTESIAN_POINT('Ctrl Pts',(-4.14411483348733,3.59537787550923,-1.24545527762321));
#91830=CARTESIAN_POINT('Ctrl Pts',(-3.94629684005022,3.00386860560673,2.33552444683395));
#91831=CARTESIAN_POINT('Ctrl Pts',(-3.74847884661311,-0.320831111098236,
3.79143358123437));
#91832=CARTESIAN_POINT('Ctrl Pts',(-3.5839710496874,-2.84292582825253,2.13330013806421));
#91833=CARTESIAN_POINT('Ctrl Pts',(-3.48540258390739,-3.21767899328834,
0.530667648085214));
#91834=CARTESIAN_POINT('Ctrl Pts',(-3.45277344927309,-3.21754654631761,
8.96524766732035E-5));
#91835=CARTESIAN_POINT('Ctrl Pts',(-4.45622655072689,-3.21754606427445,
8.40326422848689E-5));
#91836=CARTESIAN_POINT('Ctrl Pts',(-4.42293765673198,-3.21741937918185,
-0.541222316776413));
#91837=CARTESIAN_POINT('Ctrl Pts',(-4.32370943159137,-2.83174183907037,
-2.15492909527557));
#91838=CARTESIAN_POINT('Ctrl Pts',(-4.15854187530505,-0.283095044828532,
-3.79443760733249));
#91839=CARTESIAN_POINT('Ctrl Pts',(-3.96072388186794,3.02695530111143,-2.30552388116989));
#91840=CARTESIAN_POINT('Ctrl Pts',(-3.76290588843083,3.58280909899496,1.28116306328493));
#91841=CARTESIAN_POINT('Ctrl Pts',(-3.56508789499372,0.878699899841087,
3.70213276488018));
#91842=CARTESIAN_POINT('Ctrl Pts',(-3.37952811575908,-2.40781911009861,
2.81328558268817));
#91843=CARTESIAN_POINT('Ctrl Pts',(-3.25990766767013,-3.21644528899918,
0.865578381945218));
#91844=CARTESIAN_POINT('Ctrl Pts',(-3.20622655072689,-3.22425454871545,
-0.00272374443152663));
#91845=CARTESIAN_POINT('Origin',(-31.5777734492731,0.,0.));
#91846=CARTESIAN_POINT('',(-5.95277344927308,-3.22555111435178,-0.00235478566260707));
#91847=CARTESIAN_POINT('',(-5.70622655072688,-3.22455715194561,0.0026580719403356));
#91848=CARTESIAN_POINT('',(-31.5777734492731,-3.22275,-1.53308031181269E-14));
#91849=CARTESIAN_POINT('Ctrl Pts',(-5.95277344927308,-3.22555111435178,
-0.00235478566260758));
#91850=CARTESIAN_POINT('Ctrl Pts',(-5.94334122432249,-3.22680408121872,
-0.154763702667427));
#91851=CARTESIAN_POINT('Ctrl Pts',(-5.86796966822619,-3.14789702397088,
-1.37133825070766));
#91852=CARTESIAN_POINT('Ctrl Pts',(-5.72665878098419,-1.60076786459875,
-3.45187532233801));
#91853=CARTESIAN_POINT('Ctrl Pts',(-5.52884078754708,2.02154698800078,-3.22354599370549));
#91854=CARTESIAN_POINT('Ctrl Pts',(-5.33102279410997,3.80447619524911,-0.0621439922320252));
#91855=CARTESIAN_POINT('Ctrl Pts',(-5.13320480067286,2.12575007586871,3.15580221373199));
#91856=CARTESIAN_POINT('Ctrl Pts',(-4.93538680723576,-1.48717505057987,
3.50231514455317));
#91857=CARTESIAN_POINT('Ctrl Pts',(-4.7919096901025,-3.12617529492704,1.44231545368255));
#91858=CARTESIAN_POINT('Ctrl Pts',(-4.71437190411494,-3.22623197722897,
0.190215817493454));
#91859=CARTESIAN_POINT('Ctrl Pts',(-4.70277344927309,-3.22456736268998,
0.00265569320671703));
#91860=CARTESIAN_POINT('Ctrl Pts',(-5.70622655072688,-3.22455715194561,
0.0026580719403353));
#91861=CARTESIAN_POINT('Ctrl Pts',(-5.65190697693952,-3.21675725766117,
-0.875757854126423));
#91862=CARTESIAN_POINT('Ctrl Pts',(-5.53164807200646,-2.39195967703322,
-2.83338771458464));
#91863=CARTESIAN_POINT('Ctrl Pts',(-5.34544983592769,0.914301858020527,
-3.69350124840367));
#91864=CARTESIAN_POINT('Ctrl Pts',(-5.14763184249059,3.59497741079579,-1.24661010706821));
#91865=CARTESIAN_POINT('Ctrl Pts',(-4.94981384905348,3.00461851577406,2.33455925849379));
#91866=CARTESIAN_POINT('Ctrl Pts',(-4.75199585561637,-0.319613108768782,
3.79153621228826));
#91867=CARTESIAN_POINT('Ctrl Pts',(-4.58746675617418,-2.84256693314919,
2.13399857022515));
#91868=CARTESIAN_POINT('Ctrl Pts',(-4.48887698787768,-3.21767031963884,
0.531008518860414));
#91869=CARTESIAN_POINT('Ctrl Pts',(-4.45622655072689,-3.21754606427445,
8.40326422848689E-5));
#91870=CARTESIAN_POINT('Origin',(-31.5777734492731,0.,0.));
#91871=CARTESIAN_POINT('',(-7.20277344927309,-3.21766867394755,-0.000654425321133341));
#91872=CARTESIAN_POINT('',(-6.95622655072689,-3.22556017215824,-0.00235126095564336));
#91873=CARTESIAN_POINT('',(-31.5777734492731,-3.22275,-1.53308031181269E-14));
#91874=CARTESIAN_POINT('Ctrl Pts',(-7.20277344927309,-3.21766867394755,
-0.000654425321134147));
#91875=CARTESIAN_POINT('Ctrl Pts',(-7.17231054453004,-3.21857350729905,
-0.495960687819342));
#91876=CARTESIAN_POINT('Ctrl Pts',(-7.07590830864129,-2.8786031740959,-2.0622188852842));
#91877=CARTESIAN_POINT('Ctrl Pts',(-6.91356674160684,-0.444488776435454,
-3.77893248484412));
#91878=CARTESIAN_POINT('Ctrl Pts',(-6.71574874816972,2.92598744650415,-2.43238534371312));
#91879=CARTESIAN_POINT('Ctrl Pts',(-6.51793075473262,3.63413658105342,1.12736520596504));
#91880=CARTESIAN_POINT('Ctrl Pts',(-6.32011276129551,1.03562072148409,3.66133728555581));
#91881=CARTESIAN_POINT('Ctrl Pts',(-6.131726992809,-2.33636534844852,2.90191784046031));
#91882=CARTESIAN_POINT('Ctrl Pts',(-6.00928055546819,-3.21804476964733,
0.910705166086102));
#91883=CARTESIAN_POINT('Ctrl Pts',(-5.95277344927308,-3.22555111435178,
-0.00235478566260758));
#91884=CARTESIAN_POINT('Ctrl Pts',(-6.95622655072689,-3.22556017215824,
-0.00235126095564378));
#91885=CARTESIAN_POINT('Ctrl Pts',(-6.94681562829278,-3.22680900478704,
-0.154414820411473));
#91886=CARTESIAN_POINT('Ctrl Pts',(-6.87146537471296,-3.14810407601409,
-1.37064060382828));
#91887=CARTESIAN_POINT('Ctrl Pts',(-6.73017578998745,-1.60187655206341,
-3.45136072672716));
#91888=CARTESIAN_POINT('Ctrl Pts',(-6.53235779655034,2.02051125516165,-3.22419503472727));
#91889=CARTESIAN_POINT('Ctrl Pts',(-6.33453980311323,3.80445582041375,-0.0633661140739026));
#91890=CARTESIAN_POINT('Ctrl Pts',(-6.13672180967612,2.12676359733563,3.1551190080601));
#91891=CARTESIAN_POINT('Ctrl Pts',(-5.93890381623902,-1.48604982490852,
3.50279249639495));
#91892=CARTESIAN_POINT('Ctrl Pts',(-5.79540539658927,-3.12595508153286,
1.44301375609325));
#91893=CARTESIAN_POINT('Ctrl Pts',(-5.71784630808522,-3.22622566428263,
0.190564184027195));
#91894=CARTESIAN_POINT('Ctrl Pts',(-5.70622655072688,-3.22455715194561,
0.0026580719403353));
#91895=CARTESIAN_POINT('Origin',(-31.5777734492731,0.,0.));
#91896=CARTESIAN_POINT('',(-8.45277344927309,-3.22319594283231,0.00286971858088855));
#91897=CARTESIAN_POINT('',(-8.20622655072689,-3.21767060863508,-0.000659891891161835));
#91898=CARTESIAN_POINT('',(-31.5777734492731,-3.22275,-1.53308031181269E-14));
#91899=CARTESIAN_POINT('Ctrl Pts',(-8.45277344927309,-3.22319594283231,
0.00286971858088854));
#91900=CARTESIAN_POINT('Ctrl Pts',(-8.40127986473759,-3.21558063935123,
-0.8307531566189));
#91901=CARTESIAN_POINT('Ctrl Pts',(-8.28384694905639,-2.46091776083998,
-2.7440933325883));
#91902=CARTESIAN_POINT('Ctrl Pts',(-8.10047470222948,0.756121223608606,
-3.72909931385589));
#91903=CARTESIAN_POINT('Ctrl Pts',(-7.90265670879237,3.53860570694324,-1.39863170569708));
#91904=CARTESIAN_POINT('Ctrl Pts',(-7.70483871535527,3.10134779529267,2.20443708234665));
#91905=CARTESIAN_POINT('Ctrl Pts',(-7.50702072191815,-0.15779585471615,
3.80171033426082));
#91906=CARTESIAN_POINT('Ctrl Pts',(-7.3396656332241,-2.79358212650196,2.22656213163102));
#91907=CARTESIAN_POINT('Ctrl Pts',(-7.23824987567574,-3.21661492500036,
0.576168314220868));
#91908=CARTESIAN_POINT('Ctrl Pts',(-7.20277344927309,-3.21766867394755,
-0.000654425321134147));
#91909=CARTESIAN_POINT('Ctrl Pts',(-8.20622655072689,-3.21767060863508,
-0.000659891891162043));
#91910=CARTESIAN_POINT('Ctrl Pts',(-8.17578494850033,-3.21858239645565,
-0.495618948061391));
#91911=CARTESIAN_POINT('Ctrl Pts',(-8.07940401512807,-2.87894598482745,
-2.06151932593722));
#91912=CARTESIAN_POINT('Ctrl Pts',(-7.91708375061009,-0.445702651221169,
-3.77878929033658));
#91913=CARTESIAN_POINT('Ctrl Pts',(-7.71926575717298,2.92520576373441,-2.43332500786197));
#91914=CARTESIAN_POINT('Ctrl Pts',(-7.52144776373588,3.63449833574001,1.12619767428708));
#91915=CARTESIAN_POINT('Ctrl Pts',(-7.32362977029877,1.03679675659798,3.66100421190307));
#91916=CARTESIAN_POINT('Ctrl Pts',(-7.13522269929578,-2.33581422869672,
2.90258229478908));
#91917=CARTESIAN_POINT('Ctrl Pts',(-7.01275495943848,-3.21805883296996,
0.911046028124277));
#91918=CARTESIAN_POINT('Ctrl Pts',(-6.95622655072689,-3.22556017215824,
-0.00235126095564378));
#91919=CARTESIAN_POINT('Origin',(-31.5777734492731,0.,0.));
#91920=CARTESIAN_POINT('',(-9.70277344927309,-3.22667916477104,-0.00179405147487009));
#91921=CARTESIAN_POINT('',(-9.45622655072689,-3.2231853869298,0.00287052290945347));
#91922=CARTESIAN_POINT('',(-31.5777734492731,-3.22275,-1.53308031181269E-14));
#91923=CARTESIAN_POINT('Ctrl Pts',(-9.70277344927309,-3.22667916477104,
-0.00179405147487066));
#91924=CARTESIAN_POINT('Ctrl Pts',(-9.69618851609084,-3.22739165962895,
-0.10809806421905));
#91925=CARTESIAN_POINT('Ctrl Pts',(-9.62366425176289,-3.17451256225385,
-1.27817778786519));
#91926=CARTESIAN_POINT('Ctrl Pts',(-9.48520065628923,-1.74745727030714,
-3.37998433218895));
#91927=CARTESIAN_POINT('Ctrl Pts',(-9.28738266285213,1.88131977313113,-3.30734590096318));
#91928=CARTESIAN_POINT('Ctrl Pts',(-9.08956466941502,3.79830252985678,-0.225386088913072));
#91929=CARTESIAN_POINT('Ctrl Pts',(-8.8917466759779,2.25924731649643,3.06165030013156));
#91930=CARTESIAN_POINT('Ctrl Pts',(-8.69392868254081,-1.33547472388757,
3.56292130971895));
#91931=CARTESIAN_POINT('Ctrl Pts',(-8.54760427363919,-3.09563628545797,
1.53572413753069));
#91932=CARTESIAN_POINT('Ctrl Pts',(-8.46721919588329,-3.22533230108819,
0.236730012678338));
#91933=CARTESIAN_POINT('Ctrl Pts',(-8.45277344927309,-3.22319594283231,
0.00286971858088854));
#91934=CARTESIAN_POINT('Ctrl Pts',(-9.45622655072689,-3.2231853869298,0.00287052290945312));
#91935=CARTESIAN_POINT('Ctrl Pts',(-9.40475426870788,-3.21557354337093,
-0.830414323179482));
#91936=CARTESIAN_POINT('Ctrl Pts',(-9.28734265554316,-2.46142530178796,
-2.74341705299499));
#91937=CARTESIAN_POINT('Ctrl Pts',(-9.10399171123273,0.754923226864277,
-3.72934180192827));
#91938=CARTESIAN_POINT('Ctrl Pts',(-8.90617371779564,3.53815603498388,-1.3997682758857));
#91939=CARTESIAN_POINT('Ctrl Pts',(-8.70835572435851,3.10205560019449,2.20344058403463));
#91940=CARTESIAN_POINT('Ctrl Pts',(-8.51053773092143,-0.156574597645193,
3.80176061180093));
#91941=CARTESIAN_POINT('Ctrl Pts',(-8.34316133971087,-2.79320214739646,
2.22725889318856));
#91942=CARTESIAN_POINT('Ctrl Pts',(-8.24172427964603,-3.21660737954993,
0.576508230576168));
#91943=CARTESIAN_POINT('Ctrl Pts',(-8.20622655072689,-3.21767060863508,
-0.000659891891162043));
#91944=CARTESIAN_POINT('Origin',(-31.5777734492731,0.,0.));
#91945=CARTESIAN_POINT('',(-10.9527734492731,-3.2181054871608,-0.00135616439500266));
#91946=CARTESIAN_POINT('',(-10.7062265507269,-3.22668646461764,-0.00178921965619527));
#91947=CARTESIAN_POINT('',(-31.5777734492731,-3.22275,-1.53308031181269E-14));
#91948=CARTESIAN_POINT('Ctrl Pts',(-10.9527734492731,-3.2181054871608,-0.00135616439500295));
#91949=CARTESIAN_POINT('Ctrl Pts',(-10.9251578362984,-3.21981873729031,
-0.450214994152712));
#91950=CARTESIAN_POINT('Ctrl Pts',(-10.831602892178,-2.92310678984398,-1.96867411684349));
#91951=CARTESIAN_POINT('Ctrl Pts',(-10.6721086169119,-0.606282086762444,
-3.75637099188338));
#91952=CARTESIAN_POINT('Ctrl Pts',(-10.4742906234748,2.81888564080964,-2.55573565562428));
#91953=CARTESIAN_POINT('Ctrl Pts',(-10.2764726300377,3.67917715554996,0.970338320108655));
#91954=CARTESIAN_POINT('Ctrl Pts',(-10.0786546366006,1.19182170212393,3.61351103882891));
#91955=CARTESIAN_POINT('Ctrl Pts',(-9.88742157634569,-2.2610636442974,2.99024725147983));
#91956=CARTESIAN_POINT('Ctrl Pts',(-9.76212784723654,-3.22025697305356,
0.956394969264087));
#91957=CARTESIAN_POINT('Ctrl Pts',(-9.70277344927309,-3.22667916477104,
-0.00179405147487066));
#91958=CARTESIAN_POINT('Ctrl Pts',(-10.7062265507269,-3.22668646461764,
-0.00178921965619555));
#91959=CARTESIAN_POINT('Ctrl Pts',(-10.6996629200611,-3.22739513133839,
-0.10774868125948));
#91960=CARTESIAN_POINT('Ctrl Pts',(-10.6271599582497,-3.1747033654712,-1.27748131867));
#91961=CARTESIAN_POINT('Ctrl Pts',(-10.4887176652925,-1.74854284806569,
-3.37942262266014));
#91962=CARTESIAN_POINT('Ctrl Pts',(-10.2908996718554,1.88025713615946,-3.30794988716429));
#91963=CARTESIAN_POINT('Ctrl Pts',(-10.0930816784183,3.79822971656082,-0.226606209763087));
#91964=CARTESIAN_POINT('Ctrl Pts',(-9.89526368498117,2.26023057897525,3.06092422054745));
#91965=CARTESIAN_POINT('Ctrl Pts',(-9.69744569154406,-1.33433004645538,
3.56334992404553));
#91966=CARTESIAN_POINT('Ctrl Pts',(-9.55109998012597,-3.09539896911836,
1.53642335041516));
#91967=CARTESIAN_POINT('Ctrl Pts',(-9.47069359985358,-3.22532480858339,
0.237077601593841));
#91968=CARTESIAN_POINT('Ctrl Pts',(-9.45622655072689,-3.2231853869298,0.00287052290945312));
#91969=CARTESIAN_POINT('Origin',(-31.5777734492731,0.,0.));
#91970=CARTESIAN_POINT('',(-12.2027734492731,-3.22182548726639,0.00287273816568898));
#91971=CARTESIAN_POINT('',(-11.9562265507269,-3.21810971317159,-0.00136113665029886));
#91972=CARTESIAN_POINT('',(-31.5777734492731,-3.22275,-1.53308031181269E-14));
#91973=CARTESIAN_POINT('Ctrl Pts',(-12.2027734492731,-3.22182548726639,
0.00287273816568887));
#91974=CARTESIAN_POINT('Ctrl Pts',(-12.1541271565059,-3.21489726619265,
-0.78551235421924));
#91975=CARTESIAN_POINT('Ctrl Pts',(-12.0395415325931,-2.52718466035753,
-2.65335903695121));
#91976=CARTESIAN_POINT('Ctrl Pts',(-11.8590165775345,0.595360400383641,
-3.75811747967609));
#91977=CARTESIAN_POINT('Ctrl Pts',(-11.6611985840974,3.47531106646949,-1.54923012773011));
#91978=CARTESIAN_POINT('Ctrl Pts',(-11.4633805906603,3.19311050600954,2.06928642140315));
#91979=CARTESIAN_POINT('Ctrl Pts',(-11.2655625972232,0.00553022271176743,
3.80497968641473));
#91980=CARTESIAN_POINT('Ctrl Pts',(-11.0953602167608,-2.74138972731681,
2.31956968971646));
#91981=CARTESIAN_POINT('Ctrl Pts',(-10.9910971674441,-3.21572791490918,
0.621550135239206));
#91982=CARTESIAN_POINT('Ctrl Pts',(-10.9527734492731,-3.2181054871608,-0.00135616439500295));
#91983=CARTESIAN_POINT('Ctrl Pts',(-11.9562265507269,-3.21810971317159,
-0.00136113665029847));
#91984=CARTESIAN_POINT('Ctrl Pts',(-11.9286322402687,-3.2198280570441,-0.449872156052723));
#91985=CARTESIAN_POINT('Ctrl Pts',(-11.8350985986648,-2.92342951382292,
-1.96797377055099));
#91986=CARTESIAN_POINT('Ctrl Pts',(-11.6756256259151,-0.607488696492234,
-3.75617582624975));
#91987=CARTESIAN_POINT('Ctrl Pts',(-11.477807632478,2.81806434528784,-2.55664090162977));
#91988=CARTESIAN_POINT('Ctrl Pts',(-11.2799896390409,3.67948846292253,0.969156336866661));
#91989=CARTESIAN_POINT('Ctrl Pts',(-11.0821716456038,1.1929823568862,3.61312779323221));
#91990=CARTESIAN_POINT('Ctrl Pts',(-10.8909172828325,-2.26048748756761,
2.99090395355496));
#91991=CARTESIAN_POINT('Ctrl Pts',(-10.7656022512068,-3.22027574696849,
0.956737787048822));
#91992=CARTESIAN_POINT('Ctrl Pts',(-10.7062265507269,-3.22668646461764,
-0.00178921965619555));
#91993=CARTESIAN_POINT('Origin',(-31.5777734492731,0.,0.));
#91994=CARTESIAN_POINT('',(-13.4527734492731,-3.22751445325846,-0.00107914716668534));
#91995=CARTESIAN_POINT('',(-13.2062265507269,-3.22181528236761,0.00287197708553733));
#91996=CARTESIAN_POINT('',(-31.5777734492731,-3.22275,-1.53308031181269E-14));
#91997=CARTESIAN_POINT('Ctrl Pts',(-13.4527734492731,-3.22751445325846,
-0.0010791471666857));
#91998=CARTESIAN_POINT('Ctrl Pts',(-13.4490358078592,-3.22777825363035,
-0.061376493187223));
#91999=CARTESIAN_POINT('Ctrl Pts',(-13.3793588352996,-3.19898704244113,
-1.18518051592563));
#92000=CARTESIAN_POINT('Ctrl Pts',(-13.2437425315943,-1.8909257110314,-3.30186325470216));
#92001=CARTESIAN_POINT('Ctrl Pts',(-13.0459245381572,1.7376248539901,-3.38504961029937));
#92002=CARTESIAN_POINT('Ctrl Pts',(-12.8481065447201,3.78512772048049,-0.388212747140301));
#92003=CARTESIAN_POINT('Ctrl Pts',(-12.6502885512829,2.38858024585731,2.96185506169566));
#92004=CARTESIAN_POINT('Ctrl Pts',(-12.4524705578458,-1.18131281127045,
3.61696019321754));
#92005=CARTESIAN_POINT('Ctrl Pts',(-12.3032988571759,-3.06277764869808,
1.62924239957152));
#92006=CARTESIAN_POINT('Ctrl Pts',(-12.2200664876516,-3.22428836750058,
0.283131990909709));
#92007=CARTESIAN_POINT('Ctrl Pts',(-12.2027734492731,-3.22182548726639,
0.00287273816568887));
#92008=CARTESIAN_POINT('Ctrl Pts',(-13.2062265507269,-3.22181528236761,
0.00287197708553705));
#92009=CARTESIAN_POINT('Ctrl Pts',(-13.1576015604762,-3.21489372565932,
-0.785174075009538));
#92010=CARTESIAN_POINT('Ctrl Pts',(-13.0430372390799,-2.52766830833463,
-2.65267741427113));
#92011=CARTESIAN_POINT('Ctrl Pts',(-12.8625335865378,0.594153099425664,
-3.75830832270474));
#92012=CARTESIAN_POINT('Ctrl Pts',(-12.6647155931007,3.47481302398082,-1.55034634918851));
#92013=CARTESIAN_POINT('Ctrl Pts',(-12.4668975996636,3.19377488593328,2.0682604603992));
#92014=CARTESIAN_POINT('Ctrl Pts',(-12.2690796062265,0.00675251231494511,
3.80497749765308));
#92015=CARTESIAN_POINT('Ctrl Pts',(-12.0988559232476,-2.74098816878215,
2.32026426362444));
#92016=CARTESIAN_POINT('Ctrl Pts',(-11.9945715714144,-3.21572190458911,
0.621889237501745));
#92017=CARTESIAN_POINT('Ctrl Pts',(-11.9562265507269,-3.21810971317159,
-0.00136113665029847));
#92018=CARTESIAN_POINT('Origin',(-31.5777734492731,0.,0.));
#92019=CARTESIAN_POINT('',(-14.7027734492731,-3.21883508950441,-0.00196949714717019));
#92020=CARTESIAN_POINT('',(-14.4562265507269,-3.2275191157403,-0.00107334156349448));
#92021=CARTESIAN_POINT('',(-31.5777734492731,-3.22275,-1.53308031181269E-14));
#92022=CARTESIAN_POINT('Ctrl Pts',(-14.7027734492731,-3.21883508950441,
-0.00196949714717044));
#92023=CARTESIAN_POINT('Ctrl Pts',(-14.6780051280667,-3.22109751442067,
-0.404320281781302));
#92024=CARTESIAN_POINT('Ctrl Pts',(-14.5872974757147,-2.96496213196803,
-1.87505121301113));
#92025=CARTESIAN_POINT('Ctrl Pts',(-14.4306504922169,-0.766957879978414,
-3.7268856445739));
#92026=CARTESIAN_POINT('Ctrl Pts',(-14.2328324987798,2.70658798155444,-2.6743751598265));
#92027=CARTESIAN_POINT('Ctrl Pts',(-14.0350145053427,3.71743616166189,0.811522877903334));
#92028=CARTESIAN_POINT('Ctrl Pts',(-13.8371965119056,1.34582588168488,3.55902426144851));
#92029=CARTESIAN_POINT('Ctrl Pts',(-13.6431161598824,-2.18239091772659,
3.07747832470855));
#92030=CARTESIAN_POINT('Ctrl Pts',(-13.5149751390049,-3.2231242972573,1.00238704808438));
#92031=CARTESIAN_POINT('Ctrl Pts',(-13.4527734492731,-3.22751445325846,
-0.0010791471666857));
#92032=CARTESIAN_POINT('Ctrl Pts',(-14.4562265507269,-3.2275191157403,-0.00107334156349525));
#92033=CARTESIAN_POINT('Ctrl Pts',(-14.4525102118295,-3.22778017593927,
-0.0610267823477145));
#92034=CARTESIAN_POINT('Ctrl Pts',(-14.3828545417863,-3.19916205398302,
-1.18448531601658));
#92035=CARTESIAN_POINT('Ctrl Pts',(-14.2472595405976,-1.89198617807126,
-3.3012554666454));
#92036=CARTESIAN_POINT('Ctrl Pts',(-14.0494415471604,1.73653727148651,-3.38560742833646));
#92037=CARTESIAN_POINT('Ctrl Pts',(-13.8516235537233,3.78500260309515,-0.389428618146851));
#92038=CARTESIAN_POINT('Ctrl Pts',(-13.6538055602862,2.38953143666386,2.96108744674385));
#92039=CARTESIAN_POINT('Ctrl Pts',(-13.4559875668491,-1.18015079139549,
3.61733927958623));
#92040=CARTESIAN_POINT('Ctrl Pts',(-13.3067945636627,-3.06252272261062,
1.62994232206525));
#92041=CARTESIAN_POINT('Ctrl Pts',(-13.2235408916219,-3.22427990378457,
0.283478675752636));
#92042=CARTESIAN_POINT('Ctrl Pts',(-13.2062265507269,-3.22181528236761,
0.00287197708553705));
#92043=CARTESIAN_POINT('Origin',(-31.5777734492731,0.,0.));
#92044=CARTESIAN_POINT('',(-15.9527734492731,-3.22054328874694,0.00267261023343764));
#92045=CARTESIAN_POINT('',(-15.7062265507269,-3.21884138421527,-0.0019736436849066));
#92046=CARTESIAN_POINT('',(-31.5777734492731,-3.22275,-1.53308031181269E-14));
#92047=CARTESIAN_POINT('Ctrl Pts',(-15.9527734492731,-3.22054328874694,
0.00267261023343748));
#92048=CARTESIAN_POINT('Ctrl Pts',(-15.9069744482743,-3.21466005692855,
-0.740318326976134));
#92049=CARTESIAN_POINT('Ctrl Pts',(-15.7952361161298,-2.59028920630862,
-2.56196187539477));
#92050=CARTESIAN_POINT('Ctrl Pts',(-15.6175584528396,0.433502191222674,
-3.78020857197022));
#92051=CARTESIAN_POINT('Ctrl Pts',(-15.4197404594025,3.40561062963269,-1.69697296287383));
#92052=CARTESIAN_POINT('Ctrl Pts',(-15.2219224659654,3.27898758080047,1.93032159039582));
#92053=CARTESIAN_POINT('Ctrl Pts',(-15.0241044725282,0.168846106669414,
3.80123558723405));
#92054=CARTESIAN_POINT('Ctrl Pts',(-14.8510548002975,-2.68627752097958,
2.41224661168182));
#92055=CARTESIAN_POINT('Ctrl Pts',(-14.7439444592124,-3.21507438574341,
0.666835950556258));
#92056=CARTESIAN_POINT('Ctrl Pts',(-14.7027734492731,-3.21883508950441,
-0.00196949714717044));
#92057=CARTESIAN_POINT('Ctrl Pts',(-15.7062265507269,-3.21884138421527,
-0.00197364368490657));
#92058=CARTESIAN_POINT('Ctrl Pts',(-15.681479532037,-3.22110690703042,-0.403976324022853));
#92059=CARTESIAN_POINT('Ctrl Pts',(-15.5907931822014,-2.96526531461261,
-1.87435049020682));
#92060=CARTESIAN_POINT('Ctrl Pts',(-15.4341675012202,-0.768155000592636,
-3.72663886754987));
#92061=CARTESIAN_POINT('Ctrl Pts',(-15.236349507783,2.70572858711511,-2.67524431911123));
#92062=CARTESIAN_POINT('Ctrl Pts',(-15.038531514346,3.71769644791273,0.81032862176155));
#92063=CARTESIAN_POINT('Ctrl Pts',(-14.8407135209088,1.34696901673613,3.5585915503218));
#92064=CARTESIAN_POINT('Ctrl Pts',(-14.6466118663692,-2.18178936818306,
3.07812631949869));
#92065=CARTESIAN_POINT('Ctrl Pts',(-14.5184495429752,-3.22314816164128,
1.00273244260953));
#92066=CARTESIAN_POINT('Ctrl Pts',(-14.4562265507269,-3.2275191157403,-0.00107334156349525));
#92067=CARTESIAN_POINT('Origin',(-31.5777734492731,0.,0.));
#92068=CARTESIAN_POINT('',(-17.2027734492731,-3.22793661423918,-0.000264189382539215));
#92069=CARTESIAN_POINT('',(-16.9562265507269,-3.22053404262666,0.00267039071692468));
#92070=CARTESIAN_POINT('',(-31.5777734492731,-3.22275,-1.53308031181269E-14));
#92071=CARTESIAN_POINT('Ctrl Pts',(-17.2027734492731,-3.22793661423918,
-0.00026418938253939));
#92072=CARTESIAN_POINT('Ctrl Pts',(-17.2018830996275,-3.22795359918395,
-0.0146226889311297));
#92073=CARTESIAN_POINT('Ctrl Pts',(-17.1350534188363,-3.22138006304283,
-1.09235627156946));
#92074=CARTESIAN_POINT('Ctrl Pts',(-17.0022844068993,-2.03090874143955,
-3.21765608499983));
#92075=CARTESIAN_POINT('Ctrl Pts',(-16.8044664134622,1.59072709321647,-3.45651389586373));
#92076=CARTESIAN_POINT('Ctrl Pts',(-16.6066484200251,3.7649760515017,-0.55032384012566));
#92077=CARTESIAN_POINT('Ctrl Pts',(-16.408830426588,2.51351047331346,2.85660044422309));
#92078=CARTESIAN_POINT('Ctrl Pts',(-16.2110124331509,-1.02497346786645,
3.66433218848425));
#92079=CARTESIAN_POINT('Ctrl Pts',(-16.0589934407126,-3.02753062537622,
1.72284050673799));
#92080=CARTESIAN_POINT('Ctrl Pts',(-15.97291377942,-3.22313046813009,0.329406435103203));
#92081=CARTESIAN_POINT('Ctrl Pts',(-15.9527734492731,-3.22054328874694,
0.00267261023343748));
#92082=CARTESIAN_POINT('Ctrl Pts',(-16.9562265507269,-3.22053404262666,
0.00267039071692496));
#92083=CARTESIAN_POINT('Ctrl Pts',(-16.9104488522446,-3.21465963284635,
-0.739980205315209));
#92084=CARTESIAN_POINT('Ctrl Pts',(-16.7987318226165,-2.5907494278201,-2.5612756850456));
#92085=CARTESIAN_POINT('Ctrl Pts',(-16.6210754618428,0.432287811384032,
-3.7803474181876));
#92086=CARTESIAN_POINT('Ctrl Pts',(-16.4232574684057,3.40506513462136,-1.69806677814945));
#92087=CARTESIAN_POINT('Ctrl Pts',(-16.2254394749686,3.27960731114141,1.92926805778166));
#92088=CARTESIAN_POINT('Ctrl Pts',(-16.0276214815315,0.170067175844205,
3.80118093620512));
#92089=CARTESIAN_POINT('Ctrl Pts',(-15.8545505067843,-2.68585385572339,
2.41293840251175));
#92090=CARTESIAN_POINT('Ctrl Pts',(-15.7474188631827,-3.21507033911092,
0.667174435285191));
#92091=CARTESIAN_POINT('Ctrl Pts',(-15.7062265507269,-3.21884138421527,
-0.00197364368490657));
#92092=CARTESIAN_POINT('Origin',(-31.5777734492731,0.,0.));
#92093=CARTESIAN_POINT('',(-18.4527734492731,-3.21982010873651,-0.00245263893930523));
#92094=CARTESIAN_POINT('',(-18.2062265507269,-3.22793772000202,-0.000257889290232183));
#92095=CARTESIAN_POINT('',(-31.5777734492731,-3.22275,-1.53308031181269E-14));
#92096=CARTESIAN_POINT('Ctrl Pts',(-18.4527734492731,-3.21982010873651,
-0.00245263893930543));
#92097=CARTESIAN_POINT('Ctrl Pts',(-18.4308524198351,-3.22236380461367,
-0.35827632108061));
#92098=CARTESIAN_POINT('Ctrl Pts',(-18.3429920592514,-3.00424192805471,
-1.78140187471239));
#92099=CARTESIAN_POINT('Ctrl Pts',(-18.189192367522,-0.926219993698007,
-3.69053079118249));
#92100=CARTESIAN_POINT('Ctrl Pts',(-17.9913743740849,2.5893014591106,-2.78808517646783));
#92101=CARTESIAN_POINT('Ctrl Pts',(-17.7935563806477,3.74884307925887,0.651211612676593));
#92102=CARTESIAN_POINT('Ctrl Pts',(-17.5957383872107,1.49734939509152,3.49797738506285));
#92103=CARTESIAN_POINT('Ctrl Pts',(-17.3988107434191,-2.10030201134441,
3.1634803998261));
#92104=CARTESIAN_POINT('Ctrl Pts',(-17.2678224307732,-3.22669569348036,
1.04876837458784));
#92105=CARTESIAN_POINT('Ctrl Pts',(-17.2027734492731,-3.22793661423918,
-0.00026418938253939));
#92106=CARTESIAN_POINT('Ctrl Pts',(-18.2062265507269,-3.22793772000202,
-0.000257889290232734));
#92107=CARTESIAN_POINT('Ctrl Pts',(-18.2053575035978,-3.22795391650523,
-0.0142728313140034));
#92108=CARTESIAN_POINT('Ctrl Pts',(-18.138549125323,-3.22153971724754,-1.09166239659244));
#92109=CARTESIAN_POINT('Ctrl Pts',(-18.0058014159026,-2.03194214307649,
-3.21700333870802));
#92110=CARTESIAN_POINT('Ctrl Pts',(-17.8079834224654,1.5896165698452,-3.45702451755008));
#92111=CARTESIAN_POINT('Ctrl Pts',(-17.6101654290284,3.76479886064709,-0.551533220159296));
#92112=CARTESIAN_POINT('Ctrl Pts',(-17.4123474355912,2.51442783918464,2.85579270879419));
#92113=CARTESIAN_POINT('Ctrl Pts',(-17.2145294421542,-1.0237962474182,3.66466104815183));
#92114=CARTESIAN_POINT('Ctrl Pts',(-17.0624891471994,-3.02725756873777,
1.72354089465449));
#92115=CARTESIAN_POINT('Ctrl Pts',(-16.9763881833903,-3.22312127824644,
0.329752114150966));
#92116=CARTESIAN_POINT('Ctrl Pts',(-16.9562265507269,-3.22053404262666,
0.00267039071692496));
#92117=CARTESIAN_POINT('Origin',(-31.5777734492731,0.,0.));
#92118=CARTESIAN_POINT('',(-19.7027734492731,-3.21942420511343,0.00228930942898773));
#92119=CARTESIAN_POINT('',(-19.4562265507269,-3.21982813535995,-0.0024556690389646));
#92120=CARTESIAN_POINT('',(-31.5777734492731,-3.22275,-1.53308031181269E-14));
#92121=CARTESIAN_POINT('Ctrl Pts',(-19.7027734492731,-3.21942420511343,
0.00228930942898737));
#92122=CARTESIAN_POINT('Ctrl Pts',(-19.6598217400426,-3.21481005975396,
-0.695121887590858));
#92123=CARTESIAN_POINT('Ctrl Pts',(-19.5509306996665,-2.6502951772353,-2.47000221202959));
#92124=CARTESIAN_POINT('Ctrl Pts',(-19.3761003281446,0.270844937974172,
-3.7953318717822));
#92125=CARTESIAN_POINT('Ctrl Pts',(-19.1782823347075,3.32963287034385,-1.84158788715549));
#92126=CARTESIAN_POINT('Ctrl Pts',(-18.9804643412704,3.35882072849595,1.78779873341992));
#92127=CARTESIAN_POINT('Ctrl Pts',(-18.7826463478333,0.331850768478793,
3.79048493795346));
#92128=CARTESIAN_POINT('Ctrl Pts',(-18.6067493838342,-2.62817580074329,
2.50451000044191));
#92129=CARTESIAN_POINT('Ctrl Pts',(-18.4967917509808,-3.21471226592786,
0.71205551130674));
#92130=CARTESIAN_POINT('Ctrl Pts',(-18.4527734492731,-3.21982010873651,
-0.00245263893930543));
#92131=CARTESIAN_POINT('Ctrl Pts',(-19.4562265507269,-3.21982813535995,
-0.00245566903896481));
#92132=CARTESIAN_POINT('Ctrl Pts',(-19.4343268238054,-3.22237293973325,
-0.357931261263622));
#92133=CARTESIAN_POINT('Ctrl Pts',(-19.3464877657381,-3.00452611195908,
-1.78070113839176));
#92134=CARTESIAN_POINT('Ctrl Pts',(-19.1927093765252,-0.927405418628458,
-3.69023285763479));
#92135=CARTESIAN_POINT('Ctrl Pts',(-18.9948913830881,2.58840554981504,-2.78891664697164));
#92136=CARTESIAN_POINT('Ctrl Pts',(-18.797073389651,3.74905186462063,0.650007284923323));
#92137=CARTESIAN_POINT('Ctrl Pts',(-18.5992553962139,1.49847290337135,3.4974960059921));
#92138=CARTESIAN_POINT('Ctrl Pts',(-18.4023064499059,-2.09967475031009,
3.16411868726491));
#92139=CARTESIAN_POINT('Ctrl Pts',(-18.2712968347435,-3.22672499973764,
1.04911702658821));
#92140=CARTESIAN_POINT('Ctrl Pts',(-18.2062265507269,-3.22793772000202,
-0.000257889290232734));
#92141=CARTESIAN_POINT('Origin',(-31.5777734492731,0.,0.));
#92142=CARTESIAN_POINT('',(-20.9527734492731,-3.22783470827694,0.000576931514566297));
#92143=CARTESIAN_POINT('',(-20.7062265507269,-3.21941642796096,0.00228582146781398));
#92144=CARTESIAN_POINT('',(-31.5777734492731,-3.22275,-1.53308031181269E-14));
#92145=CARTESIAN_POINT('Ctrl Pts',(-20.9527734492731,-3.22783470827694,
0.000576931514566295));
#92146=CARTESIAN_POINT('Ctrl Pts',(-20.8887910602502,-3.22527243766867,
-1.03134253166322));
#92147=CARTESIAN_POINT('Ctrl Pts',(-20.7588693400816,-2.1314552457683,-3.13141661665854));
#92148=CARTESIAN_POINT('Ctrl Pts',(-20.5630082887673,1.44089725711671,-3.52160703256702));
#92149=CARTESIAN_POINT('Ctrl Pts',(-20.3651902953302,3.73788466707397,-0.711420559897795));
#92150=CARTESIAN_POINT('Ctrl Pts',(-20.1673723018931,2.63380772376682,2.7460804561444));
#92151=CARTESIAN_POINT('Ctrl Pts',(-19.9695543084559,-0.866744862987072,
3.70494997805335));
#92152=CARTESIAN_POINT('Ctrl Pts',(-19.8146880242493,-2.98982485439288,
1.81648289572435));
#92153=CARTESIAN_POINT('Ctrl Pts',(-19.7257610711883,-3.22189368143663,
0.375541624733414));
#92154=CARTESIAN_POINT('Ctrl Pts',(-19.7027734492731,-3.21942420511343,
0.00228930942898737));
#92155=CARTESIAN_POINT('Ctrl Pts',(-20.7062265507269,-3.21941642796096,
0.00228582146781373));
#92156=CARTESIAN_POINT('Ctrl Pts',(-20.6632961440129,-3.21481230975648,
-0.69478358435536));
#92157=CARTESIAN_POINT('Ctrl Pts',(-20.5544264061532,-2.65073246007064,
-2.46931218000302));
#92158=CARTESIAN_POINT('Ctrl Pts',(-20.3796173371479,0.269625717635743,
-3.79541846526285));
#92159=CARTESIAN_POINT('Ctrl Pts',(-20.1817993437108,3.3290409282824,-1.84265728009565));
#92160=CARTESIAN_POINT('Ctrl Pts',(-19.9839813502737,3.35939466694879,1.78671957109805));
#92161=CARTESIAN_POINT('Ctrl Pts',(-19.7861633568365,0.333068366514352,
3.79037792539165));
#92162=CARTESIAN_POINT('Ctrl Pts',(-19.610245090321,-2.62772951399423,2.50519836286118));
#92163=CARTESIAN_POINT('Ctrl Pts',(-19.5002661549511,-3.21471062052383,
0.712393627896549));
#92164=CARTESIAN_POINT('Ctrl Pts',(-19.4562265507269,-3.21982813535995,
-0.00245566903896481));
#92165=CARTESIAN_POINT('Origin',(-31.5777734492731,0.,0.));
#92166=CARTESIAN_POINT('',(-22.2027734492731,-3.22100822472723,-0.00277034754127511));
#92167=CARTESIAN_POINT('',(-21.9562265507269,-3.22783176676599,0.000583108904914156));
#92168=CARTESIAN_POINT('',(-31.5777734492731,-3.22275,-1.53308031181269E-14));
#92169=CARTESIAN_POINT('Ctrl Pts',(-22.2027734492731,-3.22100822472723,
-0.00277034754127548));
#92170=CARTESIAN_POINT('Ctrl Pts',(-22.1836997116034,-3.22357544039283,
-0.312087844936352));
#92171=CARTESIAN_POINT('Ctrl Pts',(-22.0986866427881,-3.04101832689042,
-1.68777152984388));
#92172=CARTESIAN_POINT('Ctrl Pts',(-21.947734242827,-1.08377487127288,-3.64737344205279));
#92173=CARTESIAN_POINT('Ctrl Pts',(-21.7499162493899,2.46724225947258,-2.89665611187517));
#92174=CARTESIAN_POINT('Ctrl Pts',(-21.5520982559528,3.7733400181795,0.489700014903892));
#92175=CARTESIAN_POINT('Ctrl Pts',(-21.3542802625157,1.64611294971294,3.43048293308387));
#92176=CARTESIAN_POINT('Ctrl Pts',(-21.1564622690786,-1.97889603910867,
3.24990330068325));
#92177=CARTESIAN_POINT('Ctrl Pts',(-21.0226266646644,-3.21323182514106,
1.12710744043192));
#92178=CARTESIAN_POINT('Ctrl Pts',(-20.9547303913959,-3.22791307695557,
0.0321388455921796));
#92179=CARTESIAN_POINT('Ctrl Pts',(-20.9527734492731,-3.22783470827694,
0.000576931514566295));
#92180=CARTESIAN_POINT('Ctrl Pts',(-21.9562265507269,-3.22783176676599,
0.000583108904914152));
#92181=CARTESIAN_POINT('Ctrl Pts',(-21.8922654642205,-3.22524488400269,
-1.03099509137694));
#92182=CARTESIAN_POINT('Ctrl Pts',(-21.7623650465684,-2.13207240585389,
-3.13077414396875));
#92183=CARTESIAN_POINT('Ctrl Pts',(-21.5665252977705,1.43976583982743,-3.52206951670956));
#92184=CARTESIAN_POINT('Ctrl Pts',(-21.3687073043334,3.7376557293535,-0.712621219793359));
#92185=CARTESIAN_POINT('Ctrl Pts',(-21.1708893108963,2.63468957378667,2.74523408908033));
#92186=CARTESIAN_POINT('Ctrl Pts',(-20.9730713174592,-0.865554611853212,
3.70522800485591));
#92187=CARTESIAN_POINT('Ctrl Pts',(-20.8181837307361,-2.98953313583763,
1.81718346053193));
#92188=CARTESIAN_POINT('Ctrl Pts',(-20.7292354751586,-3.22188404511044,
0.375886225235549));
#92189=CARTESIAN_POINT('Ctrl Pts',(-20.7062265507269,-3.21941642796096,
0.00228582146781373));
#92190=CARTESIAN_POINT('Origin',(-31.5777734492731,0.,0.));
#92191=CARTESIAN_POINT('',(-23.4527734492731,-3.21852952379537,0.00175287054439046));
#92192=CARTESIAN_POINT('',(-23.2062265507269,-3.2210175372949,-0.0027720277556742));
#92193=CARTESIAN_POINT('',(-31.5777734492731,-3.22275,-1.53308031181269E-14));
#92194=CARTESIAN_POINT('Ctrl Pts',(-23.4527734492731,-3.21852952379537,
0.00175287054439036));
#92195=CARTESIAN_POINT('Ctrl Pts',(-23.412669031811,-3.21528819727374,-0.649881444060061));
#92196=CARTESIAN_POINT('Ctrl Pts',(-23.3066252832032,-2.70726897394943,
-2.37757378032704));
#92197=CARTESIAN_POINT('Ctrl Pts',(-23.1346422034496,0.107688455305257,
-3.80345950341412));
#92198=CARTESIAN_POINT('Ctrl Pts',(-22.9368242100126,3.24751783306243,-1.98280834205173));
#92199=CARTESIAN_POINT('Ctrl Pts',(-22.7390062165755,3.43246279827112,1.64198055282517));
#92200=CARTESIAN_POINT('Ctrl Pts',(-22.5411882231383,0.494243753116372,
3.77274755449071));
#92201=CARTESIAN_POINT('Ctrl Pts',(-22.3624439673709,-2.56701675396682,
2.59627028778708));
#92202=CARTESIAN_POINT('Ctrl Pts',(-22.2496390427492,-3.21470038471007,
0.7572457719529));
#92203=CARTESIAN_POINT('Ctrl Pts',(-22.2027734492731,-3.22100822472723,
-0.00277034754127548));
#92204=CARTESIAN_POINT('Ctrl Pts',(-23.2062265507269,-3.2210175372949,-0.00277202775567441));
#92205=CARTESIAN_POINT('Ctrl Pts',(-23.1871741155737,-3.22358401811418,
-0.311741735937044));
#92206=CARTESIAN_POINT('Ctrl Pts',(-23.1021823492748,-3.04128404879359,
-1.68707109660414));
#92207=CARTESIAN_POINT('Ctrl Pts',(-22.9512512518303,-1.08494641550995,
-3.6470249011433));
#92208=CARTESIAN_POINT('Ctrl Pts',(-22.7534332583931,2.46631148668775,-2.89744836100596));
#92209=CARTESIAN_POINT('Ctrl Pts',(-22.555615264956,3.77349691781262,0.488487835391227));
#92210=CARTESIAN_POINT('Ctrl Pts',(-22.357797271519,1.64721476033769,3.42995377336155));
#92211=CARTESIAN_POINT('Ctrl Pts',(-22.1599792780818,-1.97785184410161,
3.25053863795708));
#92212=CARTESIAN_POINT('Ctrl Pts',(-22.0261223711511,-3.21306598821237,
1.12780169803537));
#92213=CARTESIAN_POINT('Ctrl Pts',(-21.9582047953662,-3.2279117761473,0.0324886651761775));
#92214=CARTESIAN_POINT('Ctrl Pts',(-21.9562265507269,-3.22783176676599,
0.000583108904914152));
#92215=CARTESIAN_POINT('Origin',(-31.5777734492731,0.,0.));
#92216=CARTESIAN_POINT('',(-24.7027734492731,-3.22724337194307,0.00136199953838144));
#92217=CARTESIAN_POINT('',(-24.4562265507269,-3.21852362056934,0.00174837132580694));
#92218=CARTESIAN_POINT('',(-31.5777734492731,-3.22275,-1.53308031181269E-14));
#92219=CARTESIAN_POINT('Ctrl Pts',(-24.7027734492731,-3.22724337194307,
0.00136199953838148));
#92220=CARTESIAN_POINT('Ctrl Pts',(-24.6416383520185,-3.22197027182432,
-0.985117712154));
#92221=CARTESIAN_POINT('Ctrl Pts',(-24.5145639236183,-2.2122594842165,-3.04493847307747));
#92222=CARTESIAN_POINT('Ctrl Pts',(-24.3215501640723,1.28841151633002,-3.5802090396263));
#92223=CARTESIAN_POINT('Ctrl Pts',(-24.1237321706352,3.70390350292133,-0.871205967781821));
#92224=CARTESIAN_POINT('Ctrl Pts',(-23.925914177198,2.74925026171735,2.63049881095482));
#92225=CARTESIAN_POINT('Ctrl Pts',(-23.728096183761,-0.706918648264489,
3.73873869412743));
#92226=CARTESIAN_POINT('Ctrl Pts',(-23.570382607786,-2.94958875270477,1.91012798661397));
#92227=CARTESIAN_POINT('Ctrl Pts',(-23.4786083629567,-3.22061755788753,
0.421529975821576));
#92228=CARTESIAN_POINT('Ctrl Pts',(-23.4527734492731,-3.21852952379537,
0.00175287054439036));
#92229=CARTESIAN_POINT('Ctrl Pts',(-24.4562265507269,-3.21852362056934,
0.00174837132580694));
#92230=CARTESIAN_POINT('Ctrl Pts',(-24.4161434357813,-3.21529268052088,
-0.649542676209371));
#92231=CARTESIAN_POINT('Ctrl Pts',(-24.3101209896899,-2.70768382376327,
-2.37688058269757));
#92232=CARTESIAN_POINT('Ctrl Pts',(-24.1381592124529,0.106466641732784,
-3.80349368464174));
#92233=CARTESIAN_POINT('Ctrl Pts',(-23.9403412190158,3.2468805350555,-1.98385134146986));
#92234=CARTESIAN_POINT('Ctrl Pts',(-23.7425232255787,3.43298988692531,1.64087774991356));
#92235=CARTESIAN_POINT('Ctrl Pts',(-23.5447052321416,0.495455635705227,
3.77258837765834));
#92236=CARTESIAN_POINT('Ctrl Pts',(-23.3659396738577,-2.56654734681356,
2.59695452658232));
#92237=CARTESIAN_POINT('Ctrl Pts',(-23.2531134467194,-3.21470158249578,
0.757583824704844));
#92238=CARTESIAN_POINT('Ctrl Pts',(-23.2062265507269,-3.2210175372949,-0.00277202775567441));
#92239=CARTESIAN_POINT('Origin',(-31.5777734492731,0.,0.));
#92240=CARTESIAN_POINT('',(-25.9527734492731,-3.22233294691401,-0.00289610800939979));
#92241=CARTESIAN_POINT('',(-25.7062265507269,-3.22723723078879,0.00136747617323019));
#92242=CARTESIAN_POINT('',(-31.5777734492731,-3.22275,-1.53308031181269E-14));
#92243=CARTESIAN_POINT('Ctrl Pts',(-25.9527734492731,-3.22233294691401,
-0.00289610800939966));
#92244=CARTESIAN_POINT('Ctrl Pts',(-25.9365470033718,-3.22469450962706,
-0.265764063637563));
#92245=CARTESIAN_POINT('Ctrl Pts',(-25.8543812263248,-3.07536251639807,
-1.59419957501449));
#92246=CARTESIAN_POINT('Ctrl Pts',(-25.706276118132,-1.23933208819682,-3.59749306908928));
#92247=CARTESIAN_POINT('Ctrl Pts',(-25.508458124695,2.34063535810499,-2.99988788509652));
#92248=CARTESIAN_POINT('Ctrl Pts',(-25.3106401312578,3.79088182894556,0.327285808551454));
#92249=CARTESIAN_POINT('Ctrl Pts',(-25.1128221378208,1.79184233806401,3.35666530231748));
#92250=CARTESIAN_POINT('Ctrl Pts',(-24.9150041443836,-1.83757679742267,
3.3318482175997));
#92251=CARTESIAN_POINT('Ctrl Pts',(-24.7783212482011,-3.19006587685143,
1.21999735035492));
#92252=CARTESIAN_POINT('Ctrl Pts',(-24.7075776831642,-3.22765775267426,
0.0788834148409687));
#92253=CARTESIAN_POINT('Ctrl Pts',(-24.7027734492731,-3.22724337194307,
0.00136199953838148));
#92254=CARTESIAN_POINT('Ctrl Pts',(-25.7062265507269,-3.22723723078879,
0.00136747617323013));
#92255=CARTESIAN_POINT('Ctrl Pts',(-25.6451127559888,-3.22194803267696,
-0.98477327470211));
#92256=CARTESIAN_POINT('Ctrl Pts',(-25.5180596301051,-2.21285103742733,
-3.04428668153654));
#92257=CARTESIAN_POINT('Ctrl Pts',(-25.3250671730756,1.28726128874941,-3.58062253845296));
#92258=CARTESIAN_POINT('Ctrl Pts',(-25.1272491796384,3.70362324127845,-0.872395691996212));
#92259=CARTESIAN_POINT('Ctrl Pts',(-24.9294311862013,2.750094969933,2.62961537102403));
#92260=CARTESIAN_POINT('Ctrl Pts',(-24.7316131927642,-0.705717560089592,
3.7389653762666));
#92261=CARTESIAN_POINT('Ctrl Pts',(-24.5738783142728,-2.94927783324677,
1.91082839397675));
#92262=CARTESIAN_POINT('Ctrl Pts',(-24.482082766927,-3.22060778704532,0.421873457838835));
#92263=CARTESIAN_POINT('Ctrl Pts',(-24.4562265507269,-3.21852362056934,
0.00174837132580694));
#92264=CARTESIAN_POINT('Origin',(-31.5777734492731,0.,0.));
#92265=CARTESIAN_POINT('',(-27.2027734492731,-3.21790541760435,0.00110453296622242));
#92266=CARTESIAN_POINT('',(-26.9562265507269,-3.22234299281458,-0.0028962677614916));
#92267=CARTESIAN_POINT('',(-31.5777734492731,-3.22275,-1.53308031181269E-14));
#92268=CARTESIAN_POINT('Ctrl Pts',(-27.2027734492731,-3.21790541760435,
0.00110453296622223));
#92269=CARTESIAN_POINT('Ctrl Pts',(-27.1655163235793,-3.21603557647176,
-0.60456104426713));
#92270=CARTESIAN_POINT('Ctrl Pts',(-27.0623198667399,-2.76128025085132,
-2.28476931242144));
#92271=CARTESIAN_POINT('Ctrl Pts',(-26.8931840787547,-0.0556657981542161,
-3.80457269099369));
#92272=CARTESIAN_POINT('Ctrl Pts',(-26.6953660853176,3.15941649666726,-2.12037600768663));
#92273=CARTESIAN_POINT('Ctrl Pts',(-26.4975480918805,3.49977824828921,1.49313686004087));
#92274=CARTESIAN_POINT('Ctrl Pts',(-26.2997300984434,0.655725629921395,
3.7480555903611));
#92275=CARTESIAN_POINT('Ctrl Pts',(-26.1181385509076,-2.5027348685329,2.68743146592178));
#92276=CARTESIAN_POINT('Ctrl Pts',(-26.0024863345175,-3.21509783844571,
0.802451199222868));
#92277=CARTESIAN_POINT('Ctrl Pts',(-25.9527734492731,-3.22233294691401,
-0.00289610800939966));
#92278=CARTESIAN_POINT('Ctrl Pts',(-26.9562265507269,-3.22234299281458,
-0.00289626776149219));
#92279=CARTESIAN_POINT('Ctrl Pts',(-26.9400214073421,-3.22470229693142,
-0.265417076013672));
#92280=CARTESIAN_POINT('Ctrl Pts',(-26.8578769328116,-3.07561050857835,
-1.59350023865848));
#92281=CARTESIAN_POINT('Ctrl Pts',(-26.7097931271353,-1.24048741938786,
-3.59709412115127));
#92282=CARTESIAN_POINT('Ctrl Pts',(-26.5119751336982,2.33967134712765,-3.0006396835025));
#92283=CARTESIAN_POINT('Ctrl Pts',(-26.3141571402611,3.79098660083381,0.326068132244285));
#92284=CARTESIAN_POINT('Ctrl Pts',(-26.116339146824,1.79292039549545,3.35608927428751));
#92285=CARTESIAN_POINT('Ctrl Pts',(-25.9185211533869,-1.83650628133122,
3.33243818231883));
#92286=CARTESIAN_POINT('Ctrl Pts',(-25.7818169546879,-3.18988452276931,
1.22069290348142));
#92287=CARTESIAN_POINT('Ctrl Pts',(-25.7110520871345,-3.22765486510794,
0.0792330074626153));
#92288=CARTESIAN_POINT('Ctrl Pts',(-25.7062265507269,-3.22723723078879,
0.00136747617323013));
#92289=CARTESIAN_POINT('Origin',(-31.5777734492731,0.,0.));
#92290=CARTESIAN_POINT('',(-28.4527734492731,-3.22624365146105,0.00223892240347571));
#92291=CARTESIAN_POINT('',(-28.2062265507269,-3.21789432005771,0.00111814815214523));
#92292=CARTESIAN_POINT('',(-31.5777734492731,-3.22275,-1.53308031181269E-14));
#92293=CARTESIAN_POINT('Ctrl Pts',(-28.4527734492731,-3.22624365146105,
0.0022389224034757));
#92294=CARTESIAN_POINT('Ctrl Pts',(-28.3944856437869,-3.21930460272821,
-0.938987714550561));
#92295=CARTESIAN_POINT('Ctrl Pts',(-28.270258507155,-2.28972814938004,-2.95761805447462));
#92296=CARTESIAN_POINT('Ctrl Pts',(-28.0800920393773,1.13358660582709,-3.63202487607056));
#92297=CARTESIAN_POINT('Ctrl Pts',(-27.8822740459403,3.66307656578549,-1.02948321404113));
#92298=CARTESIAN_POINT('Ctrl Pts',(-27.6844560525031,2.85963502885877,2.51011956145336));
#92299=CARTESIAN_POINT('Ctrl Pts',(-27.4866380590661,-0.545794501053909,
3.76560941640859));
#92300=CARTESIAN_POINT('Ctrl Pts',(-27.3260771913227,-2.90674871047044,
2.00373429321426));
#92301=CARTESIAN_POINT('Ctrl Pts',(-27.231455654725,-3.21934490512597,0.467373043966351));
#92302=CARTESIAN_POINT('Ctrl Pts',(-27.2027734492731,-3.21790541760435,
0.00110453296622223));
#92303=CARTESIAN_POINT('Ctrl Pts',(-28.2062265507269,-3.21789432005771,
0.00111814815214498));
#92304=CARTESIAN_POINT('Ctrl Pts',(-28.1689907275496,-3.21603799243794,
-0.604211702459132));
#92305=CARTESIAN_POINT('Ctrl Pts',(-28.0658155732266,-2.76168588303602,
-2.28410602743074));
#92306=CARTESIAN_POINT('Ctrl Pts',(-27.896701087758,-0.056879441065127,
-3.80453263781198));
#92307=CARTESIAN_POINT('Ctrl Pts',(-27.6988830943209,3.15873057113267,-2.12140205749341));
#92308=CARTESIAN_POINT('Ctrl Pts',(-27.5010651008837,3.50025983817255,1.49201838676206));
#92309=CARTESIAN_POINT('Ctrl Pts',(-27.3032471074467,0.656928350055686,
3.74784144106381));
#92310=CARTESIAN_POINT('Ctrl Pts',(-27.1216342573943,-2.50224137881404,
2.6881120697053));
#92311=CARTESIAN_POINT('Ctrl Pts',(-27.0059607384878,-3.21510220073116,
0.802789856618959));
#92312=CARTESIAN_POINT('Ctrl Pts',(-26.9562265507269,-3.22234299281458,
-0.00289626776149219));
#92313=CARTESIAN_POINT('Origin',(-0.4,5.160062080289E-16,2.1385152528819E-16));
#92314=CARTESIAN_POINT('',(-0.4,-0.4995344189117,3.90114782651498));
#92315=CARTESIAN_POINT('Ctrl Pts',(-0.399999999999999,3.01796675574746,
-1.14524144678479));
#92316=CARTESIAN_POINT('Ctrl Pts',(-0.4,3.05385943172044,-1.07546057251878));
#92317=CARTESIAN_POINT('Ctrl Pts',(-0.399999999999999,3.08696973524706,
-1.00441532534134));
#92318=CARTESIAN_POINT('Ctrl Pts',(-0.399999999999999,3.11717685628419,
-0.932224456809624));
#92319=CARTESIAN_POINT('Ctrl Pts',(-0.399999999999998,3.15685849482143,
-0.837390793341891));
#92320=CARTESIAN_POINT('Ctrl Pts',(-0.4,3.1915324278058,-0.740581154760933));
#92321=CARTESIAN_POINT('Ctrl Pts',(-0.4,3.2213387732556,-0.642171654880859));
#92322=CARTESIAN_POINT('Ctrl Pts',(-0.4,3.24002793996668,-0.580466956721544));
#92323=CARTESIAN_POINT('Ctrl Pts',(-0.399999999999998,3.25680254187822,
-0.518132581512819));
#92324=CARTESIAN_POINT('Ctrl Pts',(-0.399999999999998,3.27168843256541,
-0.455255819308803));
#92325=CARTESIAN_POINT('Ctrl Pts',(-0.399999999999998,3.27945954784241,
-0.422431275746028));
#92326=CARTESIAN_POINT('Ctrl Pts',(-0.399999999999996,3.28671581835832,
-0.389458854605961));
#92327=CARTESIAN_POINT('Ctrl Pts',(-0.399999999999996,3.29346019208002,
-0.356350636477125));
#92328=CARTESIAN_POINT('Ctrl Pts',(-0.399999999999996,3.29755533371787,
-0.336247533029876));
#92329=CARTESIAN_POINT('Ctrl Pts',(-0.399999999999985,3.30146027548614,
-0.316101286577043));
#92330=CARTESIAN_POINT('Ctrl Pts',(-0.399999999999986,3.30517468015687,
-0.295922536912268));
#92331=CARTESIAN_POINT('Ctrl Pts',(-0.399999999999987,3.32438655606123,
-0.191552747180045));
#92332=CARTESIAN_POINT('Ctrl Pts',(-0.399999999999996,3.33851780246706,
-0.0862519001458806));
#92333=CARTESIAN_POINT('Ctrl Pts',(-0.399999999999995,3.34771253438542,
0.0195864485897636));
#92334=CARTESIAN_POINT('Ctrl Pts',(-0.399999999999995,3.3564903695163,0.120625998624962));
#92335=CARTESIAN_POINT('Ctrl Pts',(-0.399999999999991,3.36076889984354,
0.222156205388883));
#92336=CARTESIAN_POINT('Ctrl Pts',(-0.399999999999991,3.36063532362138,
0.323852939879256));
#92337=CARTESIAN_POINT('Ctrl Pts',(-0.39999999999999,3.36057596369294,0.36904594491764));
#92338=CARTESIAN_POINT('Ctrl Pts',(-0.399999999999997,3.35964479686966,
0.414272015762765));
#92339=CARTESIAN_POINT('Ctrl Pts',(-0.399999999999998,3.35784710386715,
0.459503349194265));
#92340=CARTESIAN_POINT('Ctrl Pts',(-0.399999999999998,3.35707420233503,
0.478950143980882));
#92341=CARTESIAN_POINT('Ctrl Pts',(-0.399999999999997,3.35614110588597,
0.498397914812365));
#92342=CARTESIAN_POINT('Ctrl Pts',(-0.399999999999997,3.35504815107657,
0.517844463495855));
#92343=CARTESIAN_POINT('Ctrl Pts',(-0.399999999999998,3.35409082912369,
0.534877745935509));
#92344=CARTESIAN_POINT('Ctrl Pts',(-0.399999999999992,3.35301137108497,
0.551900908779291));
#92345=CARTESIAN_POINT('Ctrl Pts',(-0.399999999999992,3.35181049692923,
0.568910960665313));
#92346=CARTESIAN_POINT('Ctrl Pts',(-0.399999999999994,3.34397265912955,
0.679931775801685));
#92347=CARTESIAN_POINT('Ctrl Pts',(-0.399999999999999,3.33096547612328,
0.790412525141181));
#92348=CARTESIAN_POINT('Ctrl Pts',(-0.399999999999999,3.31293843234414,
0.899937431786043));
#92349=CARTESIAN_POINT('Ctrl Pts',(-0.4,3.29463178445671,1.01116109804079));
#92350=CARTESIAN_POINT('Ctrl Pts',(-0.399999999999993,3.27114846169325,
1.12139992524088));
#92351=CARTESIAN_POINT('Ctrl Pts',(-0.399999999999994,3.24259365432844,
1.23023390508146));
#92352=CARTESIAN_POINT('Ctrl Pts',(-0.399999999999994,3.21411812812659,
1.33876571217816));
#92353=CARTESIAN_POINT('Ctrl Pts',(-0.399999999999998,3.18059920173942,
1.4459014170632));
#92354=CARTESIAN_POINT('Ctrl Pts',(-0.400000000000001,3.14209018890566,
1.5512257962275));
#92355=CARTESIAN_POINT('Ctrl Pts',(-0.400000000000002,3.11694027798415,
1.62001225838068));
#92356=CARTESIAN_POINT('Ctrl Pts',(-0.399999999999998,3.08966091557709,
1.68802613622077));
#92357=CARTESIAN_POINT('Ctrl Pts',(-0.399999999999997,3.06025526189474,
1.75514908035963));
#92358=CARTESIAN_POINT('Ctrl Pts',(-0.399999999999997,3.05164036528084,
1.77481391183808));
#92359=CARTESIAN_POINT('Ctrl Pts',(-0.399999999999994,3.04284290901892,
1.79440225257972));
#92360=CARTESIAN_POINT('Ctrl Pts',(-0.399999999999994,3.03386282258109,
1.81391106505042));
#92361=CARTESIAN_POINT('Ctrl Pts',(-0.399999999999994,3.02664727008747,
1.82958651109929));
#92362=CARTESIAN_POINT('Ctrl Pts',(-0.399999999999994,3.01931673828124,
1.84520414701729));
#92363=CARTESIAN_POINT('Ctrl Pts',(-0.399999999999994,3.01187496318844,
1.86075544310257));
#92364=CARTESIAN_POINT('Ctrl Pts',(-0.399999999999995,2.96187696416847,
1.96523773082757));
#92365=CARTESIAN_POINT('Ctrl Pts',(-0.39999999999999,2.90681611202108,2.06682489248903));
#92366=CARTESIAN_POINT('Ctrl Pts',(-0.399999999999992,2.84680781566502,
2.16508365912674));
#92367=CARTESIAN_POINT('Ctrl Pts',(-0.399999999999992,2.81303601982972,
2.22038226294357));
#92368=CARTESIAN_POINT('Ctrl Pts',(-0.399999999999999,2.77769628795341,
2.27462673936948));
#92369=CARTESIAN_POINT('Ctrl Pts',(-0.399999999999999,2.74080195646948,
2.32773919637629));
#92370=CARTESIAN_POINT('Ctrl Pts',(-0.399999999999999,2.67744566437209,
2.41894584533261));
#92371=CARTESIAN_POINT('Ctrl Pts',(-0.399999999999998,2.60950780329113,
2.50681584887859));
#92372=CARTESIAN_POINT('Ctrl Pts',(-0.399999999999997,2.53736550365763,
2.59125872319195));
#92373=CARTESIAN_POINT('Ctrl Pts',(-0.399999999999997,2.46387235100471,
2.67728277681779));
#92374=CARTESIAN_POINT('Ctrl Pts',(-0.400000000000003,2.38601536697427,
2.75975066336544));
#92375=CARTESIAN_POINT('Ctrl Pts',(-0.400000000000003,2.30414671759461,
2.83853907492399));
#92376=CARTESIAN_POINT('Ctrl Pts',(-0.400000000000003,2.27577470203401,
2.86584361769675));
#92377=CARTESIAN_POINT('Ctrl Pts',(-0.4,2.24692051240199,2.89270597751155));
#92378=CARTESIAN_POINT('Ctrl Pts',(-0.4,2.21759770087157,2.91912009175765));
#92379=CARTESIAN_POINT('Ctrl Pts',(-0.4,2.20688460243407,2.92877049672527));
#92380=CARTESIAN_POINT('Ctrl Pts',(-0.400000000000001,2.19610981880862,
2.93836022592291));
#92381=CARTESIAN_POINT('Ctrl Pts',(-0.400000000000001,2.18528158294958,
2.94788250838123));
#92382=CARTESIAN_POINT('Ctrl Pts',(-0.400000000000001,2.09969869901333,
3.02314355783082));
#92383=CARTESIAN_POINT('Ctrl Pts',(-0.399999999999996,2.01065587601546,
3.09430616390818));
#92384=CARTESIAN_POINT('Ctrl Pts',(-0.399999999999996,1.91856670100604,
3.16129393881534));
#92385=CARTESIAN_POINT('Ctrl Pts',(-0.399999999999996,1.8235125715356,3.23043848950015));
#92386=CARTESIAN_POINT('Ctrl Pts',(-0.399999999999996,1.72521235437322,
3.29513561360273));
#92387=CARTESIAN_POINT('Ctrl Pts',(-0.399999999999994,1.62407296298976,
3.35527343326626));
#92388=CARTESIAN_POINT('Ctrl Pts',(-0.399999999999991,1.52197936605142,
3.41597862673732));
#92389=CARTESIAN_POINT('Ctrl Pts',(-0.400000000000002,1.41699210619484,
3.47203860011689));
#92390=CARTESIAN_POINT('Ctrl Pts',(-0.400000000000002,1.30949015933882,
3.52330219657907));
#92391=CARTESIAN_POINT('Ctrl Pts',(-0.400000000000002,1.23934879114686,
3.55674995170775));
#92392=CARTESIAN_POINT('Ctrl Pts',(-0.400000000000001,1.16813610343819,
3.58815507998474));
#92393=CARTESIAN_POINT('Ctrl Pts',(-0.400000000000001,1.09595051685845,
3.61746580574807));
#92394=CARTESIAN_POINT('Ctrl Pts',(-0.400000000000001,1.05572480653037,
3.6337993263292));
#92395=CARTESIAN_POINT('Ctrl Pts',(-0.400000000000002,1.01519689475796,
3.64948232247901));
#92396=CARTESIAN_POINT('Ctrl Pts',(-0.400000000000002,0.974383269726773,
3.66450467150052));
#92397=CARTESIAN_POINT('Ctrl Pts',(-0.400000000000002,0.958753801871717,
3.67025743962537));
#92398=CARTESIAN_POINT('Ctrl Pts',(-0.399999999999996,0.943091728437667,
3.6759098874143));
#92399=CARTESIAN_POINT('Ctrl Pts',(-0.399999999999996,0.927399385258908,
3.68146132666716));
#92400=CARTESIAN_POINT('Ctrl Pts',(-0.399999999999996,0.811870525443297,
3.72233166960525));
#92401=CARTESIAN_POINT('Ctrl Pts',(-0.400000000000004,0.694682613315391,
3.75773824573158));
#92402=CARTESIAN_POINT('Ctrl Pts',(-0.400000000000003,0.576262045218899,
3.78756373718036));
#92403=CARTESIAN_POINT('Ctrl Pts',(-0.400000000000002,0.45763889427005,
3.81744025129545));
#92404=CARTESIAN_POINT('Ctrl Pts',(-0.400000000000002,0.337778087304372,
3.84171704650798));
#92405=CARTESIAN_POINT('Ctrl Pts',(-0.400000000000001,0.217075768755943,
3.86023502674498));
#92406=CARTESIAN_POINT('Ctrl Pts',(-0.4,0.0986485754491533,3.87840396046184));
#92407=CARTESIAN_POINT('Ctrl Pts',(-0.399999999999999,-0.0205895151206229,
3.89102943611732));
#92408=CARTESIAN_POINT('Ctrl Pts',(-0.399999999999998,-0.14028364083043,
3.89791601923602));
#92409=CARTESIAN_POINT('Ctrl Pts',(-0.399999999999997,-0.259694075762963,
3.90478628024948));
#92410=CARTESIAN_POINT('Ctrl Pts',(-0.4,-0.379559128612082,3.90594525600568));
#92411=CARTESIAN_POINT('Ctrl Pts',(-0.4,-0.499534418911701,3.90114782651498));
#92412=CARTESIAN_POINT('',(-0.4,-4.81653586104654E-16,3.933));
#92413=CARTESIAN_POINT('Origin',(-0.4,0.,0.));
#92414=CARTESIAN_POINT('',(-0.40000000000001,-3.41554413377521,1.96277079485755));
#92415=CARTESIAN_POINT('Origin',(-0.4,0.,0.));
#92416=CARTESIAN_POINT('Ctrl Pts',(-0.399999999999993,-3.41555626699905,
1.96277456084997));
#92417=CARTESIAN_POINT('Ctrl Pts',(-0.399999999999994,-3.45586581128785,
1.87693662981294));
#92418=CARTESIAN_POINT('Ctrl Pts',(-0.4,-3.49279526202284,1.78967478039338));
#92419=CARTESIAN_POINT('Ctrl Pts',(-0.400000000000001,-3.52617474615515,
1.70109144698049));
#92420=CARTESIAN_POINT('Ctrl Pts',(-0.400000000000002,-3.56906103703463,
1.58727870533473));
#92421=CARTESIAN_POINT('Ctrl Pts',(-0.399999999999999,-3.60608888168847,
1.4712842047269));
#92422=CARTESIAN_POINT('Ctrl Pts',(-0.400000000000001,-3.63733134408434,
1.3535520921038));
#92423=CARTESIAN_POINT('Ctrl Pts',(-0.400000000000001,-3.65528841060761,
1.28588382218609));
#92424=CARTESIAN_POINT('Ctrl Pts',(-0.400000000000002,-3.67133327041293,
1.2176413971065));
#92425=CARTESIAN_POINT('Ctrl Pts',(-0.400000000000004,-3.68547211562788,
1.14890933338331));
#92426=CARTESIAN_POINT('Ctrl Pts',(-0.400000000000005,-3.69433691436354,
1.10581557980372));
#92427=CARTESIAN_POINT('Ctrl Pts',(-0.400000000000003,-3.70245233702665,
1.06252935589371));
#92428=CARTESIAN_POINT('Ctrl Pts',(-0.400000000000002,-3.70981882690422,
1.0190717129688));
#92429=CARTESIAN_POINT('Ctrl Pts',(-0.400000000000002,-3.71320117185905,
0.999118011580692));
#92430=CARTESIAN_POINT('Ctrl Pts',(-0.400000000000009,-3.71642544923357,
0.979128724847171));
#92431=CARTESIAN_POINT('Ctrl Pts',(-0.400000000000009,-3.71948985922468,
0.959119148092641));
#92432=CARTESIAN_POINT('Ctrl Pts',(-0.40000000000001,-3.73823141925564,
0.83674300226789));
#92433=CARTESIAN_POINT('Ctrl Pts',(-0.400000000000023,-3.75102036592465,
0.713479450781438));
#92434=CARTESIAN_POINT('Ctrl Pts',(-0.400000000000019,-3.75793544512979,
0.58979761469609));
#92435=CARTESIAN_POINT('Ctrl Pts',(-0.400000000000016,-3.76398613943429,
0.481576008121411));
#92436=CARTESIAN_POINT('Ctrl Pts',(-0.400000000000006,-3.76553866286515,
0.373033640931303));
#92437=CARTESIAN_POINT('Ctrl Pts',(-0.400000000000004,-3.76261070624249,
0.264490932332908));
#92438=CARTESIAN_POINT('Ctrl Pts',(-0.400000000000003,-3.76132972522008,
0.21700349732111));
#92439=CARTESIAN_POINT('Ctrl Pts',(-0.400000000000014,-3.75919074263992,
0.169516123263878));
#92440=CARTESIAN_POINT('Ctrl Pts',(-0.400000000000015,-3.75619336846896,
0.122056406365339));
#92441=CARTESIAN_POINT('Ctrl Pts',(-0.400000000000015,-3.7544301202536,
0.0941375492758329));
#92442=CARTESIAN_POINT('Ctrl Pts',(-0.400000000000005,-3.75236980031072,
0.0662282734061994));
#92443=CARTESIAN_POINT('Ctrl Pts',(-0.400000000000004,-3.75001215099025,
0.0383342975575875));
#92444=CARTESIAN_POINT('Ctrl Pts',(-0.400000000000004,-3.74818369217564,
0.0167013152595263));
#92445=CARTESIAN_POINT('Ctrl Pts',(-0.400000000000019,-3.74617606664209,
-0.0049248646594703));
#92446=CARTESIAN_POINT('Ctrl Pts',(-0.400000000000019,-3.74399167965982,
-0.0265186312542417));
#92447=CARTESIAN_POINT('Ctrl Pts',(-0.400000000000018,-3.7320274191325,
-0.144791378438078));
#92448=CARTESIAN_POINT('Ctrl Pts',(-0.400000000000008,-3.71475353950831,
-0.262239439074446));
#92449=CARTESIAN_POINT('Ctrl Pts',(-0.400000000000008,-3.69223626798488,
-0.378452392337834));
#92450=CARTESIAN_POINT('Ctrl Pts',(-0.400000000000008,-3.66987919815232,
-0.4938385353194));
#92451=CARTESIAN_POINT('Ctrl Pts',(-0.400000000000015,-3.64235278957465,
-0.608007931120418));
#92452=CARTESIAN_POINT('Ctrl Pts',(-0.400000000000015,-3.6096739605563,
-0.720541241088965));
#92453=CARTESIAN_POINT('Ctrl Pts',(-0.400000000000015,-3.57795867401629,
-0.829756481602768));
#92454=CARTESIAN_POINT('Ctrl Pts',(-0.400000000000005,-3.54138992891154,
-0.937431313648108));
#92455=CARTESIAN_POINT('Ctrl Pts',(-0.400000000000006,-3.49994321149449,
-1.04315520271956));
#92456=CARTESIAN_POINT('Ctrl Pts',(-0.400000000000006,-3.4716806339255,
-1.11524847818238));
#92457=CARTESIAN_POINT('Ctrl Pts',(-0.400000000000003,-3.44114903570196,
-1.18643402337789));
#92458=CARTESIAN_POINT('Ctrl Pts',(-0.400000000000003,-3.40833081899823,
-1.25657189330865));
#92459=CARTESIAN_POINT('Ctrl Pts',(-0.400000000000003,-3.39794175690299,
-1.2787750097216));
#92460=CARTESIAN_POINT('Ctrl Pts',(-0.400000000000002,-3.38732348880224,
-1.3008730681313));
#92461=CARTESIAN_POINT('Ctrl Pts',(-0.400000000000002,-3.3764752978588,
-1.32286143260974));
#92462=CARTESIAN_POINT('Ctrl Pts',(-0.400000000000002,-3.36937925489342,
-1.33724451084749));
#92463=CARTESIAN_POINT('Ctrl Pts',(-0.400000000000004,-3.36218359172965,
-1.3515830717022));
#92464=CARTESIAN_POINT('Ctrl Pts',(-0.400000000000004,-3.35489225176958,
-1.36586767082509));
#92465=CARTESIAN_POINT('Ctrl Pts',(-0.400000000000006,-3.30395288020021,
-1.4656639368647));
#92466=CARTESIAN_POINT('Ctrl Pts',(-0.400000000000003,-3.24844027608969,
-1.56265069548797));
#92467=CARTESIAN_POINT('Ctrl Pts',(-0.400000000000004,-3.18837281836721,
-1.65645757823181));
#92468=CARTESIAN_POINT('Ctrl Pts',(-0.400000000000005,-3.14561797202901,
-1.72322749008171));
#92469=CARTESIAN_POINT('Ctrl Pts',(-0.400000000000004,-3.10055458235714,
-1.78838591080347));
#92470=CARTESIAN_POINT('Ctrl Pts',(-0.400000000000004,-3.05317683241366,
-1.85178896301253));
#92471=CARTESIAN_POINT('Ctrl Pts',(-0.400000000000004,-2.98537511675161,
-1.94252429179267));
#92472=CARTESIAN_POINT('Ctrl Pts',(-0.40000000000001,-2.91283434670415,
-2.02966653669181));
#92473=CARTESIAN_POINT('Ctrl Pts',(-0.400000000000008,-2.83593089936814,
-2.11303626961663));
#92474=CARTESIAN_POINT('Ctrl Pts',(-0.400000000000005,-2.75873941564364,
-2.19671825794237));
#92475=CARTESIAN_POINT('Ctrl Pts',(-0.400000000000014,-2.67715161752483,
-2.27659978388866));
#92476=CARTESIAN_POINT('Ctrl Pts',(-0.400000000000015,-2.59152627560853,
-2.35245214060421));
#92477=CARTESIAN_POINT('Ctrl Pts',(-0.400000000000015,-2.57282073634438,
-2.36902269325915));
#92478=CARTESIAN_POINT('Ctrl Pts',(-0.400000000000002,-2.55392245661421,
-2.3854007680765));
#92479=CARTESIAN_POINT('Ctrl Pts',(-0.400000000000002,-2.53483510403623,
-2.40158365556471));
#92480=CARTESIAN_POINT('Ctrl Pts',(-0.400000000000002,-2.51820440401829,
-2.4156837119314));
#92481=CARTESIAN_POINT('Ctrl Pts',(-0.400000000000011,-2.50142627206165,
-2.42963864398316));
#92482=CARTESIAN_POINT('Ctrl Pts',(-0.400000000000011,-2.48452672290024,
-2.44342770418704));
#92483=CARTESIAN_POINT('Ctrl Pts',(-0.400000000000008,-2.39827220288853,
-2.51380643192344));
#92484=CARTESIAN_POINT('Ctrl Pts',(-0.400000000000015,-2.30875623932578,
-2.57995647049072));
#92485=CARTESIAN_POINT('Ctrl Pts',(-0.400000000000014,-2.21635638722814,
-2.64173828957315));
#92486=CARTESIAN_POINT('Ctrl Pts',(-0.400000000000013,-2.1238561535402,
-2.703587227348));
#92487=CARTESIAN_POINT('Ctrl Pts',(-0.400000000000001,-2.02846485802401,
-2.76105874771976));
#92488=CARTESIAN_POINT('Ctrl Pts',(-0.400000000000003,-1.93053914104806,
-2.81396554239287));
#92489=CARTESIAN_POINT('Ctrl Pts',(-0.400000000000004,-1.83380515901436,
-2.86622847273859));
#92490=CARTESIAN_POINT('Ctrl Pts',(-0.400000000000014,-1.73459720535212,
-2.91403727878679));
#92491=CARTESIAN_POINT('Ctrl Pts',(-0.400000000000016,-1.6332506304093,
-2.95716191024929));
#92492=CARTESIAN_POINT('Ctrl Pts',(-0.400000000000017,-1.57298067615276,
-2.98280776524775));
#92493=CARTESIAN_POINT('Ctrl Pts',(-0.400000000000011,-1.51195428265001,
-3.0067960672628));
#92494=CARTESIAN_POINT('Ctrl Pts',(-0.400000000000011,-1.45024239915814,
-3.02906958386214));
#92495=CARTESIAN_POINT('Ctrl Pts',(-0.400000000000012,-1.42096324775188,
-3.0396372351468));
#92496=CARTESIAN_POINT('Ctrl Pts',(-0.40000000000001,-1.39152980408315,
-3.04981878609203));
#92497=CARTESIAN_POINT('Ctrl Pts',(-0.40000000000001,-1.36194974487981,
-3.05960757992356));
#92498=CARTESIAN_POINT('Ctrl Pts',(-0.40000000000001,-1.34596495330587,
-3.06489735395956));
#92499=CARTESIAN_POINT('Ctrl Pts',(-0.40000000000001,-1.32994425166988,
-3.07007010522677));
#92500=CARTESIAN_POINT('Ctrl Pts',(-0.40000000000001,-1.31389608522276,
-3.07512291332643));
#92501=CARTESIAN_POINT('Ctrl Pts',(-0.400000000000011,-1.21135478554361,
-3.10740831560437));
#92502=CARTESIAN_POINT('Ctrl Pts',(-0.400000000000022,-1.10760140379211,
-3.13483125191197));
#92503=CARTESIAN_POINT('Ctrl Pts',(-0.40000000000002,-1.00295989448995,
-3.15722300264388));
#92504=CARTESIAN_POINT('Ctrl Pts',(-0.400000000000018,-0.899785788764044,
-3.17930075049756));
#92505=CARTESIAN_POINT('Ctrl Pts',(-0.400000000000015,-0.795747515823994,
-3.1964875260079));
#92506=CARTESIAN_POINT('Ctrl Pts',(-0.400000000000016,-0.691154690506712,
-3.20857188447556));
#92507=CARTESIAN_POINT('Ctrl Pts',(-0.400000000000016,-0.589773280006148,
-3.22028520518115));
#92508=CARTESIAN_POINT('Ctrl Pts',(-0.400000000000013,-0.48787023799748,
-3.2272045644463));
#92509=CARTESIAN_POINT('Ctrl Pts',(-0.400000000000014,-0.385736684885698,
-3.22909034216834));
#92510=CARTESIAN_POINT('Ctrl Pts',(-0.400000000000014,-0.29114362765779,
-3.23083689337062));
#92511=CARTESIAN_POINT('Ctrl Pts',(-0.40000000000001,-0.196352551596845,
-3.22826531799378));
#92512=CARTESIAN_POINT('Ctrl Pts',(-0.40000000000001,-0.101608697681888,
-3.22114781328883));
#92513=CARTESIAN_POINT('Ctrl Pts',(-29.6770630286919,-1.43290239521317,
2.8866777250487));
#92514=CARTESIAN_POINT('Ctrl Pts',(-29.6111236975462,-2.38968372905088,
2.41174619630378));
#92515=CARTESIAN_POINT('Ctrl Pts',(-29.4792450352548,-3.77781470893137,
0.444337671635494));
#92516=CARTESIAN_POINT('Ctrl Pts',(-29.2814270418177,-2.42921825930742,
-2.93180374517478));
#92517=CARTESIAN_POINT('Ctrl Pts',(-29.0836090483806,1.13283940936973,-3.63131203549138));
#92518=CARTESIAN_POINT('Ctrl Pts',(-28.8857910549435,3.66252655955179,-1.03121985822236));
#92519=CARTESIAN_POINT('Ctrl Pts',(-28.6879730615064,2.8605553688775,2.50949297218581));
#92520=CARTESIAN_POINT('Ctrl Pts',(-28.4901550680693,-0.544644508144919,
3.76563167765424));
#92521=CARTESIAN_POINT('Ctrl Pts',(-28.2923370746322,-3.45404918098007,
1.59609170665207));
#92522=CARTESIAN_POINT('Ctrl Pts',(-28.0945190811951,-3.22076798380931,
-2.02604665891755));
#92523=CARTESIAN_POINT('Ctrl Pts',(-27.896701087758,-0.056879441065127,
-3.80453263781198));
#92524=CARTESIAN_POINT('Ctrl Pts',(-27.6988830943209,3.15873057113267,-2.12140205749341));
#92525=CARTESIAN_POINT('Ctrl Pts',(-27.5010651008837,3.50025983817255,1.49201838676206));
#92526=CARTESIAN_POINT('Ctrl Pts',(-27.3032471074467,0.656928350055686,
3.74784144106381));
#92527=CARTESIAN_POINT('Ctrl Pts',(-27.1054291140095,-2.78413111524294,
2.59355341701617));
#92528=CARTESIAN_POINT('Ctrl Pts',(-26.9076111205725,-3.69193959240583,
-0.920589964011001));
#92529=CARTESIAN_POINT('Ctrl Pts',(-26.7097931271353,-1.24048741938786,
-3.59709412115127));
#92530=CARTESIAN_POINT('Ctrl Pts',(-26.5119751336982,2.33967134712765,-3.0006396835025));
#92531=CARTESIAN_POINT('Ctrl Pts',(-26.3141571402611,3.79098660083381,0.326068132244285));
#92532=CARTESIAN_POINT('Ctrl Pts',(-26.116339146824,1.79292039549545,3.35608927428751));
#92533=CARTESIAN_POINT('Ctrl Pts',(-25.9185211533869,-1.83650628133122,
3.33243818231883));
#92534=CARTESIAN_POINT('Ctrl Pts',(-25.7207031599498,-3.79491407443894,
0.276634354159837));
#92535=CARTESIAN_POINT('Ctrl Pts',(-25.5228851665127,-2.30036699385748,
-3.03087627035208));
#92536=CARTESIAN_POINT('Ctrl Pts',(-25.3250671730756,1.28726128874941,-3.58062253845296));
#92537=CARTESIAN_POINT('Ctrl Pts',(-25.1272491796384,3.70362324127845,-0.872395691996212));
#92538=CARTESIAN_POINT('Ctrl Pts',(-24.9294311862013,2.750094969933,2.62961537102403));
#92539=CARTESIAN_POINT('Ctrl Pts',(-24.7316131927642,-0.705717560089592,
3.7389653762666));
#92540=CARTESIAN_POINT('Ctrl Pts',(-24.5337951993271,-3.51940465095792,
1.44626769885165));
#92541=CARTESIAN_POINT('Ctrl Pts',(-24.33597720589,-3.13082019758146,-2.16237467684802));
#92542=CARTESIAN_POINT('Ctrl Pts',(-24.1381592124529,0.106466641732784,
-3.80349368464174));
#92543=CARTESIAN_POINT('Ctrl Pts',(-23.9403412190158,3.2468805350555,-1.98385134146986));
#92544=CARTESIAN_POINT('Ctrl Pts',(-23.7425232255787,3.43298988692531,1.64087774991356));
#92545=CARTESIAN_POINT('Ctrl Pts',(-23.5447052321416,0.495455635705227,
3.77258837765834));
#92546=CARTESIAN_POINT('Ctrl Pts',(-23.3468872387045,-2.89288880667469,
2.47165808846236));
#92547=CARTESIAN_POINT('Ctrl Pts',(-23.1490692452673,-3.64902228624806,
-1.0782094919416));
#92548=CARTESIAN_POINT('Ctrl Pts',(-22.9512512518303,-1.08494641550995,
-3.6470249011433));
#92549=CARTESIAN_POINT('Ctrl Pts',(-22.7534332583931,2.46631148668775,-2.89744836100596));
#92550=CARTESIAN_POINT('Ctrl Pts',(-22.555615264956,3.77349691781262,0.488487835391227));
#92551=CARTESIAN_POINT('Ctrl Pts',(-22.357797271519,1.64721476033769,3.42995377336155));
#92552=CARTESIAN_POINT('Ctrl Pts',(-22.1599792780818,-1.97785184410161,
3.25053863795708));
#92553=CARTESIAN_POINT('Ctrl Pts',(-21.9621612846447,-3.80329058354344,
0.113490489462255));
#92554=CARTESIAN_POINT('Ctrl Pts',(-21.7643432912076,-2.16815277209852,
-3.12682153486743));
#92555=CARTESIAN_POINT('Ctrl Pts',(-21.5665252977705,1.43976583982743,-3.52206951670956));
#92556=CARTESIAN_POINT('Ctrl Pts',(-21.3687073043334,3.7376557293535,-0.712621219793359));
#92557=CARTESIAN_POINT('Ctrl Pts',(-21.1708893108963,2.63468957378667,2.74523408908033));
#92558=CARTESIAN_POINT('Ctrl Pts',(-20.9730713174592,-0.865554611853212,
3.70522800485591));
#92559=CARTESIAN_POINT('Ctrl Pts',(-20.7752533240221,-3.57823920205966,
1.29387154188981));
#92560=CARTESIAN_POINT('Ctrl Pts',(-20.577435330585,-3.03511927138851,-2.2947658622428));
#92561=CARTESIAN_POINT('Ctrl Pts',(-20.3796173371479,0.269625717635743,
-3.79541846526285));
#92562=CARTESIAN_POINT('Ctrl Pts',(-20.1817993437108,3.3290409282824,-1.84265728009565));
#92563=CARTESIAN_POINT('Ctrl Pts',(-19.9839813502737,3.35939466694879,1.78671957109805));
#92564=CARTESIAN_POINT('Ctrl Pts',(-19.7861633568365,0.333068366514352,
3.79037792539165));
#92565=CARTESIAN_POINT('Ctrl Pts',(-19.5883453633995,-2.99631355212319,
2.34520882895996));
#92566=CARTESIAN_POINT('Ctrl Pts',(-19.3905273699623,-3.59937935322612,
-1.23384262596099));
#92567=CARTESIAN_POINT('Ctrl Pts',(-19.1927093765252,-0.927405418628458,
-3.69023285763479));
#92568=CARTESIAN_POINT('Ctrl Pts',(-18.9948913830881,2.58840554981504,-2.78891664697164));
#92569=CARTESIAN_POINT('Ctrl Pts',(-18.797073389651,3.74905186462063,0.650007284923323));
#92570=CARTESIAN_POINT('Ctrl Pts',(-18.5992553962139,1.49847290337135,3.4974960059921));
#92571=CARTESIAN_POINT('Ctrl Pts',(-18.4014374027768,-2.11555175776316,
3.16264764308231));
#92572=CARTESIAN_POINT('Ctrl Pts',(-18.2036194093397,-3.80465676201416,
-0.0498625844572021));
#92573=CARTESIAN_POINT('Ctrl Pts',(-18.0058014159026,-2.03194214307649,
-3.21700333870802));
#92574=CARTESIAN_POINT('Ctrl Pts',(-17.8079834224654,1.5896165698452,-3.45702451755008));
#92575=CARTESIAN_POINT('Ctrl Pts',(-17.6101654290284,3.76479886064709,-0.551533220159296));
#92576=CARTESIAN_POINT('Ctrl Pts',(-17.4123474355912,2.51442783918464,2.85579270879419));
#92577=CARTESIAN_POINT('Ctrl Pts',(-17.2145294421542,-1.0237962474182,3.66466104815183));
#92578=CARTESIAN_POINT('Ctrl Pts',(-17.016711448717,-3.6304782367563,1.13909048214257));
#92579=CARTESIAN_POINT('Ctrl Pts',(-16.8188934552799,-2.93382392331867,
-2.42292726697108));
#92580=CARTESIAN_POINT('Ctrl Pts',(-16.6210754618428,0.432287811384032,
-3.7803474181876));
#92581=CARTESIAN_POINT('Ctrl Pts',(-16.4232574684057,3.40506513462136,-1.69806677814945));
#92582=CARTESIAN_POINT('Ctrl Pts',(-16.2254394749686,3.27960731114141,1.92926805778166));
#92583=CARTESIAN_POINT('Ctrl Pts',(-16.0276214815315,0.170067175844205,
3.80118093620512));
#92584=CARTESIAN_POINT('Ctrl Pts',(-15.8298034880944,-3.09421540362715,
2.21443681102563));
#92585=CARTESIAN_POINT('Ctrl Pts',(-15.6319854946573,-3.54310193749609,
-1.38720150467778));
#92586=CARTESIAN_POINT('Ctrl Pts',(-15.4341675012202,-0.768155000592636,
-3.72663886754987));
#92587=CARTESIAN_POINT('Ctrl Pts',(-15.236349507783,2.70572858711511,-2.67524431911123));
#92588=CARTESIAN_POINT('Ctrl Pts',(-15.038531514346,3.71769644791273,0.81032862176155));
#92589=CARTESIAN_POINT('Ctrl Pts',(-14.8407135209088,1.34696901673613,3.5585915503218));
#92590=CARTESIAN_POINT('Ctrl Pts',(-14.6428955274718,-2.24935222372163,
3.06892716233335));
#92591=CARTESIAN_POINT('Ctrl Pts',(-14.4450775340346,-3.79901008437419,
-0.213123750183017));
#92592=CARTESIAN_POINT('Ctrl Pts',(-14.2472595405976,-1.89198617807126,
-3.3012554666454));
#92593=CARTESIAN_POINT('Ctrl Pts',(-14.0494415471604,1.73653727148651,-3.38560742833646));
#92594=CARTESIAN_POINT('Ctrl Pts',(-13.8516235537233,3.78500260309515,-0.389428618146851));
#92595=CARTESIAN_POINT('Ctrl Pts',(-13.6538055602862,2.38953143666386,2.96108744674385));
#92596=CARTESIAN_POINT('Ctrl Pts',(-13.4559875668491,-1.18015079139549,
3.61733927958623));
#92597=CARTESIAN_POINT('Ctrl Pts',(-13.258169573412,-3.67602546636253,0.982209817056931));
#92598=CARTESIAN_POINT('Ctrl Pts',(-13.0603515799749,-2.82712086403723,
-2.54662266034728));
#92599=CARTESIAN_POINT('Ctrl Pts',(-12.8625335865378,0.594153099425664,
-3.75830832270474));
#92600=CARTESIAN_POINT('Ctrl Pts',(-12.6647155931007,3.47481302398082,-1.55034634918851));
#92601=CARTESIAN_POINT('Ctrl Pts',(-12.4668975996636,3.19377488593328,2.0682604603992));
#92602=CARTESIAN_POINT('Ctrl Pts',(-12.2690796062265,0.00675251231494511,
3.80497749765308));
#92603=CARTESIAN_POINT('Ctrl Pts',(-12.0712616127893,-3.18641390558911,
2.07958307752715));
#92604=CARTESIAN_POINT('Ctrl Pts',(-11.8734436193523,-3.48029377126023,
-1.53800345246562));
#92605=CARTESIAN_POINT('Ctrl Pts',(-11.6756256259151,-0.607488696492234,
-3.75617582624975));
#92606=CARTESIAN_POINT('Ctrl Pts',(-11.477807632478,2.81806434528784,-2.55664090162977));
#92607=CARTESIAN_POINT('Ctrl Pts',(-11.2799896390409,3.67948846292253,0.969156336866661));
#92608=CARTESIAN_POINT('Ctrl Pts',(-11.0821716456038,1.1929823568862,3.61312779323221));
#92609=CARTESIAN_POINT('Ctrl Pts',(-10.8843536521667,-2.37900661699238,
2.96954994407828));
#92610=CARTESIAN_POINT('Ctrl Pts',(-10.6865356587296,-3.78636095874714,
-0.37599207989568));
#92611=CARTESIAN_POINT('Ctrl Pts',(-10.4887176652925,-1.74854284806569,
-3.37942262266014));
#92612=CARTESIAN_POINT('Ctrl Pts',(-10.2908996718554,1.88025713615946,-3.30794988716429));
#92613=CARTESIAN_POINT('Ctrl Pts',(-10.0930816784183,3.79822971656082,-0.226606209763087));
#92614=CARTESIAN_POINT('Ctrl Pts',(-9.89526368498117,2.26023057897525,3.06092422054745));
#92615=CARTESIAN_POINT('Ctrl Pts',(-9.69744569154406,-1.33433004645538,
3.56334992404553));
#92616=CARTESIAN_POINT('Ctrl Pts',(-9.49962769810695,-3.71479693687478,
0.823518713724579));
#92617=CARTESIAN_POINT('Ctrl Pts',(-9.30180970466985,-2.71520677178563,
-2.66562404335614));
#92618=CARTESIAN_POINT('Ctrl Pts',(-9.10399171123273,0.754923226864277,
-3.72934180192827));
#92619=CARTESIAN_POINT('Ctrl Pts',(-8.90617371779564,3.53815603498388,-1.3997682758857));
#92620=CARTESIAN_POINT('Ctrl Pts',(-8.70835572435851,3.10205560019449,2.20344058403463));
#92621=CARTESIAN_POINT('Ctrl Pts',(-8.51053773092143,-0.156574597645193,
3.80176061180093));
#92622=CARTESIAN_POINT('Ctrl Pts',(-8.3127197374843,-3.27273911499761,1.94089619486303));
#92623=CARTESIAN_POINT('Ctrl Pts',(-8.11490174404721,-3.41107062439205,
-1.68597050670474));
#92624=CARTESIAN_POINT('Ctrl Pts',(-7.91708375061009,-0.445702651221169,
-3.77878929033658));
#92625=CARTESIAN_POINT('Ctrl Pts',(-7.71926575717298,2.92520576373441,-2.43332500786197));
#92626=CARTESIAN_POINT('Ctrl Pts',(-7.52144776373588,3.63449833574001,1.12619767428708));
#92627=CARTESIAN_POINT('Ctrl Pts',(-7.32362977029877,1.03679675659798,3.66100421190307));
#92628=CARTESIAN_POINT('Ctrl Pts',(-7.12581177686167,-2.50427595475653,
2.86469916335302));
#92629=CARTESIAN_POINT('Ctrl Pts',(-6.92799378342455,-3.76673270037306,
-0.538167369865845));
#92630=CARTESIAN_POINT('Ctrl Pts',(-6.73017578998745,-1.60187655206341,
-3.45136072672716));
#92631=CARTESIAN_POINT('Ctrl Pts',(-6.53235779655034,2.02051125516165,-3.22419503472727));
#92632=CARTESIAN_POINT('Ctrl Pts',(-6.33453980311323,3.80445582041375,-0.0633661140739026));
#92633=CARTESIAN_POINT('Ctrl Pts',(-6.13672180967612,2.12676359733563,3.1551190080601));
#92634=CARTESIAN_POINT('Ctrl Pts',(-5.93890381623902,-1.48604982490852,
3.50279249639495));
#92635=CARTESIAN_POINT('Ctrl Pts',(-5.74108582280191,-3.74672118340988,
0.66330967612812));
#92636=CARTESIAN_POINT('Ctrl Pts',(-5.5432678293648,-2.59828793024122,-2.77971206881013));
#92637=CARTESIAN_POINT('Ctrl Pts',(-5.34544983592769,0.914301858020527,
-3.69350124840367));
#92638=CARTESIAN_POINT('Ctrl Pts',(-5.14763184249059,3.59497741079579,-1.24661010706821));
#92639=CARTESIAN_POINT('Ctrl Pts',(-4.94981384905348,3.00461851577406,2.33455925849379));
#92640=CARTESIAN_POINT('Ctrl Pts',(-4.75199585561637,-0.319613108768782,
3.79153621228826));
#92641=CARTESIAN_POINT('Ctrl Pts',(-4.55417786217927,-3.35303190681402,
1.79863178680334));
#92642=CARTESIAN_POINT('Ctrl Pts',(-4.35635986874215,-3.33556010608343,
-1.83082991481484));
#92643=CARTESIAN_POINT('Ctrl Pts',(-4.15854187530505,-0.283095044828532,
-3.79443760733249));
#92644=CARTESIAN_POINT('Ctrl Pts',(-3.96072388186794,3.02695530111143,-2.30552388116989));
#92645=CARTESIAN_POINT('Ctrl Pts',(-3.76290588843083,3.58280909899496,1.28116306328493));
#92646=CARTESIAN_POINT('Ctrl Pts',(-3.56508789499372,0.878699899841087,
3.70213276488018));
#92647=CARTESIAN_POINT('Ctrl Pts',(-3.36726990155662,-2.62492895022921,
2.75456769027902));
#92648=CARTESIAN_POINT('Ctrl Pts',(-3.1694519081195,-3.74016222880254,-0.699349939622732));
#92649=CARTESIAN_POINT('Ctrl Pts',(-2.9716339146824,-1.45225621275822,-3.51693862418514));
#92650=CARTESIAN_POINT('Ctrl Pts',(-2.7738159212453,2.15703839529281,-3.13449448646742));
#92651=CARTESIAN_POINT('Ctrl Pts',(-2.57599792780818,3.80367463162103,0.0999854885590033));
#92652=CARTESIAN_POINT('Ctrl Pts',(-2.37817993437108,1.98936656034495,3.24350831648798));
#92653=CARTESIAN_POINT('Ctrl Pts',(-2.18036194093398,-1.63501143994855,
3.43575922529938));
#92654=CARTESIAN_POINT('Ctrl Pts',(-1.98254394749686,-3.77177579799328,
0.501915131585207));
#92655=CARTESIAN_POINT('Ctrl Pts',(-1.78472595405976,-2.47651009463211,
-2.88874751957624));
#92656=CARTESIAN_POINT('Ctrl Pts',(-1.58690796062265,1.07186168277273,-3.65071665635791));
#92657=CARTESIAN_POINT('Ctrl Pts',(-1.38908996718554,3.64542809306271,-1.09141468478898));
#92658=CARTESIAN_POINT('Ctrl Pts',(-1.19127197374844,2.90115349698225,2.46187399806776));
#92659=CARTESIAN_POINT('Ctrl Pts',(-0.993453980311327,-0.481122552182907,
3.77336366075504));
#92660=CARTESIAN_POINT('Ctrl Pts',(-0.795635986874217,-3.42896535177265,
1.65492331179306));
#92661=CARTESIAN_POINT('Ctrl Pts',(-0.597817993437111,-3.25022050800311,
-1.97620509836622));
#92662=CARTESIAN_POINT('Ctrl Pts',(-0.465939331145708,-1.16924921554908,
-3.18746989196983));
#92663=CARTESIAN_POINT('Ctrl Pts',(-0.400000000000005,-0.101608697681796,
-3.22114781328883));
#92664=CARTESIAN_POINT('Ctrl Pts',(-29.5403753524613,-1.53816642191916,
3.09873914818276));
#92665=CARTESIAN_POINT('Ctrl Pts',(-29.4744360213156,-2.5652349268952,2.5889181494416));
#92666=CARTESIAN_POINT('Ctrl Pts',(-29.3425573590242,-4.05534093105207,
0.47697965247785));
#92667=CARTESIAN_POINT('Ctrl Pts',(-29.144739365587,-2.60767374697821,-3.14718022075313));
#92668=CARTESIAN_POINT('Ctrl Pts',(-28.94692137215,1.2160601773996,-3.89807586278254));
#92669=CARTESIAN_POINT('Ctrl Pts',(-28.7491033787128,3.93158347149777,-1.10697544008076));
#92670=CARTESIAN_POINT('Ctrl Pts',(-28.5512853852758,3.07069778873066,2.69384560927059));
#92671=CARTESIAN_POINT('Ctrl Pts',(-28.3534673918386,-0.584655240377733,
4.04226290864784));
#92672=CARTESIAN_POINT('Ctrl Pts',(-28.1556493984016,-3.7077909057794,1.71334396374614));
#92673=CARTESIAN_POINT('Ctrl Pts',(-27.9578314049644,-3.45737238072711,
-2.17488431200846));
#92674=CARTESIAN_POINT('Ctrl Pts',(-27.7600134115274,-0.0610579245566097,
-4.0840216152387));
#92675=CARTESIAN_POINT('Ctrl Pts',(-27.5621954180902,3.39077756910511,-2.2772447189197));
#92676=CARTESIAN_POINT('Ctrl Pts',(-27.3643774246531,3.7573962951386,1.60162519866677));
#92677=CARTESIAN_POINT('Ctrl Pts',(-27.1665594312159,0.705187689711472,
4.02316576382289));
#92678=CARTESIAN_POINT('Ctrl Pts',(-26.9687414377789,-2.98865924852468,
2.78408131135441));
#92679=CARTESIAN_POINT('Ctrl Pts',(-26.7709234443418,-3.96315724766984,
-0.988218440926554));
#92680=CARTESIAN_POINT('Ctrl Pts',(-26.5731054509047,-1.33161623686985,
-3.86134422841449));
#92681=CARTESIAN_POINT('Ctrl Pts',(-26.3752874574675,2.51154853010259,-3.22107299203379));
#92682=CARTESIAN_POINT('Ctrl Pts',(-26.1774694640305,4.06948045786504,0.3500217837248));
#92683=CARTESIAN_POINT('Ctrl Pts',(-25.9796514705934,1.92463210246421,3.60263465810181));
#92684=CARTESIAN_POINT('Ctrl Pts',(-25.7818334771562,-1.97141989923679,
3.57724610712342));
#92685=CARTESIAN_POINT('Ctrl Pts',(-25.5840154837191,-4.07369645194989,
0.296956496227123));
#92686=CARTESIAN_POINT('Ctrl Pts',(-25.386197490282,-2.46935679629198,-3.25353082221178));
#92687=CARTESIAN_POINT('Ctrl Pts',(-25.1883794968449,1.38182621314983,-3.8436626085728));
#92688=CARTESIAN_POINT('Ctrl Pts',(-24.9905615034078,3.97569920198674,-0.936483716224004));
#92689=CARTESIAN_POINT('Ctrl Pts',(-24.7927435099707,2.95212273632246,2.82279245242654));
#92690=CARTESIAN_POINT('Ctrl Pts',(-24.5949255165336,-0.757561057832579,
4.01363764461851));
#92691=CARTESIAN_POINT('Ctrl Pts',(-24.3971075230965,-3.77794752617762,
1.55251356890149));
#92692=CARTESIAN_POINT('Ctrl Pts',(-24.1992895296594,-3.36081684075186,
-2.32122727315359));
#92693=CARTESIAN_POINT('Ctrl Pts',(-24.0014715362223,0.114287905383463,
-4.08290633838123));
#92694=CARTESIAN_POINT('Ctrl Pts',(-23.8036535427852,3.48540321496378,-2.12958923770538));
#92695=CARTESIAN_POINT('Ctrl Pts',(-23.605835549348,3.6851845516463,1.76142008403567));
#92696=CARTESIAN_POINT('Ctrl Pts',(-23.408017555911,0.53185284980909,4.0497306624805));
#92697=CARTESIAN_POINT('Ctrl Pts',(-23.2101995624738,-3.10540650894146,
2.65323129533334));
#92698=CARTESIAN_POINT('Ctrl Pts',(-23.0123815690367,-3.91708714584599,
-1.1574170312224));
#92699=CARTESIAN_POINT('Ctrl Pts',(-22.8145635755996,-1.16464886337962,
-3.91494302862625));
#92700=CARTESIAN_POINT('Ctrl Pts',(-22.6167455821625,2.64749192093593,-3.11030101773335));
#92701=CARTESIAN_POINT('Ctrl Pts',(-22.4189275887254,4.0507059459073,0.524373180214398));
#92702=CARTESIAN_POINT('Ctrl Pts',(-22.2211095952883,1.76822262458715,3.68192539878807));
#92703=CARTESIAN_POINT('Ctrl Pts',(-22.0232916018512,-2.12314900462943,
3.48933004980607));
#92704=CARTESIAN_POINT('Ctrl Pts',(-21.8254736084141,-4.08268831704865,
0.121827739754767));
#92705=CARTESIAN_POINT('Ctrl Pts',(-21.627655614977,-2.32742983944607,-3.3565244278563));
#92706=CARTESIAN_POINT('Ctrl Pts',(-21.4298376215399,1.54553406962469,-3.78080815857784));
#92707=CARTESIAN_POINT('Ctrl Pts',(-21.2320196281028,4.01223178828592,-0.764971874912774));
#92708=CARTESIAN_POINT('Ctrl Pts',(-21.0342016346657,2.82823941680707,2.94690476492853));
#92709=CARTESIAN_POINT('Ctrl Pts',(-20.8363836412285,-0.929140075930861,
3.97742185487519));
#92710=CARTESIAN_POINT('Ctrl Pts',(-20.6385656477914,-3.84110418727031,
1.38892206940278));
#92711=CARTESIAN_POINT('Ctrl Pts',(-20.4407476543543,-3.25808552303732,
-2.46334419375657));
#92712=CARTESIAN_POINT('Ctrl Pts',(-20.2429296609172,0.289432990508367,
-4.07423789638565));
#92713=CARTESIAN_POINT('Ctrl Pts',(-20.0451116674801,3.57359928365308,-1.97802276332043));
#92714=CARTESIAN_POINT('Ctrl Pts',(-19.847293674043,3.60618287186699,1.9179757524517));
#92715=CARTESIAN_POINT('Ctrl Pts',(-19.6494756806059,0.357536269942257,
4.06882706784342));
#92716=CARTESIAN_POINT('Ctrl Pts',(-19.4516576871688,-3.21642905393536,
2.51749280700861));
#92717=CARTESIAN_POINT('Ctrl Pts',(-19.2538396937317,-3.86379733844877,
-1.32448330292826));
#92718=CARTESIAN_POINT('Ctrl Pts',(-19.0560217002946,-0.995534573189098,
-3.96132513256925));
#92719=CARTESIAN_POINT('Ctrl Pts',(-18.8582037068575,2.77855527099065,-2.99379633548938));
#92720=CARTESIAN_POINT('Ctrl Pts',(-18.6603857134204,4.02446510764256,0.697758188563256));
#92721=CARTESIAN_POINT('Ctrl Pts',(-18.4625677199833,1.60855387765517,3.75442942602735));
#92722=CARTESIAN_POINT('Ctrl Pts',(-18.2647497265462,-2.27096464385436,
3.39498239740695));
#92723=CARTESIAN_POINT('Ctrl Pts',(-18.066931733109,-4.0841548578661,-0.0535255948893623));
#92724=CARTESIAN_POINT('Ctrl Pts',(-17.869113739672,-2.18121289084575,-3.45333117687081));
#92725=CARTESIAN_POINT('Ctrl Pts',(-17.6712957462348,1.70639314975703,-3.71098481683796));
#92726=CARTESIAN_POINT('Ctrl Pts',(-17.4734777527977,4.04136891114997,-0.592050011679798));
#92727=CARTESIAN_POINT('Ctrl Pts',(-17.2756597593606,2.69914300198876,3.06558525361058));
#92728=CARTESIAN_POINT('Ctrl Pts',(-17.0778417659235,-1.09900647519767,
3.9338747641242));
#92729=CARTESIAN_POINT('Ctrl Pts',(-16.8800237724864,-3.89718081143694,
1.222770467139));
#92730=CARTESIAN_POINT('Ctrl Pts',(-16.6822057790493,-3.14934880543664,
-2.60092060510013));
#92731=CARTESIAN_POINT('Ctrl Pts',(-16.4843877856122,0.464044584123203,
-4.05805969846249));
#92732=CARTESIAN_POINT('Ctrl Pts',(-16.2865697921751,3.65520838824687,-1.8228103386884));
#92733=CARTESIAN_POINT('Ctrl Pts',(-16.088751798738,3.52053416892211,2.07099615108081));
#92734=CARTESIAN_POINT('Ctrl Pts',(-15.8909338053009,0.182560668631769,
4.08042369057531));
#92735=CARTESIAN_POINT('Ctrl Pts',(-15.6931158118638,-3.32152298156795,
2.37711400131663));
#92736=CARTESIAN_POINT('Ctrl Pts',(-15.4952978184266,-3.80338566527584,
-1.4891082477489));
#92737=CARTESIAN_POINT('Ctrl Pts',(-15.2974798249896,-0.824585284167319,
-4.0004056046199));
#92738=CARTESIAN_POINT('Ctrl Pts',(-15.0996618315524,2.90449710561624,-2.87177339910489));
#92739=CARTESIAN_POINT('Ctrl Pts',(-14.9018438381154,3.99080625600933,0.869857068337309));
#92740=CARTESIAN_POINT('Ctrl Pts',(-14.7040258446782,1.4459201965398,3.82001317767071));
#92741=CARTESIAN_POINT('Ctrl Pts',(-14.5062078512411,-2.41459437373826,
3.29437701282824));
#92742=CARTESIAN_POINT('Ctrl Pts',(-14.308389857804,-4.0780933633985,-0.228780269570442));
#92743=CARTESIAN_POINT('Ctrl Pts',(-14.1105718643669,-2.03097546599567,
-3.54377264350625));
#92744=CARTESIAN_POINT('Ctrl Pts',(-13.9127538709298,1.86410695545964,-3.6343212778931));
#92745=CARTESIAN_POINT('Ctrl Pts',(-13.7149358774927,4.06305686305413,-0.418036864317439));
#92746=CARTESIAN_POINT('Ctrl Pts',(-13.5171178840555,2.5650714467888,3.17861516469175));
#92747=CARTESIAN_POINT('Ctrl Pts',(-13.3192998906185,-1.26684715315575,
3.88307663881113));
#92748=CARTESIAN_POINT('Ctrl Pts',(-13.1214818971813,-3.94607403642267,
1.05436501810828));
#92749=CARTESIAN_POINT('Ctrl Pts',(-12.9236639037443,-3.03480711477366,
-2.7337029224952));
#92750=CARTESIAN_POINT('Ctrl Pts',(-12.7258459103071,0.637800837006619,
-4.03440156462557));
#92751=CARTESIAN_POINT('Ctrl Pts',(-12.52802791687,3.73008010440203,-1.66423805601355));
#92752=CARTESIAN_POINT('Ctrl Pts',(-12.3302099234329,3.42839631305133,2.22019922822156));
#92753=CARTESIAN_POINT('Ctrl Pts',(-12.1323919299958,0.00724856608596741,
4.08449915542031));
#92754=CARTESIAN_POINT('Ctrl Pts',(-11.9345739365587,-3.42049457959367,
2.23235362864174));
#92755=CARTESIAN_POINT('Ctrl Pts',(-11.7367559431216,-3.73596347891545,
-1.65098842411134));
#92756=CARTESIAN_POINT('Ctrl Pts',(-11.5389379496845,-0.65211609510973,
-4.03211241049135));
#92757=CARTESIAN_POINT('Ctrl Pts',(-11.3411199562474,3.02508528508984,-2.74445712487416));
#92758=CARTESIAN_POINT('Ctrl Pts',(-11.1433019628103,3.94979143200078,1.04035260178115));
#92759=CARTESIAN_POINT('Ctrl Pts',(-10.9454839693731,1.28062135246228,3.87855576780291));
#92760=CARTESIAN_POINT('Ctrl Pts',(-10.7476659759361,-2.55377345170589,
3.18769933489685));
#92761=CARTESIAN_POINT('Ctrl Pts',(-10.5498479824989,-4.06451500637211,
-0.40361324967779));
#92762=CARTESIAN_POINT('Ctrl Pts',(-10.3520299890619,-1.87699448697021,
-3.62768212337065));
#92763=CARTESIAN_POINT('Ctrl Pts',(-10.1542119956247,2.01838478397135,-3.55095885025052));
#92764=CARTESIAN_POINT('Ctrl Pts',(-9.95639400218765,4.07725566812261,-0.243253179016498));
#92765=CARTESIAN_POINT('Ctrl Pts',(-9.75857600875052,2.4262718758715,3.2857861580898));
#92766=CARTESIAN_POINT('Ctrl Pts',(-9.56075801531343,-1.43235274089283,
3.82512111154619));
#92767=CARTESIAN_POINT('Ctrl Pts',(-9.3629400218763,-3.98769374078607,0.884016132225644));
#92768=CARTESIAN_POINT('Ctrl Pts',(-9.16512202843922,-2.91467157768749,
-2.86144639763884));
#92769=CARTESIAN_POINT('Ctrl Pts',(-8.96730403500207,0.810381476483423,
-4.00330710224835));
#92770=CARTESIAN_POINT('Ctrl Pts',(-8.769486041565,3.79807642635226,-1.50259820042715));
#92771=CARTESIAN_POINT('Ctrl Pts',(-8.57166804812787,3.32993913548144,2.36530996834002));
#92772=CARTESIAN_POINT('Ctrl Pts',(-8.37385005469078,-0.168076897231722,
4.08104595036081));
#92773=CARTESIAN_POINT('Ctrl Pts',(-8.17603206125366,-3.51316142062967,
2.08347851559342));
#92774=CARTESIAN_POINT('Ctrl Pts',(-7.97821406781657,-3.66165505393974,
-1.80982544967654));
#92775=CARTESIAN_POINT('Ctrl Pts',(-7.78039607437944,-0.478444906337645,
-4.05638710725913));
#92776=CARTESIAN_POINT('Ctrl Pts',(-7.58257808094236,3.14009753770512,-2.6120821859277));
#92777=CARTESIAN_POINT('Ctrl Pts',(-7.38476008750522,3.9014962353557,1.20893052647464));
#92778=CARTESIAN_POINT('Ctrl Pts',(-7.18694209406814,1.11296202915234,3.9299492889857));
#92779=CARTESIAN_POINT('Ctrl Pts',(-6.98912410063102,-2.68824533875734,
3.07514599507246));
#92780=CARTESIAN_POINT('Ctrl Pts',(-6.79130610719391,-4.04344481481362,
-0.577702277884071));
#92781=CARTESIAN_POINT('Ctrl Pts',(-6.5934881137568,-1.71955377608047,-3.70490495201694));
#92782=CARTESIAN_POINT('Ctrl Pts',(-6.3956701203197,2.16894226583871,-3.46105119002063));
#92783=CARTESIAN_POINT('Ctrl Pts',(-6.19785212688258,4.08393915467268,-0.0680211222212914));
#92784=CARTESIAN_POINT('Ctrl Pts',(-6.00003413344548,2.28300012876661,3.38690069300563));
#92785=CARTESIAN_POINT('Ctrl Pts',(-5.80221614000837,-1.59521817369359,
3.76011500776615));
#92786=CARTESIAN_POINT('Ctrl Pts',(-5.60439814657127,-4.02196320968319,
0.712037801432078));
#92787=CARTESIAN_POINT('Ctrl Pts',(-5.40658015313415,-2.78916363188875,
-2.98391556963731));
#92788=CARTESIAN_POINT('Ctrl Pts',(-5.20876215969706,0.981468397431387,
-3.9648336262051));
#92789=CARTESIAN_POINT('Ctrl Pts',(-5.01094416625994,3.85907202005989,-1.33818871007757));
#92790=CARTESIAN_POINT('Ctrl Pts',(-4.81312617282284,3.22534411770083,2.50606089667497));
#92791=CARTESIAN_POINT('Ctrl Pts',(-4.61530817938572,-0.343092560634735,
4.07007044493406));
#92792=CARTESIAN_POINT('Ctrl Pts',(-4.41749018594862,-3.59935268997692,
1.93076306460202));
#92793=CARTESIAN_POINT('Ctrl Pts',(-4.21967219251151,-3.58059737398049,
-1.9653265348854));
#92794=CARTESIAN_POINT('Ctrl Pts',(-4.0218541990744,-0.303891802834324,
-4.07318498256667));
#92795=CARTESIAN_POINT('Ctrl Pts',(-3.8240362056373,3.24932181031572,-2.47489251940337));
#92796=CARTESIAN_POINT('Ctrl Pts',(-3.62621821220018,3.84600979845569,1.37527999920385));
#92797=CARTESIAN_POINT('Ctrl Pts',(-3.42840021876308,0.943251044449692,
3.9740992320543));
#92798=CARTESIAN_POINT('Ctrl Pts',(-3.23058222532597,-2.8177617572936,2.95692403212172));
#92799=CARTESIAN_POINT('Ctrl Pts',(-3.03276423188887,-4.01492242046153,
-0.750725658560183));
#92800=CARTESIAN_POINT('Ctrl Pts',(-2.83494623845176,-1.55894201164752,
-3.77530033988628));
#92801=CARTESIAN_POINT('Ctrl Pts',(-2.63712824501465,2.31549897712062,-3.36476105063503));
#92802=CARTESIAN_POINT('Ctrl Pts',(-2.43931025157754,4.08310057810657,0.107330633052476));
#92803=CARTESIAN_POINT('Ctrl Pts',(-2.24149225814044,2.13550961617047,3.4817832661206));
#92804=CARTESIAN_POINT('Ctrl Pts',(-2.04367426470333,-1.75512282259002,
3.68815733144775));
#92805=CARTESIAN_POINT('Ctrl Pts',(-1.84585627126622,-4.04885838900248,
0.538786873855875));
#92806=CARTESIAN_POINT('Ctrl Pts',(-1.64803827782911,-2.65843974009147,
-3.10096099417392));
#92807=CARTESIAN_POINT('Ctrl Pts',(-1.45022028439201,1.15060289862765,-3.91890598795134));
#92808=CARTESIAN_POINT('Ctrl Pts',(-1.25240229095489,3.91322891566222,-1.17159230533783));
#92809=CARTESIAN_POINT('Ctrl Pts',(-1.05458429751779,3.11427834079904,2.64272844505947));
#92810=CARTESIAN_POINT('Ctrl Pts',(-0.856766304080684,-0.516466827795134,
4.05056289950572));
#92811=CARTESIAN_POINT('Ctrl Pts',(-0.658948310643573,-3.68086436566828,
1.77649746246159));
#92812=CARTESIAN_POINT('Ctrl Pts',(-0.461130317206468,-3.48898854935592,
-2.12138128548535));
#92813=CARTESIAN_POINT('Ctrl Pts',(-0.329251654915064,-1.25514472459608,
-3.42162814095714));
#92814=CARTESIAN_POINT('Ctrl Pts',(-0.263312323769361,-0.109073086534847,
-3.45778011327987));
#92815=CARTESIAN_POINT('Ctrl Pts',(-29.4036876762306,-1.64343044862514,
3.31080057131682));
#92816=CARTESIAN_POINT('Ctrl Pts',(-29.3377483450849,-2.74078612473952,
2.76609010257943));
#92817=CARTESIAN_POINT('Ctrl Pts',(-29.2058696827936,-4.33286715317278,
0.509621633320206));
#92818=CARTESIAN_POINT('Ctrl Pts',(-29.0080516893564,-2.786129234649,-3.36255669633147));
#92819=CARTESIAN_POINT('Ctrl Pts',(-28.8102336959193,1.29928094542948,-4.1648396900737));
#92820=CARTESIAN_POINT('Ctrl Pts',(-28.6124157024822,4.20064038344374,-1.18273102193916));
#92821=CARTESIAN_POINT('Ctrl Pts',(-28.4145977090451,3.28084020858381,2.87819824635538));
#92822=CARTESIAN_POINT('Ctrl Pts',(-28.216779715608,-0.624665972610546,
4.31889413964144));
#92823=CARTESIAN_POINT('Ctrl Pts',(-28.0189617221709,-3.96153263057873,
1.8305962208402));
#92824=CARTESIAN_POINT('Ctrl Pts',(-27.8211437287337,-3.69397677764492,
-2.32372196509937));
#92825=CARTESIAN_POINT('Ctrl Pts',(-27.6233257352967,-0.0652364080480912,
-4.36351059266543));
#92826=CARTESIAN_POINT('Ctrl Pts',(-27.4255077418595,3.62282456707754,-2.43308738034599));
#92827=CARTESIAN_POINT('Ctrl Pts',(-27.2276897484225,4.01453275210466,1.71123201057149));
#92828=CARTESIAN_POINT('Ctrl Pts',(-27.0298717549853,0.75344702936726,4.29849008658198));
#92829=CARTESIAN_POINT('Ctrl Pts',(-26.8320537615483,-3.19318738180644,
2.97460920569266));
#92830=CARTESIAN_POINT('Ctrl Pts',(-26.6342357681111,-4.23437490293385,
-1.05584691784211));
#92831=CARTESIAN_POINT('Ctrl Pts',(-26.436417774674,-1.42274505435184,-4.12559433567772));
#92832=CARTESIAN_POINT('Ctrl Pts',(-26.2385997812369,2.68342571307752,-3.44150630056508));
#92833=CARTESIAN_POINT('Ctrl Pts',(-26.0407817877998,4.34797431489627,0.373975435205314));
#92834=CARTESIAN_POINT('Ctrl Pts',(-25.8429637943627,2.05634380943297,3.84918004191613));
#92835=CARTESIAN_POINT('Ctrl Pts',(-25.6451458009256,-2.10633351714236,
3.822054031928));
#92836=CARTESIAN_POINT('Ctrl Pts',(-25.4473278074885,-4.35247882946084,
0.31727863829441));
#92837=CARTESIAN_POINT('Ctrl Pts',(-25.2495098140514,-2.63834659872647,
-3.47618537407148));
#92838=CARTESIAN_POINT('Ctrl Pts',(-25.0516918206143,1.47639113755023,-4.10670267869265));
#92839=CARTESIAN_POINT('Ctrl Pts',(-24.8538738271771,4.24777516269504,-1.00057174045179));
#92840=CARTESIAN_POINT('Ctrl Pts',(-24.6560558337401,3.15415050271192,3.01596953382905));
#92841=CARTESIAN_POINT('Ctrl Pts',(-24.4582378403029,-0.809404555575561,
4.28830991297042));
#92842=CARTESIAN_POINT('Ctrl Pts',(-24.2604198468659,-4.03649040139732,
1.65875943895133));
#92843=CARTESIAN_POINT('Ctrl Pts',(-24.0626018534287,-3.59081348392226,
-2.48007986945916));
#92844=CARTESIAN_POINT('Ctrl Pts',(-23.8647838599917,0.122109169034145,
-4.36231899212071));
#92845=CARTESIAN_POINT('Ctrl Pts',(-23.6669658665545,3.72392589487205,-2.27532713394089));
#92846=CARTESIAN_POINT('Ctrl Pts',(-23.4691478731174,3.93737921636729,1.88196241815778));
#92847=CARTESIAN_POINT('Ctrl Pts',(-23.2713298796803,0.568250063912948,
4.32687294730266));
#92848=CARTESIAN_POINT('Ctrl Pts',(-23.0735118862432,-3.31792421120822,
2.83480450220432));
#92849=CARTESIAN_POINT('Ctrl Pts',(-22.8756938928061,-4.18515200544392,
-1.23662457050318));
#92850=CARTESIAN_POINT('Ctrl Pts',(-22.6778758993689,-1.24435131124929,
-4.1828611561092));
#92851=CARTESIAN_POINT('Ctrl Pts',(-22.4800579059319,2.82867235518411,-3.32315367446072));
#92852=CARTESIAN_POINT('Ctrl Pts',(-22.2822399124947,4.32791497400198,0.560258525037564));
#92853=CARTESIAN_POINT('Ctrl Pts',(-22.0844219190577,1.88923048883661,3.9338970242146));
#92854=CARTESIAN_POINT('Ctrl Pts',(-21.8866039256205,-2.26844616515726,
3.72812146165506));
#92855=CARTESIAN_POINT('Ctrl Pts',(-21.6887859321835,-4.36208605055386,
0.13016499004728));
#92856=CARTESIAN_POINT('Ctrl Pts',(-21.4909679387463,-2.48670690679362,
-3.58622732084516));
#92857=CARTESIAN_POINT('Ctrl Pts',(-21.2931499453092,1.65130229942196,-4.03954680044611));
#92858=CARTESIAN_POINT('Ctrl Pts',(-21.0953319518721,4.28680784721833,-0.817322530032182));
#92859=CARTESIAN_POINT('Ctrl Pts',(-20.897513958435,3.02178925982747,3.14857544077672));
#92860=CARTESIAN_POINT('Ctrl Pts',(-20.6996959649979,-0.992725540008512,
4.24961570489448));
#92861=CARTESIAN_POINT('Ctrl Pts',(-20.5018779715608,-4.10396917248096,
1.48397259691575));
#92862=CARTESIAN_POINT('Ctrl Pts',(-20.3040599781237,-3.48105177468615,
-2.63192252527032));
#92863=CARTESIAN_POINT('Ctrl Pts',(-20.1062419846866,0.309240263380999,
-4.35305732750844));
#92864=CARTESIAN_POINT('Ctrl Pts',(-19.9084239912495,3.81815763902375,-2.1133882465452));
#92865=CARTESIAN_POINT('Ctrl Pts',(-19.7106059978124,3.8529710767852,2.04923193380534));
#92866=CARTESIAN_POINT('Ctrl Pts',(-19.5127880043752,0.382004173370155,
4.34727621029521));
#92867=CARTESIAN_POINT('Ctrl Pts',(-19.3149700109382,-3.43654455574752,
2.68977678505725));
#92868=CARTESIAN_POINT('Ctrl Pts',(-19.117152017501,-4.12821532367142,-1.41512397989553));
#92869=CARTESIAN_POINT('Ctrl Pts',(-18.9193340240639,-1.06366372774973,
-4.23241740750371));
#92870=CARTESIAN_POINT('Ctrl Pts',(-18.7215160306268,2.96870499216626,-3.19867602400712));
#92871=CARTESIAN_POINT('Ctrl Pts',(-18.5236980371897,4.2998783506645,0.745509092203192));
#92872=CARTESIAN_POINT('Ctrl Pts',(-18.3258800437526,1.71863485193899,4.01136284606261));
#92873=CARTESIAN_POINT('Ctrl Pts',(-18.1280620503155,-2.42637752994556,
3.62731715173159));
#92874=CARTESIAN_POINT('Ctrl Pts',(-17.9302440568784,-4.36365295371805,
-0.0571886053215215));
#92875=CARTESIAN_POINT('Ctrl Pts',(-17.7324260634413,-2.330483638615,-3.6896590150336));
#92876=CARTESIAN_POINT('Ctrl Pts',(-17.5346080700042,1.82316972966886,-3.96494511612583));
#92877=CARTESIAN_POINT('Ctrl Pts',(-17.3367900765671,4.31793896165287,-0.63256680320031));
#92878=CARTESIAN_POINT('Ctrl Pts',(-17.13897208313,2.88385816479288,3.27537779842697));
#92879=CARTESIAN_POINT('Ctrl Pts',(-16.9411540896929,-1.17421670297713,
4.20308848009656));
#92880=CARTESIAN_POINT('Ctrl Pts',(-16.7433360962557,-4.16388338611759,
1.30645045213544));
#92881=CARTESIAN_POINT('Ctrl Pts',(-16.5455181028187,-3.36487368755462,
-2.77891394322918));
#92882=CARTESIAN_POINT('Ctrl Pts',(-16.3477001093815,0.495801356862377,
-4.33577197873739));
#92883=CARTESIAN_POINT('Ctrl Pts',(-16.1498821159444,3.90535164187237,-1.94755389922735));
#92884=CARTESIAN_POINT('Ctrl Pts',(-15.9520641225073,3.7614610267028,2.21272424437995));
#92885=CARTESIAN_POINT('Ctrl Pts',(-15.7542461290702,0.19505416141933,4.35966644494551));
#92886=CARTESIAN_POINT('Ctrl Pts',(-15.5564281356331,-3.54883055950875,
2.53979119160763));
#92887=CARTESIAN_POINT('Ctrl Pts',(-15.358610142196,-4.0636693930556,-1.59101499082003));
#92888=CARTESIAN_POINT('Ctrl Pts',(-15.1607921487589,-0.881015567742002,
-4.27417234168993));
#92889=CARTESIAN_POINT('Ctrl Pts',(-14.9629741553218,3.10326562411736,-3.06830247909855));
#92890=CARTESIAN_POINT('Ctrl Pts',(-14.7651561618847,4.26391606410594,0.929385514913071));
#92891=CARTESIAN_POINT('Ctrl Pts',(-14.5673381684476,1.54487137634347,4.08143480501962));
#92892=CARTESIAN_POINT('Ctrl Pts',(-14.3695201750105,-2.57983652375489,
3.51982686332313));
#92893=CARTESIAN_POINT('Ctrl Pts',(-14.1717021815733,-4.3571766424228,-0.244436788957864));
#92894=CARTESIAN_POINT('Ctrl Pts',(-13.9738841881363,-2.16996475392007,
-3.7862898203671));
#92895=CARTESIAN_POINT('Ctrl Pts',(-13.7760661946991,1.99167663943278,-3.88303512744974));
#92896=CARTESIAN_POINT('Ctrl Pts',(-13.578248201262,4.3411111230131,-0.446645110488031));
#92897=CARTESIAN_POINT('Ctrl Pts',(-13.3804302078249,2.74061145691375,3.39614288263965));
#92898=CARTESIAN_POINT('Ctrl Pts',(-13.1826122143878,-1.35354351491601,
4.14881399803603));
#92899=CARTESIAN_POINT('Ctrl Pts',(-12.9847942209507,-4.21612260648281,
1.12652021915962));
#92900=CARTESIAN_POINT('Ctrl Pts',(-12.7869762275136,-3.24249336551008,
-2.92078318464312));
#92901=CARTESIAN_POINT('Ctrl Pts',(-12.5891582340765,0.681448574587572,
-4.3104948065464));
#92902=CARTESIAN_POINT('Ctrl Pts',(-12.3913402406394,3.98534718482324,-1.77812976283858));
#92903=CARTESIAN_POINT('Ctrl Pts',(-12.1935222472022,3.66301774016938,2.37213799604391));
#92904=CARTESIAN_POINT('Ctrl Pts',(-11.9957042537652,0.0077446198569954,
4.36402081318755));
#92905=CARTESIAN_POINT('Ctrl Pts',(-11.797886260328,-3.65457525359824,2.38512417975633));
#92906=CARTESIAN_POINT('Ctrl Pts',(-11.600068266891,-3.99163318657067,-1.76397339575705));
#92907=CARTESIAN_POINT('Ctrl Pts',(-11.4022502734539,-0.696743493727229,
-4.30804899473296));
#92908=CARTESIAN_POINT('Ctrl Pts',(-11.2044322800167,3.23210622489183,-2.93227334811854));
#92909=CARTESIAN_POINT('Ctrl Pts',(-11.0066142865797,4.22009440107903,1.11154886669564));
#92910=CARTESIAN_POINT('Ctrl Pts',(-10.8087962931425,1.36826034803836,4.14398374237361));
#92911=CARTESIAN_POINT('Ctrl Pts',(-10.6109782997055,-2.72854028641939,
3.40584872571541));
#92912=CARTESIAN_POINT('Ctrl Pts',(-10.4131603062683,-4.34266905399709,
-0.431234419459898));
#92913=CARTESIAN_POINT('Ctrl Pts',(-10.2153423128312,-2.00544612587474,
-3.87594162408116));
#92914=CARTESIAN_POINT('Ctrl Pts',(-10.0175243193941,2.15651243178323,-3.79396781333675));
#92915=CARTESIAN_POINT('Ctrl Pts',(-9.81970632595701,4.35628161968441,-0.259900148269901));
#92916=CARTESIAN_POINT('Ctrl Pts',(-9.62188833251987,2.59231317276776,3.51064809563215));
#92917=CARTESIAN_POINT('Ctrl Pts',(-9.42407033908278,-1.53037543533029,
4.08689229904686));
#92918=CARTESIAN_POINT('Ctrl Pts',(-9.22625234564566,-4.26059054469735,
0.944513550726706));
#92919=CARTESIAN_POINT('Ctrl Pts',(-9.02843435220857,-3.11413638358937,
-3.05726875192153));
#92920=CARTESIAN_POINT('Ctrl Pts',(-8.83061635877144,0.865839726102576,
-4.27727240256842));
#92921=CARTESIAN_POINT('Ctrl Pts',(-8.63279836533435,4.05799681772063,-1.6054281249686));
#92922=CARTESIAN_POINT('Ctrl Pts',(-8.43498037189723,3.5578226707684,2.52717935264541));
#92923=CARTESIAN_POINT('Ctrl Pts',(-8.23716237846013,-0.179579196818253,
4.36033128892069));
#92924=CARTESIAN_POINT('Ctrl Pts',(-8.03934438502301,-3.75358372626171,
2.2260608363238));
#92925=CARTESIAN_POINT('Ctrl Pts',(-7.84152639158592,-3.91223948348743,
-1.93368039264833));
#92926=CARTESIAN_POINT('Ctrl Pts',(-7.64370839814879,-0.511187161454119,
-4.33398492418169));
#92927=CARTESIAN_POINT('Ctrl Pts',(-7.44589040471171,3.35498931167584,-2.79083936399343));
#92928=CARTESIAN_POINT('Ctrl Pts',(-7.24807241127459,4.16849413497138,1.2916633786622));
#92929=CARTESIAN_POINT('Ctrl Pts',(-7.05025441783749,1.1891273017067,4.19889436606833));
#92930=CARTESIAN_POINT('Ctrl Pts',(-6.85243642440037,-2.87221472275815,
3.2855928267919));
#92931=CARTESIAN_POINT('Ctrl Pts',(-6.65461843096327,-4.32015692925418,
-0.617237185902298));
#92932=CARTESIAN_POINT('Ctrl Pts',(-6.45680043752616,-1.83723100009755,
-3.95844917730672));
#92933=CARTESIAN_POINT('Ctrl Pts',(-6.25898244408905,2.31737327651579,-3.697907345314));
#92934=CARTESIAN_POINT('Ctrl Pts',(-6.06116445065195,4.3634224889316,-0.0726761303686811));
#92935=CARTESIAN_POINT('Ctrl Pts',(-5.86334645721483,2.4392366601976,3.61868237795117));
#92936=CARTESIAN_POINT('Ctrl Pts',(-5.66552846377773,-1.70438652247867,
4.01743751913734));
#92937=CARTESIAN_POINT('Ctrl Pts',(-5.46771047034062,-4.29720523595649,
0.76076592673604));
#92938=CARTESIAN_POINT('Ctrl Pts',(-5.26989247690351,-2.9800393335363,-3.18811907046449));
#92939=CARTESIAN_POINT('Ctrl Pts',(-5.07207448346641,1.04863493684225,-4.23616600400653));
#92940=CARTESIAN_POINT('Ctrl Pts',(-4.8742564900293,4.123166629324,-1.42976731308693));
#92941=CARTESIAN_POINT('Ctrl Pts',(-4.67643849659219,3.44606971962761,2.67756253485615));
#92942=CARTESIAN_POINT('Ctrl Pts',(-4.47862050315508,-0.366572012500694,
4.34860467757986));
#92943=CARTESIAN_POINT('Ctrl Pts',(-4.28080250971799,-3.84567347313981,
2.0628943424007));
#92944=CARTESIAN_POINT('Ctrl Pts',(-4.08298451628086,-3.82563464187755,
-2.09982315495596));
#92945=CARTESIAN_POINT('Ctrl Pts',(-3.88516652284376,-0.324688560840112,
-4.35193235780086));
#92946=CARTESIAN_POINT('Ctrl Pts',(-3.68734852940666,3.47168831952001,-2.64426115763686));
#92947=CARTESIAN_POINT('Ctrl Pts',(-3.48953053596954,4.10921049791642,1.46939693512277));
#92948=CARTESIAN_POINT('Ctrl Pts',(-3.29171254253244,1.0078021890583,4.24606569922841));
#92949=CARTESIAN_POINT('Ctrl Pts',(-3.09389454909533,-3.01059456435799,
3.15928037396442));
#92950=CARTESIAN_POINT('Ctrl Pts',(-2.89607655565822,-4.28968261212052,
-0.80210137749764));
#92951=CARTESIAN_POINT('Ctrl Pts',(-2.69825856222111,-1.66562781053683,
-4.0336620555874));
#92952=CARTESIAN_POINT('Ctrl Pts',(-2.50044056878401,2.47395955894843,-3.59502761480265));
#92953=CARTESIAN_POINT('Ctrl Pts',(-2.30262257534689,4.36252652459211,0.114675777545951));
#92954=CARTESIAN_POINT('Ctrl Pts',(-2.10480458190979,2.28165267199598,3.72005821575322));
#92955=CARTESIAN_POINT('Ctrl Pts',(-1.90698658847269,-1.87523420523149,
3.94055543759611));
#92956=CARTESIAN_POINT('Ctrl Pts',(-1.70916859503558,-4.32594098001169,
0.575658616126547));
#92957=CARTESIAN_POINT('Ctrl Pts',(-1.51135060159847,-2.84036938555083,
-3.3131744687716));
#92958=CARTESIAN_POINT('Ctrl Pts',(-1.31353260816137,1.22934411448257,-4.18709531954478));
#92959=CARTESIAN_POINT('Ctrl Pts',(-1.11571461472425,4.18102973826174,-1.25176992588667));
#92960=CARTESIAN_POINT('Ctrl Pts',(-0.917896621287149,3.32740318461583,
2.82358289205118));
#92961=CARTESIAN_POINT('Ctrl Pts',(-0.720078627850039,-0.55181110340736,
4.32776213825641));
#92962=CARTESIAN_POINT('Ctrl Pts',(-0.52226063441293,-3.93276337956392,
1.89807161313012));
#92963=CARTESIAN_POINT('Ctrl Pts',(-0.324442640975823,-3.72775659070872,
-2.26655747260449));
#92964=CARTESIAN_POINT('Ctrl Pts',(-0.192563978684421,-1.34104023364309,
-3.65578638994445));
#92965=CARTESIAN_POINT('Ctrl Pts',(-0.126624647538717,-0.116537475387898,
-3.69441241327091));
#92966=CARTESIAN_POINT('Ctrl Pts',(-29.267,-1.74869447533113,3.52286199445087));
#92967=CARTESIAN_POINT('Ctrl Pts',(-29.2010606688543,-2.91633732258384,
2.94326205571725));
#92968=CARTESIAN_POINT('Ctrl Pts',(-29.0691820065629,-4.61039337529348,
0.542263614162568));
#92969=CARTESIAN_POINT('Ctrl Pts',(-28.8713640131258,-2.96458472231979,
-3.57793317190983));
#92970=CARTESIAN_POINT('Ctrl Pts',(-28.6735460196887,1.38250171345935,-4.43160351736486));
#92971=CARTESIAN_POINT('Ctrl Pts',(-28.4757280262516,4.46969729538972,-1.25848660379756));
#92972=CARTESIAN_POINT('Ctrl Pts',(-28.2779100328145,3.49098262843696,3.06255088344016));
#92973=CARTESIAN_POINT('Ctrl Pts',(-28.0800920393773,-0.66467670484336,
4.59552537063505));
#92974=CARTESIAN_POINT('Ctrl Pts',(-27.8822740459403,-4.21527435537805,
1.94784847793426));
#92975=CARTESIAN_POINT('Ctrl Pts',(-27.6844560525031,-3.93058117456272,
-2.47255961819028));
#92976=CARTESIAN_POINT('Ctrl Pts',(-27.486638059066,-0.069414891539576,
-4.64299957009216));
#92977=CARTESIAN_POINT('Ctrl Pts',(-27.2888200656289,3.85487156504997,-2.58893004177228));
#92978=CARTESIAN_POINT('Ctrl Pts',(-27.0910020721918,4.27166920907071,1.8208388224762));
#92979=CARTESIAN_POINT('Ctrl Pts',(-26.8931840787547,0.801706369023046,
4.57381440934107));
#92980=CARTESIAN_POINT('Ctrl Pts',(-26.6953660853176,-3.39771551508819,
3.16513710003091));
#92981=CARTESIAN_POINT('Ctrl Pts',(-26.4975480918805,-4.50559255819786,
-1.12347539475766));
#92982=CARTESIAN_POINT('Ctrl Pts',(-26.2997300984434,-1.51387387183383,
-4.38984444294094));
#92983=CARTESIAN_POINT('Ctrl Pts',(-26.1019121050063,2.85530289605246,-3.66193960909637));
#92984=CARTESIAN_POINT('Ctrl Pts',(-25.9040941115692,4.62646817192751,0.39792908668583));
#92985=CARTESIAN_POINT('Ctrl Pts',(-25.7062761181321,2.18805551640172,4.09572542573043));
#92986=CARTESIAN_POINT('Ctrl Pts',(-25.5084581246949,-2.24124713504792,
4.06686195673259));
#92987=CARTESIAN_POINT('Ctrl Pts',(-25.3106401312579,-4.63126120697179,
0.337600780361695));
#92988=CARTESIAN_POINT('Ctrl Pts',(-25.1128221378207,-2.80733640116096,
-3.69883992593119));
#92989=CARTESIAN_POINT('Ctrl Pts',(-24.9150041443836,1.57095606195064,-4.3697427488125));
#92990=CARTESIAN_POINT('Ctrl Pts',(-24.7171861509466,4.51985112340335,-1.06465976467958));
#92991=CARTESIAN_POINT('Ctrl Pts',(-24.5193681575094,3.35617826910138,3.20914661523155));
#92992=CARTESIAN_POINT('Ctrl Pts',(-24.3215501640723,-0.861248053318545,
4.56298218132233));
#92993=CARTESIAN_POINT('Ctrl Pts',(-24.1237321706352,-4.29503327661702,
1.76500530900118));
#92994=CARTESIAN_POINT('Ctrl Pts',(-23.9259141771981,-3.82081012709267,
-2.63893246576473));
#92995=CARTESIAN_POINT('Ctrl Pts',(-23.7280961837609,0.129930432684828,
-4.6417316458602));
#92996=CARTESIAN_POINT('Ctrl Pts',(-23.5302781903239,3.96244857478032,-2.4210650301764));
#92997=CARTESIAN_POINT('Ctrl Pts',(-23.3324601968868,4.18957388108829,2.00250475227989));
#92998=CARTESIAN_POINT('Ctrl Pts',(-23.1346422034497,0.604647278016807,
4.60401523212482));
#92999=CARTESIAN_POINT('Ctrl Pts',(-22.9368242100126,-3.53044191347499,
3.01637770907531));
#93000=CARTESIAN_POINT('Ctrl Pts',(-22.7390062165754,-4.45321686504185,
-1.31583210978398));
#93001=CARTESIAN_POINT('Ctrl Pts',(-22.5411882231384,-1.32405375911896,
-4.45077928359215));
#93002=CARTESIAN_POINT('Ctrl Pts',(-22.3433702297012,3.00985278943228,-3.53600633118811));
#93003=CARTESIAN_POINT('Ctrl Pts',(-22.1455522362642,4.60512400209667,0.596143869860738));
#93004=CARTESIAN_POINT('Ctrl Pts',(-21.947734242827,2.01023835308607,4.18586864964113));
#93005=CARTESIAN_POINT('Ctrl Pts',(-21.7499162493899,-2.41374332568508,
3.96691287350406));
#93006=CARTESIAN_POINT('Ctrl Pts',(-21.5520982559528,-4.64148378405907,
0.138502240339789));
#93007=CARTESIAN_POINT('Ctrl Pts',(-21.3542802625157,-2.64598397414117,
-3.81593021383402));
#93008=CARTESIAN_POINT('Ctrl Pts',(-21.1564622690786,1.75707052921922,-4.29828544231439));
#93009=CARTESIAN_POINT('Ctrl Pts',(-20.9586442756415,4.56138390615074,-0.869673185151591));
#93010=CARTESIAN_POINT('Ctrl Pts',(-20.7608262822044,3.21533910284787,3.35024611662491));
#93011=CARTESIAN_POINT('Ctrl Pts',(-20.5630082887673,-1.05631100408616,
4.52180955491376));
#93012=CARTESIAN_POINT('Ctrl Pts',(-20.3651902953302,-4.36683415769162,
1.57902312442871));
#93013=CARTESIAN_POINT('Ctrl Pts',(-20.167372301893,-3.70401802633496,-2.80050085678409));
#93014=CARTESIAN_POINT('Ctrl Pts',(-19.9695543084559,0.329047536253623,
-4.63187675863124));
#93015=CARTESIAN_POINT('Ctrl Pts',(-19.7717363150188,4.06271599439444,-2.24875372976998));
#93016=CARTESIAN_POINT('Ctrl Pts',(-19.5739183215817,4.0997592817034,2.18048811515899));
#93017=CARTESIAN_POINT('Ctrl Pts',(-19.3761003281446,0.406472076798061,
4.62572535274699));
#93018=CARTESIAN_POINT('Ctrl Pts',(-19.1782823347075,-3.65666005755969,
2.8620607631059));
#93019=CARTESIAN_POINT('Ctrl Pts',(-18.9804643412704,-4.39263330889407,
-1.5057646568628));
#93020=CARTESIAN_POINT('Ctrl Pts',(-18.7826463478333,-1.13179288231037,
-4.50350968243817));
#93021=CARTESIAN_POINT('Ctrl Pts',(-18.5848283543962,3.15885471334188,-3.40355571252486));
#93022=CARTESIAN_POINT('Ctrl Pts',(-18.3870103609591,4.57529159368643,0.793259995843121));
#93023=CARTESIAN_POINT('Ctrl Pts',(-18.189192367522,1.82871582622281,4.26829626609787));
#93024=CARTESIAN_POINT('Ctrl Pts',(-17.9913743740849,-2.58179041603676,
3.85965190605623));
#93025=CARTESIAN_POINT('Ctrl Pts',(-17.7935563806477,-4.64315104957,-0.0608516157536774));
#93026=CARTESIAN_POINT('Ctrl Pts',(-17.5957383872107,-2.47975438638425,
-3.92598685319639));
#93027=CARTESIAN_POINT('Ctrl Pts',(-17.3979203937735,1.93994630958068,-4.2189054154137));
#93028=CARTESIAN_POINT('Ctrl Pts',(-17.2001024003365,4.59450901215576,-0.673083594720819));
#93029=CARTESIAN_POINT('Ctrl Pts',(-17.0022844068993,3.06857332759699,3.48517034324336));
#93030=CARTESIAN_POINT('Ctrl Pts',(-16.8044664134622,-1.24942693075659,
4.47230219606893));
#93031=CARTESIAN_POINT('Ctrl Pts',(-16.6066484200251,-4.43058596079823,
1.39013043713188));
#93032=CARTESIAN_POINT('Ctrl Pts',(-16.408830426588,-3.58039856967259,-2.95690728135824));
#93033=CARTESIAN_POINT('Ctrl Pts',(-16.2110124331509,0.527558129601547,
-4.61348425901228));
#93034=CARTESIAN_POINT('Ctrl Pts',(-16.0131944397138,4.15549489549788,-2.07229745976629));
#93035=CARTESIAN_POINT('Ctrl Pts',(-15.8153764462767,4.00238788448349,2.35445233767909));
#93036=CARTESIAN_POINT('Ctrl Pts',(-15.6175584528395,0.207547654206896,
4.63890919931572));
#93037=CARTESIAN_POINT('Ctrl Pts',(-15.4197404594025,-3.77613813744956,
2.70246838189863));
#93038=CARTESIAN_POINT('Ctrl Pts',(-15.2219224659653,-4.32395312083535,
-1.69292173389115));
#93039=CARTESIAN_POINT('Ctrl Pts',(-15.0241044725283,-0.937445851316686,
-4.54793907875995));
#93040=CARTESIAN_POINT('Ctrl Pts',(-14.8262864790911,3.30203414261849,-3.26483155909222));
#93041=CARTESIAN_POINT('Ctrl Pts',(-14.6284684856541,4.53702587220254,0.988913961488839));
#93042=CARTESIAN_POINT('Ctrl Pts',(-14.4306504922169,1.64382255614715,4.34285643236852));
#93043=CARTESIAN_POINT('Ctrl Pts',(-14.2328324987798,-2.74507867377152,
3.74527671381803));
#93044=CARTESIAN_POINT('Ctrl Pts',(-14.0350145053427,-4.63625992144711,
-0.260093308345293));
#93045=CARTESIAN_POINT('Ctrl Pts',(-13.8371965119056,-2.30895404184448,
-4.02880699722795));
#93046=CARTESIAN_POINT('Ctrl Pts',(-13.6393785184685,2.11924632340592,-4.13174897700638));
#93047=CARTESIAN_POINT('Ctrl Pts',(-13.4415605250314,4.61916538297207,-0.475253356658625));
#93048=CARTESIAN_POINT('Ctrl Pts',(-13.2437425315943,2.9161514670387,3.61367060058756));
#93049=CARTESIAN_POINT('Ctrl Pts',(-13.0459245381572,-1.44023987667628,
4.41455135726092));
#93050=CARTESIAN_POINT('Ctrl Pts',(-12.8481065447201,-4.48617117654295,
1.19867542021098));
#93051=CARTESIAN_POINT('Ctrl Pts',(-12.650288551283,-3.45017961624651,-3.10786344679104));
#93052=CARTESIAN_POINT('Ctrl Pts',(-12.4524705578459,0.72509631216853,-4.58658804846722));
#93053=CARTESIAN_POINT('Ctrl Pts',(-12.2546525644087,4.24061426524445,-1.89202146966362));
#93054=CARTESIAN_POINT('Ctrl Pts',(-12.0568345709716,3.89763916728744,2.52407676386627));
#93055=CARTESIAN_POINT('Ctrl Pts',(-11.8590165775345,0.00824067362801503,
4.64354247095479));
#93056=CARTESIAN_POINT('Ctrl Pts',(-11.6611985840974,-3.88865592760281,
2.53789473087093));
#93057=CARTESIAN_POINT('Ctrl Pts',(-11.4633805906603,-4.24730289422589,
-1.87695836740277));
#93058=CARTESIAN_POINT('Ctrl Pts',(-11.2655625972232,-0.741370892344723,
-4.58398557897456));
#93059=CARTESIAN_POINT('Ctrl Pts',(-11.0677446037861,3.43912716469383,-3.12008957136294));
#93060=CARTESIAN_POINT('Ctrl Pts',(-10.869926610349,4.49039737015727,1.18274513161014));
#93061=CARTESIAN_POINT('Ctrl Pts',(-10.6721086169119,1.45589934361444,4.40941171694431));
#93062=CARTESIAN_POINT('Ctrl Pts',(-10.4742906234748,-2.90330712113289,
3.62399811653398));
#93063=CARTESIAN_POINT('Ctrl Pts',(-10.2764726300377,-4.62082310162206,
-0.458855589242014));
#93064=CARTESIAN_POINT('Ctrl Pts',(-10.0786546366006,-2.13389776477927,
-4.12420112479167));
#93065=CARTESIAN_POINT('Ctrl Pts',(-9.88083664316343,2.29464007959512,-4.03697677642298));
#93066=CARTESIAN_POINT('Ctrl Pts',(-9.68301864972636,4.6353075712462,-0.276547117523308));
#93067=CARTESIAN_POINT('Ctrl Pts',(-9.48520065628923,2.758354469664,3.7355100331745));
#93068=CARTESIAN_POINT('Ctrl Pts',(-9.28738266285214,-1.62839812976774,
4.34866348654753));
#93069=CARTESIAN_POINT('Ctrl Pts',(-9.08956466941501,-4.53348734860864,
1.00501096922777));
#93070=CARTESIAN_POINT('Ctrl Pts',(-8.89174667597792,-3.31360118949124,
-3.25309110620423));
#93071=CARTESIAN_POINT('Ctrl Pts',(-8.69392868254081,0.921297975721724,
-4.5512377028885));
#93072=CARTESIAN_POINT('Ctrl Pts',(-8.49611068910371,4.31791720908901,-1.70825804951004));
#93073=CARTESIAN_POINT('Ctrl Pts',(-8.29829269566658,3.78570620605536,2.68904873695079));
#93074=CARTESIAN_POINT('Ctrl Pts',(-8.1004747022295,-0.191081496404787,
4.63961662748058));
#93075=CARTESIAN_POINT('Ctrl Pts',(-7.90265670879236,-3.99400603189376,
2.36864315705417));
#93076=CARTESIAN_POINT('Ctrl Pts',(-7.70483871535528,-4.16282391303512,
-2.05753533562012));
#93077=CARTESIAN_POINT('Ctrl Pts',(-7.50702072191814,-0.543929416570591,
-4.61158274110426));
#93078=CARTESIAN_POINT('Ctrl Pts',(-7.30920272848107,3.56988108564655,-2.96959654205915));
#93079=CARTESIAN_POINT('Ctrl Pts',(-7.11138473504394,4.43549203458706,1.37439623084976));
#93080=CARTESIAN_POINT('Ctrl Pts',(-6.91356674160684,1.26529257426107,4.46783944315096));
#93081=CARTESIAN_POINT('Ctrl Pts',(-6.71574874816973,-3.05618410675896,
3.49603965851134));
#93082=CARTESIAN_POINT('Ctrl Pts',(-6.51793075473263,-4.59686904369474,
-0.656772093920519));
#93083=CARTESIAN_POINT('Ctrl Pts',(-6.32011276129551,-1.95490822411462,
-4.21199340259651));
#93084=CARTESIAN_POINT('Ctrl Pts',(-6.12229476785841,2.46580428719285,-3.93476350060735));
#93085=CARTESIAN_POINT('Ctrl Pts',(-5.9244767744213,4.64290582319052,-0.0773311385160742));
#93086=CARTESIAN_POINT('Ctrl Pts',(-5.72665878098419,2.59547319162859,3.85046406289671));
#93087=CARTESIAN_POINT('Ctrl Pts',(-5.52884078754709,-1.81355487126374,
4.27476003050852));
#93088=CARTESIAN_POINT('Ctrl Pts',(-5.33102279410998,-4.57244726222979,
0.809494052040002));
#93089=CARTESIAN_POINT('Ctrl Pts',(-5.13320480067286,-3.17091503518384,
-3.39232257129167));
#93090=CARTESIAN_POINT('Ctrl Pts',(-4.93538680723577,1.11580147625311,-4.50749838180796));
#93091=CARTESIAN_POINT('Ctrl Pts',(-4.73756881379865,4.3872612385881,-1.52134591609628));
#93092=CARTESIAN_POINT('Ctrl Pts',(-4.53975082036155,3.66679532155438,2.84906417303733));
#93093=CARTESIAN_POINT('Ctrl Pts',(-4.34193282692444,-0.390051464366645,
4.62713891022566));
#93094=CARTESIAN_POINT('Ctrl Pts',(-4.14411483348734,-4.09199425630271,
2.19502562019938));
#93095=CARTESIAN_POINT('Ctrl Pts',(-3.94629684005023,-4.07067190977461,
-2.23431977502652));
#93096=CARTESIAN_POINT('Ctrl Pts',(-3.74847884661311,-0.345485318845901,
-4.63067973303504));
#93097=CARTESIAN_POINT('Ctrl Pts',(-3.55066085317602,3.6940548287243,-2.81362979587035));
#93098=CARTESIAN_POINT('Ctrl Pts',(-3.35284285973889,4.37241119737715,1.5635138710417));
#93099=CARTESIAN_POINT('Ctrl Pts',(-3.1550248663018,1.0723533336669,4.51803216640253));
#93100=CARTESIAN_POINT('Ctrl Pts',(-2.95720687286468,-3.20342737142238,
3.36163671580712));
#93101=CARTESIAN_POINT('Ctrl Pts',(-2.75938887942758,-4.5644428037795,-0.853477096435094));
#93102=CARTESIAN_POINT('Ctrl Pts',(-2.56157088599047,-1.77231360942614,
-4.29202377128854));
#93103=CARTESIAN_POINT('Ctrl Pts',(-2.36375289255336,2.63242014077624,-3.82529417897026));
#93104=CARTESIAN_POINT('Ctrl Pts',(-2.16593489911625,4.64195247107765,0.122020922039425));
#93105=CARTESIAN_POINT('Ctrl Pts',(-1.96811690567915,2.42779572782149,3.95833316538584));
#93106=CARTESIAN_POINT('Ctrl Pts',(-1.77029891224204,-1.99534558787297,
4.19295354374447));
#93107=CARTESIAN_POINT('Ctrl Pts',(-1.57248091880493,-4.60302357102089,
0.612530358397211));
#93108=CARTESIAN_POINT('Ctrl Pts',(-1.37466292536783,-3.02229903101019,
-3.52538794336927));
#93109=CARTESIAN_POINT('Ctrl Pts',(-1.17684493193072,1.30808533033749,-4.45528465113822));
#93110=CARTESIAN_POINT('Ctrl Pts',(-0.979026938493605,4.44883056086126,
-1.33194754643551));
#93111=CARTESIAN_POINT('Ctrl Pts',(-0.781208945056505,3.54052802843261,
3.00443733904289));
#93112=CARTESIAN_POINT('Ctrl Pts',(-0.583390951619396,-0.587155379019583,
4.60496137700709));
#93113=CARTESIAN_POINT('Ctrl Pts',(-0.385572958182286,-4.18466239345957,
2.01964576379865));
#93114=CARTESIAN_POINT('Ctrl Pts',(-0.187754964745179,-3.96652463206152,
-2.41173365972362));
#93115=CARTESIAN_POINT('Ctrl Pts',(-0.0558763024537767,-1.4269357426901,
-3.88994463893176));
#93116=CARTESIAN_POINT('Ctrl Pts',(0.0100630286919268,-0.124001864240948,
-3.93104471326196));
#93117=CARTESIAN_POINT('Ctrl Pts',(-1.54616352203498,-3.93676751258924,
0.00274060645320142));
#93118=CARTESIAN_POINT('Ctrl Pts',(-1.48899665647926,-3.92780616728942,
-1.12431394949728));
#93119=CARTESIAN_POINT('Ctrl Pts',(-1.43182979092354,-3.41813976225738,
-2.25845087457351));
#93120=CARTESIAN_POINT('Ctrl Pts',(-1.37466292536783,-2.56402239412072,
-2.99071767770299));
#93121=CARTESIAN_POINT('Ctrl Pts',(-1.30872359422213,-1.57883757722767,
-3.83535351262556));
#93122=CARTESIAN_POINT('Ctrl Pts',(-1.24278426307642,-0.13537612344502,
-4.1453190818819));
#93123=CARTESIAN_POINT('Ctrl Pts',(-1.17684493193072,1.10981214186687,-3.77974568239293));
#93124=CARTESIAN_POINT('Ctrl Pts',(-1.11090560078501,2.35500040717879,-3.41417228290396));
#93125=CARTESIAN_POINT('Ctrl Pts',(-1.04496626963931,3.40191548402005,-2.3730599146697));
#93126=CARTESIAN_POINT('Ctrl Pts',(-0.979026938493604,3.77398926703588,
-1.12977291630615));
#93127=CARTESIAN_POINT('Ctrl Pts',(-0.913087607347902,4.1460630500517,0.113514082057356));
#93128=CARTESIAN_POINT('Ctrl Pts',(-0.847148276202203,3.84329553924214,
1.55897571055012));
#93129=CARTESIAN_POINT('Ctrl Pts',(-0.781208945056502,3.003964549262,2.54846053112388));
#93130=CARTESIAN_POINT('Ctrl Pts',(-0.715269613910799,2.16463355928184,
3.53794535169766));
#93131=CARTESIAN_POINT('Ctrl Pts',(-0.649330282765096,0.78873909013109,
4.07145336435238));
#93132=CARTESIAN_POINT('Ctrl Pts',(-0.583390951619391,-0.498792646850961,
3.90732143514497));
#93133=CARTESIAN_POINT('Ctrl Pts',(-0.522260634412929,-1.69242355161679,
3.75515979319585));
#93134=CARTESIAN_POINT('Ctrl Pts',(-0.461130317206467,-2.8101104753617,
3.00340652247003));
#93135=CARTESIAN_POINT('Ctrl Pts',(-0.400000000000004,-3.41555626699893,
1.96277456085016));
#93136=CARTESIAN_POINT('',(-29.267,-1.87158653173899,-2.62360084935061));
#93137=CARTESIAN_POINT('Ctrl Pts',(-29.267,-1.87556211950935,-2.62715993178767));
#93138=CARTESIAN_POINT('Ctrl Pts',(-29.267,-1.94413804945346,-2.58901550230507));
#93139=CARTESIAN_POINT('Ctrl Pts',(-29.267,-2.01110052498262,-2.54827549470737));
#93140=CARTESIAN_POINT('Ctrl Pts',(-29.267,-2.07628315157793,-2.50497168480714));
#93141=CARTESIAN_POINT('Ctrl Pts',(-29.267,-2.16191037886223,-2.44808558852224));
#93142=CARTESIAN_POINT('Ctrl Pts',(-29.267,-2.24446748355392,-2.38677728024994));
#93143=CARTESIAN_POINT('Ctrl Pts',(-29.267,-2.32386237913326,-2.32143742155821));
#93144=CARTESIAN_POINT('Ctrl Pts',(-29.267,-2.37364457503314,-2.28046801638769));
#93145=CARTESIAN_POINT('Ctrl Pts',(-29.267,-2.42218320448196,-2.23791254568436));
#93146=CARTESIAN_POINT('Ctrl Pts',(-29.267,-2.46945134988874,-2.19385797799918));
#93147=CARTESIAN_POINT('Ctrl Pts',(-29.267,-2.49412738319863,-2.17085957240706));
#93148=CARTESIAN_POINT('Ctrl Pts',(-29.267,-2.51845711293783,-2.14745250715669));
#93149=CARTESIAN_POINT('Ctrl Pts',(-29.267,-2.54243628966495,-2.12364846865249));
#93150=CARTESIAN_POINT('Ctrl Pts',(-29.267,-2.55699647231938,-2.1091946301209));
#93151=CARTESIAN_POINT('Ctrl Pts',(-29.267,-2.57142234337411,-2.09459937375049));
#93152=CARTESIAN_POINT('Ctrl Pts',(-29.267,-2.58570771899918,-2.07987136520091));
#93153=CARTESIAN_POINT('Ctrl Pts',(-29.267,-2.65959479463748,-2.00369489562351));
#93154=CARTESIAN_POINT('Ctrl Pts',(-29.267,-2.72977136737143,-1.9239251248109));
#93155=CARTESIAN_POINT('Ctrl Pts',(-29.267,-2.79613899963645,-1.84096944342322));
#93156=CARTESIAN_POINT('Ctrl Pts',(-29.267,-2.85949750354379,-1.76177499751697));
#93157=CARTESIAN_POINT('Ctrl Pts',(-29.267,-2.91938482899898,-1.67967617064163));
#93158=CARTESIAN_POINT('Ctrl Pts',(-29.267,-2.97569370105063,-1.59499101459634));
#93159=CARTESIAN_POINT('Ctrl Pts',(-29.267,-3.00071677359493,-1.55735781886826));
#93160=CARTESIAN_POINT('Ctrl Pts',(-29.267,-3.02503285489035,-1.51921344645886));
#93161=CARTESIAN_POINT('Ctrl Pts',(-29.267,-3.048630913558,-1.48058395925084));
#93162=CARTESIAN_POINT('Ctrl Pts',(-29.267,-3.05877704718637,-1.46397496845512));
#93163=CARTESIAN_POINT('Ctrl Pts',(-29.267,-3.06879043196106,-1.44727628527374));
#93164=CARTESIAN_POINT('Ctrl Pts',(-29.267,-3.07867012826134,-1.43048992553262));
#93165=CARTESIAN_POINT('Ctrl Pts',(-29.267,-3.0873232258654,-1.4157876508025));
#93166=CARTESIAN_POINT('Ctrl Pts',(-29.267,-3.09586909840926,-1.40102604067025));
#93167=CARTESIAN_POINT('Ctrl Pts',(-29.267,-3.10430668639324,-1.38620798147017));
#93168=CARTESIAN_POINT('Ctrl Pts',(-29.267,-3.15937851519779,-1.28949104992148));
#93169=CARTESIAN_POINT('Ctrl Pts',(-29.267,-3.20984986675861,-1.19035556854987));
#93170=CARTESIAN_POINT('Ctrl Pts',(-29.267,-3.25561444260331,-1.08923039523438));
#93171=CARTESIAN_POINT('Ctrl Pts',(-29.267,-3.3020888475654,-0.986536725080546));
#93172=CARTESIAN_POINT('Ctrl Pts',(-29.267,-3.34370992002807,-0.881790488775369));
#93173=CARTESIAN_POINT('Ctrl Pts',(-29.267,-3.38033216148825,-0.775399491221893));
#93174=CARTESIAN_POINT('Ctrl Pts',(-29.267,-3.41685272414127,-0.669303880004472));
#93175=CARTESIAN_POINT('Ctrl Pts',(-29.267,-3.44840267319171,-0.561571812339358));
#93176=CARTESIAN_POINT('Ctrl Pts',(-29.267,-3.47479600376177,-0.45257833184847));
#93177=CARTESIAN_POINT('Ctrl Pts',(-29.267,-3.49203326148151,-0.381395624989836));
#93178=CARTESIAN_POINT('Ctrl Pts',(-29.267,-3.5070702109759,-0.309674316182991));
#93179=CARTESIAN_POINT('Ctrl Pts',(-29.267,-3.51984382259218,-0.237514625278931));
#93180=CARTESIAN_POINT('Ctrl Pts',(-29.267,-3.52358595661669,-0.216374853486772));
#93181=CARTESIAN_POINT('Ctrl Pts',(-29.267,-3.5271337783978,-0.195197442610527));
#93182=CARTESIAN_POINT('Ctrl Pts',(-29.267,-3.53048554423178,-0.1739848805149));
#93183=CARTESIAN_POINT('Ctrl Pts',(-29.267,-3.53317888328294,-0.156939351472193));
#93184=CARTESIAN_POINT('Ctrl Pts',(-29.267,-3.53574447963492,-0.139878128935328));
#93185=CARTESIAN_POINT('Ctrl Pts',(-29.267,-3.53818070904561,-0.122810384767));
#93186=CARTESIAN_POINT('Ctrl Pts',(-29.267,-3.55454810859626,-0.00814360215415144));
#93187=CARTESIAN_POINT('Ctrl Pts',(-29.267,-3.56509706882811,0.106923245517097));
#93188=CARTESIAN_POINT('Ctrl Pts',(-29.267,-3.56968323623,0.221965651223056));
#93189=CARTESIAN_POINT('Ctrl Pts',(-29.267,-3.57226426632728,0.286709888746834));
#93190=CARTESIAN_POINT('Ctrl Pts',(-29.267,-3.57295596462551,0.351446964375039));
#93191=CARTESIAN_POINT('Ctrl Pts',(-29.267,-3.57172621322166,0.416104672924591));
#93192=CARTESIAN_POINT('Ctrl Pts',(-29.267,-3.56961444125406,0.527137143370704));
#93193=CARTESIAN_POINT('Ctrl Pts',(-29.267,-3.56183970729814,0.637935324401442));
#93194=CARTESIAN_POINT('Ctrl Pts',(-29.267,-3.54866558297903,0.748214710453893));
#93195=CARTESIAN_POINT('Ctrl Pts',(-29.267,-3.53524477571288,0.860559056824879));
#93196=CARTESIAN_POINT('Ctrl Pts',(-29.267,-3.51622037619464,0.972365678151204));
#93197=CARTESIAN_POINT('Ctrl Pts',(-29.267,-3.49181697551176,1.08333660943036));
#93198=CARTESIAN_POINT('Ctrl Pts',(-29.267,-3.48335985307657,1.12179414921221));
#93199=CARTESIAN_POINT('Ctrl Pts',(-29.267,-3.474256248861,1.16015129842181));
#93200=CARTESIAN_POINT('Ctrl Pts',(-29.267,-3.46451407474897,1.19839549460657));
#93201=CARTESIAN_POINT('Ctrl Pts',(-29.267,-3.46095476509623,1.21236803657475));
#93202=CARTESIAN_POINT('Ctrl Pts',(-29.267,-3.45731047162383,1.2263243188045));
#93203=CARTESIAN_POINT('Ctrl Pts',(-29.267,-3.45358428768816,1.24025414023616));
#93204=CARTESIAN_POINT('Ctrl Pts',(-29.267,-3.4241337376961,1.35035093350684));
#93205=CARTESIAN_POINT('Ctrl Pts',(-29.267,-3.38953078097407,1.45895736979579));
#93206=CARTESIAN_POINT('Ctrl Pts',(-29.267,-3.35007714113598,1.565780445815));
#93207=CARTESIAN_POINT('Ctrl Pts',(-29.267,-3.30935323107808,1.67604285399249));
#93208=CARTESIAN_POINT('Ctrl Pts',(-29.267,-3.26346122728659,1.78440591486737));
#93209=CARTESIAN_POINT('Ctrl Pts',(-29.267,-3.21267761166844,1.89055080029088));
#93210=CARTESIAN_POINT('Ctrl Pts',(-29.267,-3.16141486757542,1.99769713148479));
#93211=CARTESIAN_POINT('Ctrl Pts',(-29.267,-3.10516751118045,2.10258403490618));
#93212=CARTESIAN_POINT('Ctrl Pts',(-29.267,-3.04416698925102,2.20487550184191));
#93213=CARTESIAN_POINT('Ctrl Pts',(-29.267,-3.00436620678509,2.27161723281168));
#93214=CARTESIAN_POINT('Ctrl Pts',(-29.267,-2.96254087141324,2.33725386583506));
#93215=CARTESIAN_POINT('Ctrl Pts',(-29.267,-2.91874414438408,2.40168772232732));
#93216=CARTESIAN_POINT('Ctrl Pts',(-29.267,-2.8943383194777,2.4375936341674));
#93217=CARTESIAN_POINT('Ctrl Pts',(-29.267,-2.8693201667382,2.473125974087));
#93218=CARTESIAN_POINT('Ctrl Pts',(-29.267,-2.84369778827627,2.50826717296835));
#93219=CARTESIAN_POINT('Ctrl Pts',(-29.267,-2.83388561980058,2.5217246029401));
#93220=CARTESIAN_POINT('Ctrl Pts',(-29.267,-2.82399066498491,2.5351166552739));
#93221=CARTESIAN_POINT('Ctrl Pts',(-29.267,-2.81401448605096,2.54844146066517));
#93222=CARTESIAN_POINT('Ctrl Pts',(-29.267,-2.74056959066549,2.64653903334034));
#93223=CARTESIAN_POINT('Ctrl Pts',(-29.267,-2.66271315483198,2.74101121591069));
#93224=CARTESIAN_POINT('Ctrl Pts',(-29.267,-2.58073485214103,2.8315238453715));
#93225=CARTESIAN_POINT('Ctrl Pts',(-29.267,-2.49861629012292,2.92219133581491));
#93226=CARTESIAN_POINT('Ctrl Pts',(-29.267,-2.41236136137793,3.00888654180042));
#93227=CARTESIAN_POINT('Ctrl Pts',(-29.267,-2.32221139231555,3.09125732425718));
#93228=CARTESIAN_POINT('Ctrl Pts',(-29.267,-2.2337606222272,3.17207553436702));
#93229=CARTESIAN_POINT('Ctrl Pts',(-29.267,-2.14155975600952,3.24873150750497));
#93230=CARTESIAN_POINT('Ctrl Pts',(-29.267,-2.04579561361836,3.32086577349601));
#93231=CARTESIAN_POINT('Ctrl Pts',(-29.267,-1.95025849965636,3.39282903049885));
#93232=CARTESIAN_POINT('Ctrl Pts',(-29.267,-1.85117460884397,3.4602927682777));
#93233=CARTESIAN_POINT('Ctrl Pts',(-29.267,-1.74869447533116,3.52286199445086));
#93234=CARTESIAN_POINT('Ctrl Pts',(-29.267,-1.87556211950935,-2.62715993178767));
#93235=CARTESIAN_POINT('Ctrl Pts',(-29.2058696827935,-1.06959153349225,
-3.19605863350378));
#93236=CARTESIAN_POINT('Ctrl Pts',(-29.0788000344414,1.19433685232607,-3.56810302549924));
#93237=CARTESIAN_POINT('Ctrl Pts',(-28.8857910549435,3.66252655955179,-1.03121985822236));
#93238=CARTESIAN_POINT('Ctrl Pts',(-28.6879730615064,2.8605553688775,2.50949297218581));
#93239=CARTESIAN_POINT('Ctrl Pts',(-28.4901550680693,-0.544644508144919,
3.76563167765424));
#93240=CARTESIAN_POINT('Ctrl Pts',(-28.3295728978095,-2.90640396394737,
2.00447016268953));
#93241=CARTESIAN_POINT('Ctrl Pts',(-28.2349300586953,-3.21932528384686,
0.467741112490102));
#93242=CARTESIAN_POINT('Ctrl Pts',(-28.2062265507269,-3.21789432005771,
0.00111814815214498));
#93243=CARTESIAN_POINT('Origin',(-29.267,-5.160062080289E-16,2.1385152528819E-16));
#93244=CARTESIAN_POINT('',(-29.267,-3.933,-4.81653586104654E-16));
#93245=CARTESIAN_POINT('Origin',(-29.267,0.,0.));
#93246=CARTESIAN_POINT('Origin',(-29.267,0.,0.));
#93247=CARTESIAN_POINT('',(-29.267,1.87158653173901,-2.62360084935059));
#93248=CARTESIAN_POINT('Ctrl Pts',(-29.267,1.752798395271,3.52791786994593));
#93249=CARTESIAN_POINT('Ctrl Pts',(-29.267,1.83395735182908,3.47886451957651));
#93250=CARTESIAN_POINT('Ctrl Pts',(-29.267,1.91309406069084,3.42675125683998));
#93251=CARTESIAN_POINT('Ctrl Pts',(-29.267,1.99001035894838,3.37156906414815));
#93252=CARTESIAN_POINT('Ctrl Pts',(-29.267,2.08883318098501,3.30067043626935));
#93253=CARTESIAN_POINT('Ctrl Pts',(-29.267,2.18399221922082,3.22470642798029));
#93254=CARTESIAN_POINT('Ctrl Pts',(-29.267,2.27530185738888,3.14408709844798));
#93255=CARTESIAN_POINT('Ctrl Pts',(-29.267,2.32778341860941,3.09774994978225));
#93256=CARTESIAN_POINT('Ctrl Pts',(-29.267,2.37899256877283,3.0498742455389));
#93257=CARTESIAN_POINT('Ctrl Pts',(-29.267,2.42888757139592,3.00053373763079));
#93258=CARTESIAN_POINT('Ctrl Pts',(-29.267,2.46017084034004,2.96959812689661));
#93259=CARTESIAN_POINT('Ctrl Pts',(-29.267,2.49093741259874,2.93808663944416));
#93260=CARTESIAN_POINT('Ctrl Pts',(-29.267,2.5211759780696,2.90601703563223));
#93261=CARTESIAN_POINT('Ctrl Pts',(-29.267,2.53506009770383,2.89129218976028));
#93262=CARTESIAN_POINT('Ctrl Pts',(-29.267,2.54883244835416,2.87645004363996));
#93263=CARTESIAN_POINT('Ctrl Pts',(-29.267,2.5624830469874,2.8615023243299));
#93264=CARTESIAN_POINT('Ctrl Pts',(-29.267,2.64596845224788,2.77008388636619));
#93265=CARTESIAN_POINT('Ctrl Pts',(-29.267,2.72499364171481,2.67462471248027));
#93266=CARTESIAN_POINT('Ctrl Pts',(-29.267,2.79936387127853,2.57555879213958));
#93267=CARTESIAN_POINT('Ctrl Pts',(-29.267,2.86443782214679,2.48887611184149));
#93268=CARTESIAN_POINT('Ctrl Pts',(-29.267,2.92594727850818,2.3994310409066));
#93269=CARTESIAN_POINT('Ctrl Pts',(-29.267,2.98372919602265,2.30749997840723));
#93270=CARTESIAN_POINT('Ctrl Pts',(-29.267,3.00900878493524,2.26728013856375));
#93271=CARTESIAN_POINT('Ctrl Pts',(-29.267,3.03357448870034,2.22658434219884));
#93272=CARTESIAN_POINT('Ctrl Pts',(-29.267,3.05741067291968,2.18543533259932));
#93273=CARTESIAN_POINT('Ctrl Pts',(-29.267,3.07143266131865,2.16122881825439));
#93274=CARTESIAN_POINT('Ctrl Pts',(-29.267,3.08520217217235,2.13686546385367));
#93275=CARTESIAN_POINT('Ctrl Pts',(-29.267,3.09871581841762,2.11234988443433));
#93276=CARTESIAN_POINT('Ctrl Pts',(-29.267,3.10919621461938,2.09333703025958));
#93277=CARTESIAN_POINT('Ctrl Pts',(-29.267,3.11952377181851,2.07423043659365));
#93278=CARTESIAN_POINT('Ctrl Pts',(-29.267,3.12968628263755,2.05505274587221));
#93279=CARTESIAN_POINT('Ctrl Pts',(-29.267,3.18534814899617,1.95001314719307));
#93280=CARTESIAN_POINT('Ctrl Pts',(-29.267,3.23613492547288,1.84271397680196));
#93281=CARTESIAN_POINT('Ctrl Pts',(-29.267,3.28187401835454,1.73353344117171));
#93282=CARTESIAN_POINT('Ctrl Pts',(-29.267,3.32728770285637,1.62512966474171));
#93283=CARTESIAN_POINT('Ctrl Pts',(-29.267,3.36772549975111,1.51487033063548));
#93284=CARTESIAN_POINT('Ctrl Pts',(-29.267,3.40296884306188,1.40311370918593));
#93285=CARTESIAN_POINT('Ctrl Pts',(-29.267,3.43717304060426,1.29465221837269));
#93286=CARTESIAN_POINT('Ctrl Pts',(-29.267,3.46648459568988,1.18477969669452));
#93287=CARTESIAN_POINT('Ctrl Pts',(-29.267,3.49065535521413,1.07382410402513));
#93288=CARTESIAN_POINT('Ctrl Pts',(-29.267,3.50713741723422,0.998163388522294));
#93289=CARTESIAN_POINT('Ctrl Pts',(-29.267,3.52122807768353,0.921999073055619));
#93290=CARTESIAN_POINT('Ctrl Pts',(-29.267,3.53283505631117,0.845437826880077));
#93291=CARTESIAN_POINT('Ctrl Pts',(-29.267,3.53650941868402,0.821201221369631));
#93292=CARTESIAN_POINT('Ctrl Pts',(-29.267,3.53993479734101,0.796924862307499));
#93293=CARTESIAN_POINT('Ctrl Pts',(-29.267,3.54310802391695,0.772612209064599));
#93294=CARTESIAN_POINT('Ctrl Pts',(-29.267,3.54518371661638,0.756708649822146));
#93295=CARTESIAN_POINT('Ctrl Pts',(-29.267,3.54715182636697,0.740786860054947));
#93296=CARTESIAN_POINT('Ctrl Pts',(-29.267,3.54901039433523,0.724856886056574));
#93297=CARTESIAN_POINT('Ctrl Pts',(-29.267,3.56199475275373,0.613566637045098));
#93298=CARTESIAN_POINT('Ctrl Pts',(-29.267,3.56961554007749,0.502076700900192));
#93299=CARTESIAN_POINT('Ctrl Pts',(-29.267,3.57168257316973,0.390705415856302));
#93300=CARTESIAN_POINT('Ctrl Pts',(-29.267,3.57315383999081,0.311433885506525));
#93301=CARTESIAN_POINT('Ctrl Pts',(-29.267,3.57181041061219,0.232222349124384));
#93302=CARTESIAN_POINT('Ctrl Pts',(-29.267,3.56756762581781,0.153187282053559));
#93303=CARTESIAN_POINT('Ctrl Pts',(-29.267,3.56149580005725,0.0400806364220606));
#93304=CARTESIAN_POINT('Ctrl Pts',(-29.267,3.54948772715183,-0.0726657673483353));
#93305=CARTESIAN_POINT('Ctrl Pts',(-29.267,3.53175700430858,-0.184693834183496));
#93306=CARTESIAN_POINT('Ctrl Pts',(-29.267,3.51395987864282,-0.297141454124599));
#93307=CARTESIAN_POINT('Ctrl Pts',(-29.267,3.49039661484532,-0.408866144611942));
#93308=CARTESIAN_POINT('Ctrl Pts',(-29.267,3.46123882223617,-0.519478579222817));
#93309=CARTESIAN_POINT('Ctrl Pts',(-29.267,3.45486906339251,-0.543642772412126));
#93310=CARTESIAN_POINT('Ctrl Pts',(-29.267,3.44823216157597,-0.567753755563771));
#93311=CARTESIAN_POINT('Ctrl Pts',(-29.267,3.44132966501532,-0.591807239612535));
#93312=CARTESIAN_POINT('Ctrl Pts',(-29.267,3.43531557970422,-0.612764831380591));
#93313=CARTESIAN_POINT('Ctrl Pts',(-29.267,3.42909832027748,-0.633683474481864));
#93314=CARTESIAN_POINT('Ctrl Pts',(-29.267,3.42268802028739,-0.654531474620821));
#93315=CARTESIAN_POINT('Ctrl Pts',(-29.267,3.38997005995087,-0.760938981710492));
#93316=CARTESIAN_POINT('Ctrl Pts',(-29.267,3.35219258588973,-0.865637661248984));
#93317=CARTESIAN_POINT('Ctrl Pts',(-29.267,3.30959231005111,-0.968301959519508));
#93318=CARTESIAN_POINT('Ctrl Pts',(-29.267,3.26694576890514,-1.07107775461064));
#93319=CARTESIAN_POINT('Ctrl Pts',(-29.267,3.21946535835239,-1.1718154969129));
#93320=CARTESIAN_POINT('Ctrl Pts',(-29.267,3.16734388272138,-1.27016148531058));
#93321=CARTESIAN_POINT('Ctrl Pts',(-29.267,3.11585673221232,-1.36731059026764));
#93322=CARTESIAN_POINT('Ctrl Pts',(-29.267,3.05984017368962,-1.46212642571529));
#93323=CARTESIAN_POINT('Ctrl Pts',(-29.267,2.9994455855754,-1.55423154140084));
#93324=CARTESIAN_POINT('Ctrl Pts',(-29.267,2.96352940982248,-1.60900571282907));
#93325=CARTESIAN_POINT('Ctrl Pts',(-29.267,2.9260642937352,-1.6628204737105));
#93326=CARTESIAN_POINT('Ctrl Pts',(-29.267,2.88707751446442,-1.71558884474527));
#93327=CARTESIAN_POINT('Ctrl Pts',(-29.267,2.86858036962461,-1.74062461892943));
#93328=CARTESIAN_POINT('Ctrl Pts',(-29.267,2.84974065503184,-1.76542476192336));
#93329=CARTESIAN_POINT('Ctrl Pts',(-29.267,2.83056106449946,-1.78997947648368));
#93330=CARTESIAN_POINT('Ctrl Pts',(-29.267,2.82019641614239,-1.80324884120218));
#93331=CARTESIAN_POINT('Ctrl Pts',(-29.267,2.80973696569548,-1.81644076475104));
#93332=CARTESIAN_POINT('Ctrl Pts',(-29.267,2.79918811988956,-1.82954813134034));
#93333=CARTESIAN_POINT('Ctrl Pts',(-29.267,2.73178606534395,-1.91329790397479));
#93334=CARTESIAN_POINT('Ctrl Pts',(-29.267,2.66067793855252,-1.99367458528833));
#93335=CARTESIAN_POINT('Ctrl Pts',(-29.267,2.58603966220747,-2.07035807397434));
#93336=CARTESIAN_POINT('Ctrl Pts',(-29.267,2.51244806685979,-2.14596620087079));
#93337=CARTESIAN_POINT('Ctrl Pts',(-29.267,2.43542404680641,-2.21798450045409));
#93338=CARTESIAN_POINT('Ctrl Pts',(-29.267,2.35510789090453,-2.28606528024848));
#93339=CARTESIAN_POINT('Ctrl Pts',(-29.267,2.2772577781145,-2.35205569433528));
#93340=CARTESIAN_POINT('Ctrl Pts',(-29.267,2.19631404788083,-2.41434695939189));
#93341=CARTESIAN_POINT('Ctrl Pts',(-29.267,2.11238597055247,-2.47257820210255));
#93342=CARTESIAN_POINT('Ctrl Pts',(-29.267,2.03465401232407,-2.52651043396178));
#93343=CARTESIAN_POINT('Ctrl Pts',(-29.267,1.95436164731551,-2.57695984678878));
#93344=CARTESIAN_POINT('Ctrl Pts',(-29.267,1.87158653173901,-2.62360084935059));
#93345=CARTESIAN_POINT('Origin',(-29.267,0.,0.));
#93346=CARTESIAN_POINT('Origin',(-31.5777734492731,0.,0.));
#93347=CARTESIAN_POINT('Ctrl Pts',(-29.267,1.871586531739,-2.6236008493506));
#93348=CARTESIAN_POINT('Ctrl Pts',(-29.2010606688543,2.74117176403474,-2.0032686790181));
#93349=CARTESIAN_POINT('Ctrl Pts',(-29.069182006563,3.80053009112415,0.158992474904673));
#93350=CARTESIAN_POINT('Ctrl Pts',(-28.8713640131257,1.93474699165479,3.27922584988832));
#93351=CARTESIAN_POINT('Ctrl Pts',(-28.6735460196887,-1.69312072237911,
3.40633319030359));
#93352=CARTESIAN_POINT('Ctrl Pts',(-28.5340158317378,-3.16477800868145,
1.31315271293012));
#93353=CARTESIAN_POINT('Ctrl Pts',(-28.4604249749326,-3.22715455055888,
0.12579512260648));
#93354=CARTESIAN_POINT('Ctrl Pts',(-28.4527734492731,-3.22624365146105,
0.0022389224034757));
#93355=CARTESIAN_POINT('Ctrl Pts',(-29.6770630286919,2.28405859260864,-3.20180657528381));
#93356=CARTESIAN_POINT('Ctrl Pts',(-29.6111236975462,3.34528851072799,-2.44476168321409));
#93357=CARTESIAN_POINT('Ctrl Pts',(-29.4792450352549,4.63811491688505,0.194032240726105));
#93358=CARTESIAN_POINT('Ctrl Pts',(-29.2814270418177,2.36113875360431,4.00192235439013));
#93359=CARTESIAN_POINT('Ctrl Pts',(-29.0836090483806,-2.06626136098581,
4.15704241330045));
#93360=CARTESIAN_POINT('Ctrl Pts',(-28.8857910549435,-4.61251479306561,
0.535432936636152));
#93361=CARTESIAN_POINT('Ctrl Pts',(-28.6879730615064,-2.96244924208781,
-3.57632094417714));
#93362=CARTESIAN_POINT('Ctrl Pts',(-28.4901550680693,1.38341358179131,-4.4324734582532));
#93363=CARTESIAN_POINT('Ctrl Pts',(-28.2923370746322,4.47036851547105,-1.25636722700296));
#93364=CARTESIAN_POINT('Ctrl Pts',(-28.0945190811951,3.489859458072,3.06331556440806));
#93365=CARTESIAN_POINT('Ctrl Pts',(-27.896701087758,-0.666080140453031,
4.59549820331548));
#93366=CARTESIAN_POINT('Ctrl Pts',(-27.6988830943208,-4.2159381251684,1.94639706903792));
#93367=CARTESIAN_POINT('Ctrl Pts',(-27.5010651008838,-3.92976705706495,
-2.47377142775801));
#93368=CARTESIAN_POINT('Ctrl Pts',(-27.3032471074466,-0.0679337783385457,
-4.64304845044703));
#93369=CARTESIAN_POINT('Ctrl Pts',(-27.1054291140096,3.8557086591862,-2.58767786462851));
#93370=CARTESIAN_POINT('Ctrl Pts',(-26.9076111205724,4.27108148336715,1.82220379196051));
#93371=CARTESIAN_POINT('Ctrl Pts',(-26.7097931271353,0.800238585829137,
4.57407575421308));
#93372=CARTESIAN_POINT('Ctrl Pts',(-26.5119751336982,-3.39873305617157,
3.16404367576156));
#93373=CARTESIAN_POINT('Ctrl Pts',(-26.3141571402611,-4.50523127888368,
-1.12492171884469));
#93374=CARTESIAN_POINT('Ctrl Pts',(-26.116339146824,-1.51246392145779,-4.3903313135453));
#93375=CARTESIAN_POINT('Ctrl Pts',(-25.9185211533869,2.8564793618577,-3.66102212460931));
#93376=CARTESIAN_POINT('Ctrl Pts',(-25.7207031599498,4.62634030974878,0.39941512218846));
#93377=CARTESIAN_POINT('Ctrl Pts',(-25.5228851665127,2.18673986986448,4.09642840245587));
#93378=CARTESIAN_POINT('Ctrl Pts',(-25.3250671730756,-2.24255357823703,
4.06614197186242));
#93379=CARTESIAN_POINT('Ctrl Pts',(-25.1272491796384,-4.63136967163741,
0.336113082707444));
#93380=CARTESIAN_POINT('Ctrl Pts',(-24.9294311862014,-2.80614822532237,
-3.69974176897582));
#93381=CARTESIAN_POINT('Ctrl Pts',(-24.7316131927642,1.57235978395034,-4.36923812050275));
#93382=CARTESIAN_POINT('Ctrl Pts',(-24.5337951993272,4.52019315087723,-1.06320784152848));
#93383=CARTESIAN_POINT('Ctrl Pts',(-24.33597720589,3.35514739875397,3.21022475323414));
#93384=CARTESIAN_POINT('Ctrl Pts',(-24.1381592124529,-0.862713844891543,
4.5627055415416));
#93385=CARTESIAN_POINT('Ctrl Pts',(-23.9403412190158,-4.29560027900972,
1.76362560612109));
#93386=CARTESIAN_POINT('Ctrl Pts',(-23.7425232255787,-3.81996243101423,
-2.64015985521965));
#93387=CARTESIAN_POINT('Ctrl Pts',(-23.5447052321416,0.131421517249421,
-4.64168993155775));
#93388=CARTESIAN_POINT('Ctrl Pts',(-23.3468872387045,3.96322632454721,-2.41979216795887));
#93389=CARTESIAN_POINT('Ctrl Pts',(-23.1490692452674,4.18893062930736,2.0038505978625));
#93390=CARTESIAN_POINT('Ctrl Pts',(-22.9512512518303,0.603168313088729,
4.60420948935287));
#93391=CARTESIAN_POINT('Ctrl Pts',(-22.7534332583932,-3.53141089594158,
3.01524362527346));
#93392=CARTESIAN_POINT('Ctrl Pts',(-22.555615264956,-4.45279419747962,-1.31726264299215));
#93393=CARTESIAN_POINT('Ctrl Pts',(-22.357797271519,-1.32262402256341,-4.45120463814867));
#93394=CARTESIAN_POINT('Ctrl Pts',(-22.1599792780818,3.01098869180223,-3.53503948118999));
#93395=CARTESIAN_POINT('Ctrl Pts',(-21.9621612846447,4.60493252393142,0.597623197150572));
#93396=CARTESIAN_POINT('Ctrl Pts',(-21.7643432912076,2.00889371847677,4.18651442892525));
#93397=CARTESIAN_POINT('Ctrl Pts',(-21.5665252977705,-2.41501764698298,
3.96613751658901));
#93398=CARTESIAN_POINT('Ctrl Pts',(-21.3687073043334,-4.64152829967862,
0.137011236826592));
#93399=CARTESIAN_POINT('Ctrl Pts',(-21.1708893108963,-2.64475817975951,
-3.81678021456953));
#93400=CARTESIAN_POINT('Ctrl Pts',(-20.9730713174592,1.7584512953968,-4.29772103299545));
#93401=CARTESIAN_POINT('Ctrl Pts',(-20.7752533240221,4.56166329861203,-0.868207916244836));
#93402=CARTESIAN_POINT('Ctrl Pts',(-20.577435330585,3.21426290515085,3.35127901140825));
#93403=CARTESIAN_POINT('Ctrl Pts',(-20.3796173371479,-1.05776357028257,
4.52147025480841));
#93404=CARTESIAN_POINT('Ctrl Pts',(-20.1817993437108,-4.36734141674695,
1.57762035525057));
#93405=CARTESIAN_POINT('Ctrl Pts',(-19.9839813502736,-3.70311842824315,
-2.80169072920981));
#93406=CARTESIAN_POINT('Ctrl Pts',(-19.7861633568366,0.330535456070876,
-4.63177108113238));
#93407=CARTESIAN_POINT('Ctrl Pts',(-19.5883453633994,4.06343839238611,-2.24744865725935));
#93408=CARTESIAN_POINT('Ctrl Pts',(-19.3905273699623,4.09905885506931,2.18180511008938));
#93409=CARTESIAN_POINT('Ctrl Pts',(-19.1927093765252,0.404986136817035,
4.62585594941305));
#93410=CARTESIAN_POINT('Ctrl Pts',(-18.9948913830881,-3.65757946877007,
2.86088613289063));
#93411=CARTESIAN_POINT('Ctrl Pts',(-18.797073389651,-4.3921496281511,-1.50717572952404));
#93412=CARTESIAN_POINT('Ctrl Pts',(-18.5992553962139,-1.13034620594656,
-4.50387327646287));
#93413=CARTESIAN_POINT('Ctrl Pts',(-18.4014374027768,3.15994806878659,-3.40254099729982));
#93414=CARTESIAN_POINT('Ctrl Pts',(-18.2036194093397,4.57503679488795,0.794729740953231));
#93415=CARTESIAN_POINT('Ctrl Pts',(-18.0058014159026,1.82734471209214,4.26888373452864));
#93416=CARTESIAN_POINT('Ctrl Pts',(-17.8079834224655,-2.58303028228958,
3.85882256608273));
#93417=CARTESIAN_POINT('Ctrl Pts',(-17.6101654290284,-4.64313152588309,
-0.0623431558779312));
#93418=CARTESIAN_POINT('Ctrl Pts',(-17.4123474355912,-2.47849323716755,
-3.92678345583875));
#93419=CARTESIAN_POINT('Ctrl Pts',(-17.2145294421541,1.94130157710662,-4.218282259695));
#93420=CARTESIAN_POINT('Ctrl Pts',(-17.016711448717,4.59472525345006,-0.671607683876884));
#93421=CARTESIAN_POINT('Ctrl Pts',(-16.8188934552799,3.067453786841,3.48615609250776));
#93422=CARTESIAN_POINT('Ctrl Pts',(-16.6210754618428,-1.25086359448258,
4.47190086023073));
#93423=CARTESIAN_POINT('Ctrl Pts',(-16.4232574684057,-4.43103254135455,
1.38870718770775));
#93424=CARTESIAN_POINT('Ctrl Pts',(-16.2254394749686,-3.57944872782031,
-2.95805744376943));
#93425=CARTESIAN_POINT('Ctrl Pts',(-16.0276214815315,0.529040142139094,
-4.61331481298855));
#93426=CARTESIAN_POINT('Ctrl Pts',(-15.8298034880944,4.15616061014518,-2.07096258257165));
#93427=CARTESIAN_POINT('Ctrl Pts',(-15.6319854946573,4.00163157405578,2.3557380544649));
#93428=CARTESIAN_POINT('Ctrl Pts',(-15.4341675012202,0.206057478095051,
4.63897589468358));
#93429=CARTESIAN_POINT('Ctrl Pts',(-15.236349507783,-3.77700628271434,2.70125537039182));
#93430=CARTESIAN_POINT('Ctrl Pts',(-15.038531514346,-4.32340931844811,-1.69431074507903));
#93431=CARTESIAN_POINT('Ctrl Pts',(-14.8407135209088,-0.935984901700447,
-4.54824024206318));
#93432=CARTESIAN_POINT('Ctrl Pts',(-14.6428955274718,3.30308293583232,-3.26377084899469));
#93433=CARTESIAN_POINT('Ctrl Pts',(-14.4450775340346,4.53670822242377,0.99037141534212));
#93434=CARTESIAN_POINT('Ctrl Pts',(-14.2472595405975,1.64242748977322,4.34338450710635));
#93435=CARTESIAN_POINT('Ctrl Pts',(-14.0494415471604,-2.7462817996209,3.7443949194503));
#93436=CARTESIAN_POINT('Ctrl Pts',(-13.8516235537233,-4.63617639444042,
-0.261582635829614));
#93437=CARTESIAN_POINT('Ctrl Pts',(-13.6538055602862,-2.30765986238043,
-4.02954873345547));
#93438=CARTESIAN_POINT('Ctrl Pts',(-13.4559875668491,2.12057359421086,-4.13106822350708));
#93439=CARTESIAN_POINT('Ctrl Pts',(-13.258169573412,4.61931807451703,-0.473769524320169));
#93440=CARTESIAN_POINT('Ctrl Pts',(-13.0603515799749,2.91499064679445,3.61460738737074));
#93441=CARTESIAN_POINT('Ctrl Pts',(-12.8625335865378,-1.44165798983063,
4.41408872544398));
#93442=CARTESIAN_POINT('Ctrl Pts',(-12.6647155931007,-4.48655625544975,
1.19723431391644));
#93443=CARTESIAN_POINT('Ctrl Pts',(-12.4668975996636,-3.44918128141044,
-3.10897177917426));
#93444=CARTESIAN_POINT('Ctrl Pts',(-12.2690796062264,0.726569685736974,
-4.58635514624655));
#93445=CARTESIAN_POINT('Ctrl Pts',(-12.0712616127894,4.24122206948244,-1.89065924827013));
#93446=CARTESIAN_POINT('Ctrl Pts',(-11.8734436193522,3.89682836711986,2.52532883263629));
#93447=CARTESIAN_POINT('Ctrl Pts',(-11.6756256259152,0.00674900812206685,
4.64354514208956));
#93448=CARTESIAN_POINT('Ctrl Pts',(-11.477807632478,-3.88947120673092,2.5366455739313));
#93449=CARTESIAN_POINT('Ctrl Pts',(-11.2799896390409,-4.24669997254704,
-1.8783227568507));
#93450=CARTESIAN_POINT('Ctrl Pts',(-11.0821716456038,-0.739898362341693,
-4.58422375644321));
#93451=CARTESIAN_POINT('Ctrl Pts',(-10.8843536521667,3.44012946251005,-3.11898482152518));
#93452=CARTESIAN_POINT('Ctrl Pts',(-10.6865356587296,4.49001745489969,1.18418760778445));
#93453=CARTESIAN_POINT('Ctrl Pts',(-10.4887176652925,1.45448289642492,4.40987942462621));
#93454=CARTESIAN_POINT('Ctrl Pts',(-10.2908996718554,-2.90447128894164,
3.62306549312152));
#93455=CARTESIAN_POINT('Ctrl Pts',(-10.0930816784183,-4.62067572525506,
-0.460339958913909));
#93456=CARTESIAN_POINT('Ctrl Pts',(-9.89526368498118,-2.13257294053773,
-4.1248866274142));
#93457=CARTESIAN_POINT('Ctrl Pts',(-9.69744569154406,2.29593690721424,-4.03623967992807));
#93458=CARTESIAN_POINT('Ctrl Pts',(-9.49962769810695,4.63539643159623,-0.275058098734038));
#93459=CARTESIAN_POINT('Ctrl Pts',(-9.30180970466984,2.75715450958978,3.73639613076329));
#93460=CARTESIAN_POINT('Ctrl Pts',(-9.10399171123273,-1.62979507844226,
4.34814041148852));
#93461=CARTESIAN_POINT('Ctrl Pts',(-8.90617371779562,-4.53381021607703,
1.00355466235267));
#93462=CARTESIAN_POINT('Ctrl Pts',(-8.70835572435853,-3.31255620183176,
-3.25415556564835));
#93463=CARTESIAN_POINT('Ctrl Pts',(-8.5105377309214,0.922759994555157,-4.55094177376315));
#93464=CARTESIAN_POINT('Ctrl Pts',(-8.31271973748432,4.3184659825949,-1.70687099480464));
#93465=CARTESIAN_POINT('Ctrl Pts',(-8.11490174404719,3.78484241063877,2.69026484985475));
#93466=CARTESIAN_POINT('Ctrl Pts',(-7.91708375061009,-0.192571901822546,
4.63955526945863));
#93467=CARTESIAN_POINT('Ctrl Pts',(-7.71926575717298,-3.99476694213886,
2.36736015716507));
#93468=CARTESIAN_POINT('Ctrl Pts',(-7.52144776373589,-4.1621629833872,-2.05887258844547));
#93469=CARTESIAN_POINT('Ctrl Pts',(-7.32362977029875,-0.542448020392725,
-4.6117574937218));
#93470=CARTESIAN_POINT('Ctrl Pts',(-7.12581177686167,3.57083504060222,-2.96844978879022));
#93471=CARTESIAN_POINT('Ctrl Pts',(-6.92799378342454,4.43505055411778,1.37582107053309));
#93472=CARTESIAN_POINT('Ctrl Pts',(-6.73017578998745,1.2638573571009,4.468245921679));
#93473=CARTESIAN_POINT('Ctrl Pts',(-6.53235779655033,-3.05730717071301,
3.49505792510332));
#93474=CARTESIAN_POINT('Ctrl Pts',(-6.33453980311323,-4.59665808958816,
-0.658248769765227));
#93475=CARTESIAN_POINT('Ctrl Pts',(-6.13672180967612,-1.95355519710399,
-4.21262140803828));
#93476=CARTESIAN_POINT('Ctrl Pts',(-5.938903816239,2.46706828137679,-3.93397141982583));
#93477=CARTESIAN_POINT('Ctrl Pts',(-5.74108582280191,4.6429306883608,-0.0758396777437203));
#93478=CARTESIAN_POINT('Ctrl Pts',(-5.54326782936478,2.59423630389935,3.85129783774972));
#93479=CARTESIAN_POINT('Ctrl Pts',(-5.3454498359277,-1.8149280812755,4.27417747685288));
#93480=CARTESIAN_POINT('Ctrl Pts',(-5.14763184249057,-4.57270732177326,
0.808025227938727));
#93481=CARTESIAN_POINT('Ctrl Pts',(-4.94981384905348,-3.16982532347193,
-3.3933411939276));
#93482=CARTESIAN_POINT('Ctrl Pts',(-4.75199585561636,1.11724945052968,-4.50713997473964));
#93483=CARTESIAN_POINT('Ctrl Pts',(-4.55417786217926,4.38774996024445,-1.51993657804425));
#93484=CARTESIAN_POINT('Ctrl Pts',(-4.35635986874214,3.66588014144792,2.85024207568007));
#93485=CARTESIAN_POINT('Ctrl Pts',(-4.15854187530505,-0.391537897742414,
4.62701366069188));
#93486=CARTESIAN_POINT('Ctrl Pts',(-3.96072388186793,-4.09269932772028,
2.19371109521874));
#93487=CARTESIAN_POINT('Ctrl Pts',(-3.76290588843083,-4.06995431948468,
-2.23562733635738));
#93488=CARTESIAN_POINT('Ctrl Pts',(-3.56508789499372,-0.343997539878338,
-4.63079091104292));
#93489=CARTESIAN_POINT('Ctrl Pts',(-3.36726990155661,3.69495820917957,-2.81244282287592));
#93490=CARTESIAN_POINT('Ctrl Pts',(-3.1694519081195,4.37190987169366,1.56491781598413));
#93491=CARTESIAN_POINT('Ctrl Pts',(-2.9716339146824,1.07090025667334,4.51837787661333));
#93492=CARTESIAN_POINT('Ctrl Pts',(-2.77381592124529,-3.20450393868088,
3.36060536487351));
#93493=CARTESIAN_POINT('Ctrl Pts',(-2.57599792780818,-4.56417502327569,
-0.854938919742906));
#93494=CARTESIAN_POINT('Ctrl Pts',(-2.37817993437107,-1.7709226905566,-4.29260161786294));
#93495=CARTESIAN_POINT('Ctrl Pts',(-2.18036194093397,2.6336256434247,-3.82443230564715));
#93496=CARTESIAN_POINT('Ctrl Pts',(-1.98254394749686,4.64195796464309,0.12348092454259));
#93497=CARTESIAN_POINT('Ctrl Pts',(-1.78472595405975,2.42643865805515,3.95917273074786));
#93498=CARTESIAN_POINT('Ctrl Pts',(-1.58690796062265,-1.9965287407846,4.19219835928893));
#93499=CARTESIAN_POINT('Ctrl Pts',(-1.38908996718554,-4.60353401029951,
0.611270499633702));
#93500=CARTESIAN_POINT('Ctrl Pts',(-1.19127197374843,-3.0205655885075,-3.52677822827127));
#93501=CARTESIAN_POINT('Ctrl Pts',(-0.993453980311325,1.30836214558254,
-4.45405726657038));
#93502=CARTESIAN_POINT('Ctrl Pts',(-0.79563598687421,4.45150143479259,-1.33210124254099));
#93503=CARTESIAN_POINT('Ctrl Pts',(-0.597817993437107,3.53497485386071,
3.00893856288978));
#93504=CARTESIAN_POINT('Ctrl Pts',(-0.465939331145702,0.793490219260556,
4.06671712560122));
#93505=CARTESIAN_POINT('Ctrl Pts',(-0.4,-0.4995344189117,3.90114782651498));
#93506=CARTESIAN_POINT('Ctrl Pts',(-29.5403753524613,2.14656790565209,-3.00907133330607));
#93507=CARTESIAN_POINT('Ctrl Pts',(-29.4744360213156,3.14391626183024,-2.29759734848209));
#93508=CARTESIAN_POINT('Ctrl Pts',(-29.3425573590242,4.35891997496475,0.182352318785631));
#93509=CARTESIAN_POINT('Ctrl Pts',(-29.1447393655871,2.21900816628781,3.76102351955619));
#93510=CARTESIAN_POINT('Ctrl Pts',(-28.94692137215,-1.94188114811691,3.90680600563483));
#93511=CARTESIAN_POINT('Ctrl Pts',(-28.7491033787128,-4.33486087054888,
0.503202133750661));
#93512=CARTESIAN_POINT('Ctrl Pts',(-28.5512853852758,-2.78412230131377,
-3.36104151790357));
#93513=CARTESIAN_POINT('Ctrl Pts',(-28.3534673918386,1.30013792313657,-4.16565726419232));
#93514=CARTESIAN_POINT('Ctrl Pts',(-28.1556493984015,4.2012711989092,-1.18073922268235));
#93515=CARTESIAN_POINT('Ctrl Pts',(-27.9578314049644,3.27978464833425,2.87891689675649));
#93516=CARTESIAN_POINT('Ctrl Pts',(-27.7600134115273,-0.62598492731999,
4.31886860767985));
#93517=CARTESIAN_POINT('Ctrl Pts',(-27.5621954180902,-3.96215644422926,
1.82923218063347));
#93518=CARTESIAN_POINT('Ctrl Pts',(-27.3643774246531,-3.69321166658437,
-2.32486082884581));
#93519=CARTESIAN_POINT('Ctrl Pts',(-27.166559431216,-0.0638444516104365,
-4.36355653062925));
#93520=CARTESIAN_POINT('Ctrl Pts',(-26.9687414377789,3.62361127167989,-2.43191057898122));
#93521=CARTESIAN_POINT('Ctrl Pts',(-26.7709234443418,4.01398040500783,1.71251481465396));
#93522=CARTESIAN_POINT('Ctrl Pts',(-26.5731054509047,0.752067600526557,
4.29873569959576));
#93523=CARTESIAN_POINT('Ctrl Pts',(-26.3752874574676,-3.19414367121133,
2.97358160094932));
#93524=CARTESIAN_POINT('Ctrl Pts',(-26.1774694640304,-4.23403537110954,
-1.05720617932359));
#93525=CARTESIAN_POINT('Ctrl Pts',(-25.9796514705933,-1.42141997703747,
-4.12605189872662));
#93526=CARTESIAN_POINT('Ctrl Pts',(-25.7818334771563,2.6845313606068,-3.44064404477171));
#93527=CARTESIAN_POINT('Ctrl Pts',(-25.5840154837191,4.34785414948105,0.375372017642794));
#93528=CARTESIAN_POINT('Ctrl Pts',(-25.3861974902821,2.05510735926432,3.84984070240973));
#93529=CARTESIAN_POINT('Ctrl Pts',(-25.1883794968449,-2.10756131796558,
3.82137738710818));
#93530=CARTESIAN_POINT('Ctrl Pts',(-24.9905615034079,-4.35258076501138,
0.31588049375982));
#93531=CARTESIAN_POINT('Ctrl Pts',(-24.7927435099707,-2.63722994605843,
-3.47703292997124));
#93532=CARTESIAN_POINT('Ctrl Pts',(-24.5949255165336,1.47771036141024,-4.10622842687727));
#93533=CARTESIAN_POINT('Ctrl Pts',(-24.3971075230965,4.2480966015586,-0.999207216946258));
#93534=CARTESIAN_POINT('Ctrl Pts',(-24.1992895296594,3.15318168640843,3.01698277247436));
#93535=CARTESIAN_POINT('Ctrl Pts',(-24.0014715362223,-0.810782112682527,
4.28804992573688));
#93536=CARTESIAN_POINT('Ctrl Pts',(-23.8036535427852,-4.03702327263912,
1.65746278836132));
#93537=CARTESIAN_POINT('Ctrl Pts',(-23.6058355493481,-3.59001681556988,
-2.48123337524934));
#93538=CARTESIAN_POINT('Ctrl Pts',(-23.4080175559109,0.123510496601368,
-4.36227978884321));
#93539=CARTESIAN_POINT('Ctrl Pts',(-23.2101995624739,3.72465682738561,-2.27413089265649));
#93540=CARTESIAN_POINT('Ctrl Pts',(-23.0123815690367,3.93677468562862,1.88322724951672));
#93541=CARTESIAN_POINT('Ctrl Pts',(-22.8145635755996,0.566860126431276,
4.32705551106549));
#93542=CARTESIAN_POINT('Ctrl Pts',(-22.6167455821625,-3.31883486502011,
2.83373868546072));
#93543=CARTESIAN_POINT('Ctrl Pts',(-22.4189275887254,-4.18475478068498,
-1.23796899165007));
#93544=CARTESIAN_POINT('Ctrl Pts',(-22.2211095952883,-1.2430076387999,-4.18326090611671));
#93545=CARTESIAN_POINT('Ctrl Pts',(-22.0232916018512,2.82973988102568,-3.32224502475171));
#93546=CARTESIAN_POINT('Ctrl Pts',(-21.8254736084141,4.32773502201412,0.561648803068342));
#93547=CARTESIAN_POINT('Ctrl Pts',(-21.627655614977,1.88796679555549,3.93450393031146));
#93548=CARTESIAN_POINT('Ctrl Pts',(-21.4298376215398,-2.26964377769154,
3.72739277795376));
#93549=CARTESIAN_POINT('Ctrl Pts',(-21.2320196281028,-4.362127886521,0.128763738652503));
#93550=CARTESIAN_POINT('Ctrl Pts',(-21.0342016346657,-2.48555490006003,
-3.58702615512398));
#93551=CARTESIAN_POINT('Ctrl Pts',(-20.8363836412285,1.65259994930344,-4.03901636618597));
#93552=CARTESIAN_POINT('Ctrl Pts',(-20.6385656477914,4.28707042143268,-0.815945464129155));
#93553=CARTESIAN_POINT('Ctrl Pts',(-20.4407476543543,3.02077784468951,3.14954615965363));
#93554=CARTESIAN_POINT('Ctrl Pts',(-20.2429296609173,-0.994090667850735,
4.24929682922339));
#93555=CARTESIAN_POINT('Ctrl Pts',(-20.0451116674801,-4.10444589668216,
1.48265426852147));
#93556=CARTESIAN_POINT('Ctrl Pts',(-19.847293674043,-3.48020632860252,-2.63304077239811));
#93557=CARTESIAN_POINT('Ctrl Pts',(-19.6494756806059,0.310638616705305,
-4.35295801134899));
#93558=CARTESIAN_POINT('Ctrl Pts',(-19.4516576871688,3.81883655170536,-2.1121617338914));
#93559=CARTESIAN_POINT('Ctrl Pts',(-19.2538396937317,3.85231281287818,2.05046965119956));
#93560=CARTESIAN_POINT('Ctrl Pts',(-19.0560217002946,0.380607680704291,
4.34739894559319));
#93561=CARTESIAN_POINT('Ctrl Pts',(-18.8582037068575,-3.43740862228359,
2.68867286262318));
#93562=CARTESIAN_POINT('Ctrl Pts',(-18.6603857134204,-4.12776075846771,
-1.41645011193827));
#93563=CARTESIAN_POINT('Ctrl Pts',(-18.4625677199833,-1.06230413519704,
-4.23275911470275));
#93564=CARTESIAN_POINT('Ctrl Pts',(-18.2647497265461,2.96973253222793,-3.19772239035583));
#93565=CARTESIAN_POINT('Ctrl Pts',(-18.066931733109,4.29963888967826,0.74689036486102));
#93566=CARTESIAN_POINT('Ctrl Pts',(-17.8691137396719,1.71734627309193,4.01191495137338));
#93567=CARTESIAN_POINT('Ctrl Pts',(-17.6712957462348,-2.42754276148306,
3.6265377345241));
#93568=CARTESIAN_POINT('Ctrl Pts',(-17.4734777527977,-4.36363460527469,
-0.0585903610256284));
#93569=CARTESIAN_POINT('Ctrl Pts',(-17.2756597593606,-2.32929840525822,
-3.69040766555911));
#93570=CARTESIAN_POINT('Ctrl Pts',(-17.0778417659235,1.8244434158099,-3.96435947175124));
#93571=CARTESIAN_POINT('Ctrl Pts',(-16.8800237724864,4.31814218613394,-0.63117973595981));
#93572=CARTESIAN_POINT('Ctrl Pts',(-16.6822057790493,2.88280601566515,3.2763042097462));
#93573=CARTESIAN_POINT('Ctrl Pts',(-16.4843877856122,-1.17556688561053,
4.20271130298191));
#93574=CARTESIAN_POINT('Ctrl Pts',(-16.2865697921751,-4.1643030844093,1.30511287631955));
#93575=CARTESIAN_POINT('Ctrl Pts',(-16.088751798738,-3.36398102217285,-2.77999487071771));
#93576=CARTESIAN_POINT('Ctrl Pts',(-15.8909338053009,0.497194158500287,
-4.33561273264911));
#93577=CARTESIAN_POINT('Ctrl Pts',(-15.6931158118637,3.90597728330769,-1.94629937600571));
#93578=CARTESIAN_POINT('Ctrl Pts',(-15.4952978184266,3.76075024297067,2.21393256644188));
#93579=CARTESIAN_POINT('Ctrl Pts',(-15.2974798249895,0.193653687619838,
4.35972912553373));
#93580=CARTESIAN_POINT('Ctrl Pts',(-15.0996618315524,-3.54964644609277,
2.53865119827378));
#93581=CARTESIAN_POINT('Ctrl Pts',(-14.9018438381153,-4.06315832527685,
-1.59232038939699));
#93582=CARTESIAN_POINT('Ctrl Pts',(-14.7040258446782,-0.879642561126436,
-4.27445537623342));
#93583=CARTESIAN_POINT('Ctrl Pts',(-14.5062078512411,3.10425128440637,-3.06730561927196));
#93584=CARTESIAN_POINT('Ctrl Pts',(-14.308389857804,4.26361753550314,0.930755236195858));
#93585=CARTESIAN_POINT('Ctrl Pts',(-14.1105718643669,1.5435602870771,4.08193109188707));
#93586=CARTESIAN_POINT('Ctrl Pts',(-13.9127538709298,-2.58096722650616,
3.51899814925455));
#93587=CARTESIAN_POINT('Ctrl Pts',(-13.7149358774927,-4.35709814338938,
-0.245836465213632));
#93588=CARTESIAN_POINT('Ctrl Pts',(-13.5171178840556,-2.16874847859741,
-3.78698690720437));
#93589=CARTESIAN_POINT('Ctrl Pts',(-13.3192998906185,1.99292401413727,-3.88239535243784));
#93590=CARTESIAN_POINT('Ctrl Pts',(-13.1214818971814,4.34125462317152,-0.445250598593546));
#93591=CARTESIAN_POINT('Ctrl Pts',(-12.9236639037442,2.73952051314873,3.39702327881237));
#93592=CARTESIAN_POINT('Ctrl Pts',(-12.7258459103071,-1.3548762636439,4.14837921470184));
#93593=CARTESIAN_POINT('Ctrl Pts',(-12.52802791687,-4.21648450526471,1.12516586138155));
#93594=CARTESIAN_POINT('Ctrl Pts',(-12.3302099234329,-3.24155512621748,
-2.9218248000948));
#93595=CARTESIAN_POINT('Ctrl Pts',(-12.1323919299958,0.682833257285865,
-4.3102759240564));
#93596=CARTESIAN_POINT('Ctrl Pts',(-11.9345739365587,3.98591840181145,-1.77684954142345));
#93597=CARTESIAN_POINT('Ctrl Pts',(-11.7367559431216,3.66225574674975,2.37331469555857));
#93598=CARTESIAN_POINT('Ctrl Pts',(-11.5389379496845,0.00634274631863393,
4.36402332353129));
#93599=CARTESIAN_POINT('Ctrl Pts',(-11.3411199562474,-3.65534145636389,
2.38395021679216));
#93600=CARTESIAN_POINT('Ctrl Pts',(-11.1433019628103,-3.99106655823213,
-1.76525565471889));
#93601=CARTESIAN_POINT('Ctrl Pts',(-10.9454839693732,-0.695359603815275,
-4.30827283492326));
#93602=CARTESIAN_POINT('Ctrl Pts',(-10.7476659759361,3.23304818860991,-2.93123509955822));
#93603=CARTESIAN_POINT('Ctrl Pts',(-10.5498479824989,4.21973735511645,1.11290451189252));
#93604=CARTESIAN_POINT('Ctrl Pts',(-10.3520299890619,1.36692916499126,4.14442329602711));
#93605=CARTESIAN_POINT('Ctrl Pts',(-10.1542119956247,-2.72963437623965,
3.40497224229606));
#93606=CARTESIAN_POINT('Ctrl Pts',(-9.95639400218764,-4.34253054906534,
-0.432629436342625));
#93607=CARTESIAN_POINT('Ctrl Pts',(-9.75857600875052,-2.00420105046087,
-3.87658586233912));
#93608=CARTESIAN_POINT('Ctrl Pts',(-9.56075801531341,2.1577311958532,-3.79327508693977));
#93609=CARTESIAN_POINT('Ctrl Pts',(-9.36294002187631,4.35636513101642,-0.25850076212705));
#93610=CARTESIAN_POINT('Ctrl Pts',(-9.16512202843919,2.59118544522533,3.51148085388605));
#93611=CARTESIAN_POINT('Ctrl Pts',(-8.9673040350021,-1.53168829359069,4.08640071089866));
#93612=CARTESIAN_POINT('Ctrl Pts',(-8.76948604156497,-4.26089397690688,
0.943144907378862));
#93613=CARTESIAN_POINT('Ctrl Pts',(-8.57166804812789,-3.11315429977641,
-3.05826913539988));
#93614=CARTESIAN_POINT('Ctrl Pts',(-8.37385005469076,0.867213737572975,
-4.2769942871274));
#93615=CARTESIAN_POINT('Ctrl Pts',(-8.17603206125366,4.05851255737768,-1.60412456510211));
#93616=CARTESIAN_POINT('Ctrl Pts',(-7.97821406781655,3.55701087219007,2.52832226068538));
#93617=CARTESIAN_POINT('Ctrl Pts',(-7.78039607437944,-0.180979886120416,
4.3602736243927));
#93618=CARTESIAN_POINT('Ctrl Pts',(-7.58257808094234,-3.75429883292162,
2.22485506761286));
#93619=CARTESIAN_POINT('Ctrl Pts',(-7.38476008750524,-3.91161833901473,
-1.93493714849773));
#93620=CARTESIAN_POINT('Ctrl Pts',(-7.18694209406812,-0.509794939073633,
-4.33414915742924));
#93621=CARTESIAN_POINT('Ctrl Pts',(-6.98912410063102,3.35588584256953,-2.78976164043119));
#93622=CARTESIAN_POINT('Ctrl Pts',(-6.7913061071939,4.168079229763,1.29300244901041));
#93623=CARTESIAN_POINT('Ctrl Pts',(-6.59348811375681,1.18777847856196,4.1992763763046));
#93624=CARTESIAN_POINT('Ctrl Pts',(-6.39567012031969,-2.87327018300228,
3.28467018959145));
#93625=CARTESIAN_POINT('Ctrl Pts',(-6.19785212688259,-4.31995867369443,
-0.618624972093756));
#93626=CARTESIAN_POINT('Ctrl Pts',(-6.00003413344547,-1.83595941960225,
-3.95903937947152));
#93627=CARTESIAN_POINT('Ctrl Pts',(-5.80221614000837,2.31856118358479,-3.69716294445239));
#93628=CARTESIAN_POINT('Ctrl Pts',(-5.60439814657126,4.36344585732357,-0.0712744492398178));
#93629=CARTESIAN_POINT('Ctrl Pts',(-5.40658015313416,2.43807422788913,3.61946596307714));
#93630=CARTESIAN_POINT('Ctrl Pts',(-5.20876215969704,-1.70567707104362,
4.01689003275298));
#93631=CARTESIAN_POINT('Ctrl Pts',(-5.01094416625994,-4.29744964101308,
0.7593855196462));
#93632=CARTESIAN_POINT('Ctrl Pts',(-4.81312617282283,-2.9790152178701,-3.18907637631703));
#93633=CARTESIAN_POINT('Ctrl Pts',(-4.61530817938572,1.04999574917882,-4.23582917153099));
#93634=CARTESIAN_POINT('Ctrl Pts',(-4.41749018594862,4.12362593199937,-1.42844281123723));
#93635=CARTESIAN_POINT('Ctrl Pts',(-4.21967219251151,3.44520962950086,2.67866953273136));
#93636=CARTESIAN_POINT('Ctrl Pts',(-4.0218541990744,-0.367968968861021,
4.34848696753938));
#93637=CARTESIAN_POINT('Ctrl Pts',(-3.8240362056373,-3.84633610223394,2.06165894627568));
#93638=CARTESIAN_POINT('Ctrl Pts',(-3.62621821220018,-3.82496024749434,
-2.10105200661351));
#93639=CARTESIAN_POINT('Ctrl Pts',(-3.42840021876308,-0.323290339886936,
-4.35203684336192));
#93640=CARTESIAN_POINT('Ctrl Pts',(-3.23058222532597,3.47253732028477,-2.64314563540684));
#93641=CARTESIAN_POINT('Ctrl Pts',(-3.03276423188886,4.10873934992313,1.47071636850529));
#93642=CARTESIAN_POINT('Ctrl Pts',(-2.83494623845175,1.00643658116675,4.24639059914366));
#93643=CARTESIAN_POINT('Ctrl Pts',(-2.63712824501465,-3.0116063268114,3.15831110600399));
#93644=CARTESIAN_POINT('Ctrl Pts',(-2.43931025157754,-4.28943095087281,
-0.803475205212229));
#93645=CARTESIAN_POINT('Ctrl Pts',(-2.24149225814043,-1.6643206191126,-4.03420511823695));
#93646=CARTESIAN_POINT('Ctrl Pts',(-2.04367426470332,2.47509249542551,-3.59421762261588));
#93647=CARTESIAN_POINT('Ctrl Pts',(-1.84585627126622,4.36253168746809,0.11604789406065));
#93648=CARTESIAN_POINT('Ctrl Pts',(-1.64803827782911,2.28037729210179,3.72084724282401));
#93649=CARTESIAN_POINT('Ctrl Pts',(-1.45022028439201,-1.87634613733157,
3.93984571205739));
#93650=CARTESIAN_POINT('Ctrl Pts',(-1.25240229095489,-4.32642069300014,
0.574474595543115));
#93651=CARTESIAN_POINT('Ctrl Pts',(-1.05458429751779,-2.83874028897046,
-3.31448106439046));
#93652=CARTESIAN_POINT('Ctrl Pts',(-0.856766304080679,1.22960426661822,
-4.18594181834751));
#93653=CARTESIAN_POINT('Ctrl Pts',(-0.658948310643567,4.18353983685536,
-1.2519143701353));
#93654=CARTESIAN_POINT('Ctrl Pts',(-0.461130317206463,3.32218428771488,
2.82781316122078));
#93655=CARTESIAN_POINT('Ctrl Pts',(-0.329251654915058,0.745725457142593,
3.82191791901945));
#93656=CARTESIAN_POINT('Ctrl Pts',(-0.263312323769356,-0.469464555276475,
3.66631519292041));
#93657=CARTESIAN_POINT('Ctrl Pts',(-29.4036876762306,2.00907721869555,-2.81633609132833));
#93658=CARTESIAN_POINT('Ctrl Pts',(-29.3377483450849,2.94254401293249,-2.1504330137501));
#93659=CARTESIAN_POINT('Ctrl Pts',(-29.2058696827936,4.07972503304445,0.170672396845149));
#93660=CARTESIAN_POINT('Ctrl Pts',(-29.0080516893564,2.0768775789713,3.52012468472226));
#93661=CARTESIAN_POINT('Ctrl Pts',(-28.8102336959193,-1.81750093524801,
3.65656959796921));
#93662=CARTESIAN_POINT('Ctrl Pts',(-28.6124157024822,-4.05720694803216,
0.470971330865179));
#93663=CARTESIAN_POINT('Ctrl Pts',(-28.4145977090451,-2.60579536053973,
-3.14576209163));
#93664=CARTESIAN_POINT('Ctrl Pts',(-28.216779715608,1.21686226448183,-3.89884107013144));
#93665=CARTESIAN_POINT('Ctrl Pts',(-28.0189617221709,3.93217388234734,-1.10511121836174));
#93666=CARTESIAN_POINT('Ctrl Pts',(-27.8211437287338,3.06970983859651,2.69451822910493));
#93667=CARTESIAN_POINT('Ctrl Pts',(-27.6233257352967,-0.585889714186953,
4.04223901204422));
#93668=CARTESIAN_POINT('Ctrl Pts',(-27.4255077418596,-3.70837476329012,
1.712067292229));
#93669=CARTESIAN_POINT('Ctrl Pts',(-27.2276897484225,-3.45665627610379,
-2.1759502299336));
#93670=CARTESIAN_POINT('Ctrl Pts',(-27.0298717549854,-0.0597551248823223,
-4.08406461081147));
#93671=CARTESIAN_POINT('Ctrl Pts',(-26.8320537615482,3.39151388417357,-2.27614329333393));
#93672=CARTESIAN_POINT('Ctrl Pts',(-26.6342357681111,3.75687932664852,1.60282583734741));
#93673=CARTESIAN_POINT('Ctrl Pts',(-26.436417774674,0.703896615223974,4.02339564497843));
#93674=CARTESIAN_POINT('Ctrl Pts',(-26.2385997812369,-2.98955428625109,
2.78311952613708));
#93675=CARTESIAN_POINT('Ctrl Pts',(-26.0407817877998,-3.96283946333539,
-0.989490639802492));
#93676=CARTESIAN_POINT('Ctrl Pts',(-25.8429637943627,-1.33037603261715,
-3.86177248390795));
#93677=CARTESIAN_POINT('Ctrl Pts',(-25.6451458009256,2.51258335935589,-3.22026596493412));
#93678=CARTESIAN_POINT('Ctrl Pts',(-25.4473278074885,4.0693679892133,0.351328913097125));
#93679=CARTESIAN_POINT('Ctrl Pts',(-25.2495098140513,1.92347484866417,3.60325300236361));
#93680=CARTESIAN_POINT('Ctrl Pts',(-25.0516918206143,-1.97256905769413,
3.57661280235394));
#93681=CARTESIAN_POINT('Ctrl Pts',(-24.8538738271771,-4.07379185838536,
0.2956479048122));
#93682=CARTESIAN_POINT('Ctrl Pts',(-24.65605583374,-2.46831166679449,-3.25432409096666));
#93683=CARTESIAN_POINT('Ctrl Pts',(-24.458237840303,1.38306093887013,-3.84321873325179));
#93684=CARTESIAN_POINT('Ctrl Pts',(-24.2604198468658,3.97600005223996,-0.935206592364037));
#93685=CARTESIAN_POINT('Ctrl Pts',(-24.0626018534288,2.9512159740629,2.82374079171459));
#93686=CARTESIAN_POINT('Ctrl Pts',(-23.8647838599916,-0.758850380473512,
4.01339430993215));
#93687=CARTESIAN_POINT('Ctrl Pts',(-23.6669658665545,-3.77844626626852,
1.55129997060155));
#93688=CARTESIAN_POINT('Ctrl Pts',(-23.4691478731174,-3.36007120012553,
-2.32230689527902));
#93689=CARTESIAN_POINT('Ctrl Pts',(-23.2713298796803,0.115599475953315,
-4.08286964612867));
#93690=CARTESIAN_POINT('Ctrl Pts',(-23.0735118862432,3.48608733022402,-2.12846961735411));
#93691=CARTESIAN_POINT('Ctrl Pts',(-22.8756938928061,3.68461874194987,1.76260390117095));
#93692=CARTESIAN_POINT('Ctrl Pts',(-22.677875899369,0.530551939773822,4.0499015327781));
#93693=CARTESIAN_POINT('Ctrl Pts',(-22.4800579059319,-3.10625883409863,
2.65223374564798));
#93694=CARTESIAN_POINT('Ctrl Pts',(-22.2822399124948,-3.91671536389035,
-1.158675340308));
#93695=CARTESIAN_POINT('Ctrl Pts',(-22.0844219190576,-1.16339125503638,
-3.91531717408475));
#93696=CARTESIAN_POINT('Ctrl Pts',(-21.8866039256206,2.64849107024913,-3.10945056831344));
#93697=CARTESIAN_POINT('Ctrl Pts',(-21.6887859321834,4.05053752009681,0.52567440898612));
#93698=CARTESIAN_POINT('Ctrl Pts',(-21.4909679387464,1.76703987263422,3.68249343169766));
#93699=CARTESIAN_POINT('Ctrl Pts',(-21.2931499453092,-2.12426990840011,
3.4886480393185));
#93700=CARTESIAN_POINT('Ctrl Pts',(-21.0953319518721,-4.08272747336339,
0.120516240478409));
#93701=CARTESIAN_POINT('Ctrl Pts',(-20.897513958435,-2.32635162036054,-3.35727209567843));
#93702=CARTESIAN_POINT('Ctrl Pts',(-20.6996959649979,1.54674860321008,-3.7803116993765));
#93703=CARTESIAN_POINT('Ctrl Pts',(-20.5018779715608,4.01247754425332,-0.763683012013472));
#93704=CARTESIAN_POINT('Ctrl Pts',(-20.3040599781237,2.82729278422816,2.94781330789901));
#93705=CARTESIAN_POINT('Ctrl Pts',(-20.1062419846866,-0.930417765418907,
3.97712340363837));
#93706=CARTESIAN_POINT('Ctrl Pts',(-19.9084239912495,-3.84155037661736,
1.38768818179236));
#93707=CARTESIAN_POINT('Ctrl Pts',(-19.7106059978124,-3.2572942289619,-2.46439081558641));
#93708=CARTESIAN_POINT('Ctrl Pts',(-19.5127880043753,0.290741777339739,
-4.0741449415656));
#93709=CARTESIAN_POINT('Ctrl Pts',(-19.3149700109381,3.5742347110246,-1.97687481052344));
#93710=CARTESIAN_POINT('Ctrl Pts',(-19.117152017501,3.60556677068707,1.91913419230974));
#93711=CARTESIAN_POINT('Ctrl Pts',(-18.9193340240639,0.356229224591542,
4.06894194177332));
#93712=CARTESIAN_POINT('Ctrl Pts',(-18.7215160306268,-3.21723777579712,
2.51645959235574));
#93713=CARTESIAN_POINT('Ctrl Pts',(-18.5236980371897,-3.86337188878432,
-1.32572449435251));
#93714=CARTESIAN_POINT('Ctrl Pts',(-18.3258800437526,-0.994262064447525,
-3.96164495294261));
#93715=CARTESIAN_POINT('Ctrl Pts',(-18.1280620503155,2.77951699566927,-2.99290378341184));
#93716=CARTESIAN_POINT('Ctrl Pts',(-17.9302440568784,4.02424098446856,0.69905098876881));
#93717=CARTESIAN_POINT('Ctrl Pts',(-17.7324260634413,1.60734783409173,3.75494616821811));
#93718=CARTESIAN_POINT('Ctrl Pts',(-17.5346080700042,-2.27205524067654,
3.39425290296547));
#93719=CARTESIAN_POINT('Ctrl Pts',(-17.3367900765671,-4.08413768466629,
-0.0548375661733324));
#93720=CARTESIAN_POINT('Ctrl Pts',(-17.13897208313,-2.18010357334888,-3.45403187527947));
#93721=CARTESIAN_POINT('Ctrl Pts',(-16.9411540896928,1.70758525451319,-3.71043668380749));
#93722=CARTESIAN_POINT('Ctrl Pts',(-16.7433360962558,4.04155911881782,-0.590751788042732));
#93723=CARTESIAN_POINT('Ctrl Pts',(-16.5455181028186,2.6981582444893,3.06645232698464));
#93724=CARTESIAN_POINT('Ctrl Pts',(-16.3477001093816,-1.10027017673849,
3.93352174573308));
#93725=CARTESIAN_POINT('Ctrl Pts',(-16.1498821159444,-3.89757362746404,
1.22151856493134));
#93726=CARTESIAN_POINT('Ctrl Pts',(-15.9520641225073,-3.14851331652539,
-2.60193229766599));
#93727=CARTESIAN_POINT('Ctrl Pts',(-15.7542461290702,0.465348174861481,
-4.05791065230967));
#93728=CARTESIAN_POINT('Ctrl Pts',(-15.5564281356331,3.65579395647019,-1.82163616943977));
#93729=CARTESIAN_POINT('Ctrl Pts',(-15.358610142196,3.51986891188557,2.07212707841885));
#93730=CARTESIAN_POINT('Ctrl Pts',(-15.1607921487589,0.181249897144626,
4.08048235638389));
#93731=CARTESIAN_POINT('Ctrl Pts',(-14.9629741553218,-3.3222866094712,2.37604702615573));
#93732=CARTESIAN_POINT('Ctrl Pts',(-14.7651561618847,-3.80290733210558,
-1.49033003371495));
#93733=CARTESIAN_POINT('Ctrl Pts',(-14.5673381684476,-0.823300220552425,
-4.00067051040366));
#93734=CARTESIAN_POINT('Ctrl Pts',(-14.3695201750105,2.90541963298041,-2.87084038954923));
#93735=CARTESIAN_POINT('Ctrl Pts',(-14.1717021815733,3.99052684858251,0.871139057049595));
#93736=CARTESIAN_POINT('Ctrl Pts',(-13.9738841881363,1.44469308438099,3.8204776766678));
#93737=CARTESIAN_POINT('Ctrl Pts',(-13.7760661946991,-2.41565265339143,
3.29360137905881));
#93738=CARTESIAN_POINT('Ctrl Pts',(-13.5782482012621,-4.07801989233833,
-0.230090294597647));
#93739=CARTESIAN_POINT('Ctrl Pts',(-13.3804302078249,-2.02983709481441,
-3.54442508095327));
#93740=CARTESIAN_POINT('Ctrl Pts',(-13.1826122143878,1.86527443406369,-3.63372248136861));
#93741=CARTESIAN_POINT('Ctrl Pts',(-12.9847942209507,4.063191171826,-0.416731672866926));
#93742=CARTESIAN_POINT('Ctrl Pts',(-12.7869762275136,2.56405037950302,3.17943917025402));
#93743=CARTESIAN_POINT('Ctrl Pts',(-12.5891582340765,-1.26809453745718,
3.88266970395969));
#93744=CARTESIAN_POINT('Ctrl Pts',(-12.3913402406394,-3.94641275507968,
1.05309740884666));
#93745=CARTESIAN_POINT('Ctrl Pts',(-12.1935222472023,-3.03392897102452,
-2.73467782101535));
#93746=CARTESIAN_POINT('Ctrl Pts',(-11.9957042537652,0.639096828834754,
-4.03419670186625));
#93747=CARTESIAN_POINT('Ctrl Pts',(-11.797886260328,3.73061473414047,-1.66303983457679));
#93748=CARTESIAN_POINT('Ctrl Pts',(-11.600068266891,3.42768312637964,2.22130055848087));
#93749=CARTESIAN_POINT('Ctrl Pts',(-11.4022502734538,0.00593648451520102,
4.08450150497301));
#93750=CARTESIAN_POINT('Ctrl Pts',(-11.2044322800167,-3.42121170599686,
2.23125485965302));
#93751=CARTESIAN_POINT('Ctrl Pts',(-11.0066142865796,-3.73543314391723,
-1.65218855258708));
#93752=CARTESIAN_POINT('Ctrl Pts',(-10.8087962931425,-0.650820845288858,
-4.03232191340333));
#93753=CARTESIAN_POINT('Ctrl Pts',(-10.6109782997054,3.02596691470977,-2.74348537759124));
#93754=CARTESIAN_POINT('Ctrl Pts',(-10.4131603062683,3.9494572553332,1.04162141600058));
#93755=CARTESIAN_POINT('Ctrl Pts',(-10.2153423128312,1.2793754335576,3.87896716742802));
#93756=CARTESIAN_POINT('Ctrl Pts',(-10.0175243193941,-2.55479746353766,
3.1868789914706));
#93757=CARTESIAN_POINT('Ctrl Pts',(-9.81970632595699,-4.06438537287563,
-0.404918913771338));
#93758=CARTESIAN_POINT('Ctrl Pts',(-9.62188833251988,-1.875829160384,-3.62828509726404));
#93759=CARTESIAN_POINT('Ctrl Pts',(-9.42407033908277,2.01952548449217,-3.55031049395147));
#93760=CARTESIAN_POINT('Ctrl Pts',(-9.22625234564567,4.0773338304366,-0.241943425520061));
#93761=CARTESIAN_POINT('Ctrl Pts',(-9.02843435220854,2.42521638086088,3.2865655770088));
#93762=CARTESIAN_POINT('Ctrl Pts',(-8.83061635877145,-1.43358150873913,
3.82466101030881));
#93763=CARTESIAN_POINT('Ctrl Pts',(-8.63279836533434,-3.98797773773671,
0.88273515240505));
#93764=CARTESIAN_POINT('Ctrl Pts',(-8.43498037189723,-2.91375239772107,
-2.8623827051514));
#93765=CARTESIAN_POINT('Ctrl Pts',(-8.23716237846012,0.811667480590791,
-4.00304680049164));
#93766=CARTESIAN_POINT('Ctrl Pts',(-8.03934438502302,3.79855913216046,-1.5013781353996));
#93767=CARTESIAN_POINT('Ctrl Pts',(-7.84152639158591,3.32917933374137,2.36637967151602));
#93768=CARTESIAN_POINT('Ctrl Pts',(-7.6437083981488,-0.169387870418285,
4.08099197932676));
#93769=CARTESIAN_POINT('Ctrl Pts',(-7.4458904047117,-3.51383072370439,2.08234997806065));
#93770=CARTESIAN_POINT('Ctrl Pts',(-7.24807241127459,-3.66107369464226,
-1.81100170854999));
#93771=CARTESIAN_POINT('Ctrl Pts',(-7.05025441783748,-0.477141857754542,
-4.05654082113668));
#93772=CARTESIAN_POINT('Ctrl Pts',(-6.85243642440037,3.14093664453684,-2.61107349207216));
#93773=CARTESIAN_POINT('Ctrl Pts',(-6.65461843096327,3.90110790540821,1.21018382748773));
#93774=CARTESIAN_POINT('Ctrl Pts',(-6.45680043752616,1.11169960002302,3.9303068309302));
#93775=CARTESIAN_POINT('Ctrl Pts',(-6.25898244408904,-2.68923319529155,
3.07428245407957));
#93776=CARTESIAN_POINT('Ctrl Pts',(-6.06116445065195,-4.04325925780071,
-0.579001174422278));
#93777=CARTESIAN_POINT('Ctrl Pts',(-5.86334645721482,-1.7183636421005,-3.70545735090477));
#93778=CARTESIAN_POINT('Ctrl Pts',(-5.66552846377773,2.17005408579278,-3.46035446907894));
#93779=CARTESIAN_POINT('Ctrl Pts',(-5.46771047034061,4.08396102628634,-0.0667092207359237));
#93780=CARTESIAN_POINT('Ctrl Pts',(-5.26989247690351,2.28191215187892,3.38763408840457));
#93781=CARTESIAN_POINT('Ctrl Pts',(-5.0720744834664,-1.59642606081174,3.75960258865307));
#93782=CARTESIAN_POINT('Ctrl Pts',(-4.87425649002929,-4.02219196025289,
0.710745811353679));
#93783=CARTESIAN_POINT('Ctrl Pts',(-4.67643849659218,-2.78820511226827,
-2.98481155870647));
#93784=CARTESIAN_POINT('Ctrl Pts',(-4.47862050315508,0.982742047827972,
-3.96451836832234));
#93785=CARTESIAN_POINT('Ctrl Pts',(-4.28080250971797,3.8595019037543,-1.33694904443022));
#93786=CARTESIAN_POINT('Ctrl Pts',(-4.08298451628086,3.22453911755379,2.50709698978266));
#93787=CARTESIAN_POINT('Ctrl Pts',(-3.88516652284376,-0.34440003997963,
4.06996027438687));
#93788=CARTESIAN_POINT('Ctrl Pts',(-3.68734852940665,-3.5999728767476,1.92960679733263));
#93789=CARTESIAN_POINT('Ctrl Pts',(-3.48953053596953,-3.579966175504,-1.96647667686965));
#93790=CARTESIAN_POINT('Ctrl Pts',(-3.29171254253244,-0.302583139895528,
-4.0732827756809));
#93791=CARTESIAN_POINT('Ctrl Pts',(-3.09389454909532,3.25011643138997,-2.47384844793777));
#93792=CARTESIAN_POINT('Ctrl Pts',(-2.89607655565822,3.8455688281526,1.37651492102646));
#93793=CARTESIAN_POINT('Ctrl Pts',(-2.69825856222111,0.941972905660164,
3.97440332167399));
#93794=CARTESIAN_POINT('Ctrl Pts',(-2.50044056878401,-2.81870871494191,
2.95601684713447));
#93795=CARTESIAN_POINT('Ctrl Pts',(-2.30262257534689,-4.01468687846993,
-0.752011490681563));
#93796=CARTESIAN_POINT('Ctrl Pts',(-2.10480458190979,-1.55771854766859,
-3.77580861861094));
#93797=CARTESIAN_POINT('Ctrl Pts',(-1.90698658847268,2.31655934742633,-3.36400293958462));
#93798=CARTESIAN_POINT('Ctrl Pts',(-1.70916859503557,4.0831054102931,0.108614863578718));
#93799=CARTESIAN_POINT('Ctrl Pts',(-1.51135060159846,2.13431592614843,3.48252175490014));
#93800=CARTESIAN_POINT('Ctrl Pts',(-1.31353260816136,-1.75616353387854,
3.68749306482585));
#93801=CARTESIAN_POINT('Ctrl Pts',(-1.11571461472425,-4.04930737570077,
0.537678691452524));
#93802=CARTESIAN_POINT('Ctrl Pts',(-0.917896621287142,-2.65691498943343,
-3.10218390050965));
#93803=CARTESIAN_POINT('Ctrl Pts',(-0.720078627850037,1.1508463876539,-3.91782637012465));
#93804=CARTESIAN_POINT('Ctrl Pts',(-0.522260634412922,3.91557823891813,
-1.17172749772961));
#93805=CARTESIAN_POINT('Ctrl Pts',(-0.324442640975819,3.10939372156906,
2.64668775955179));
#93806=CARTESIAN_POINT('Ctrl Pts',(-0.192563978684414,0.697960695024636,
3.57711871243769));
#93807=CARTESIAN_POINT('Ctrl Pts',(-0.126624647538713,-0.43939469164125,
3.43148255932585));
#93808=CARTESIAN_POINT('Ctrl Pts',(-29.267,1.871586531739,-2.6236008493506));
#93809=CARTESIAN_POINT('Ctrl Pts',(-29.2010606688543,2.74117176403474,-2.0032686790181));
#93810=CARTESIAN_POINT('Ctrl Pts',(-29.069182006563,3.80053009112415,0.158992474904673));
#93811=CARTESIAN_POINT('Ctrl Pts',(-28.8713640131257,1.93474699165479,3.27922584988832));
#93812=CARTESIAN_POINT('Ctrl Pts',(-28.6735460196887,-1.69312072237911,
3.40633319030359));
#93813=CARTESIAN_POINT('Ctrl Pts',(-28.4757280262515,-3.77955302551543,
0.438740527979693));
#93814=CARTESIAN_POINT('Ctrl Pts',(-28.2779100328145,-2.4274684197657,-2.93048266535644));
#93815=CARTESIAN_POINT('Ctrl Pts',(-28.0800920393773,1.13358660582709,-3.63202487607056));
#93816=CARTESIAN_POINT('Ctrl Pts',(-27.8822740459403,3.66307656578549,-1.02948321404113));
#93817=CARTESIAN_POINT('Ctrl Pts',(-27.6844560525031,2.85963502885877,2.51011956145336));
#93818=CARTESIAN_POINT('Ctrl Pts',(-27.4866380590661,-0.545794501053909,
3.76560941640859));
#93819=CARTESIAN_POINT('Ctrl Pts',(-27.2888200656289,-3.45459308235099,
1.59490240382455));
#93820=CARTESIAN_POINT('Ctrl Pts',(-27.0910020721918,-3.2201008856232,-2.02703963102139));
#93821=CARTESIAN_POINT('Ctrl Pts',(-26.8931840787547,-0.0556657981542161,
-3.80457269099369));
#93822=CARTESIAN_POINT('Ctrl Pts',(-26.6953660853176,3.15941649666726,-2.12037600768663));
#93823=CARTESIAN_POINT('Ctrl Pts',(-26.4975480918805,3.49977824828921,1.49313686004087));
#93824=CARTESIAN_POINT('Ctrl Pts',(-26.2997300984434,0.655725629921395,
3.7480555903611));
#93825=CARTESIAN_POINT('Ctrl Pts',(-26.1019121050063,-2.78496490129086,
2.59265745132483));
#93826=CARTESIAN_POINT('Ctrl Pts',(-25.9040941115692,-3.69164355556124,
-0.921775100281393));
#93827=CARTESIAN_POINT('Ctrl Pts',(-25.706276118132,-1.23933208819682,-3.59749306908928));
#93828=CARTESIAN_POINT('Ctrl Pts',(-25.508458124695,2.34063535810499,-2.99988788509652));
#93829=CARTESIAN_POINT('Ctrl Pts',(-25.3106401312578,3.79088182894556,0.327285808551454));
#93830=CARTESIAN_POINT('Ctrl Pts',(-25.1128221378208,1.79184233806401,3.35666530231748));
#93831=CARTESIAN_POINT('Ctrl Pts',(-24.9150041443836,-1.83757679742267,
3.3318482175997));
#93832=CARTESIAN_POINT('Ctrl Pts',(-24.7171861509465,-3.79500295175934,
0.275415315864581));
#93833=CARTESIAN_POINT('Ctrl Pts',(-24.5193681575094,-2.29939338753055,
-3.03161525196208));
#93834=CARTESIAN_POINT('Ctrl Pts',(-24.3215501640723,1.28841151633002,-3.5802090396263));
#93835=CARTESIAN_POINT('Ctrl Pts',(-24.1237321706352,3.70390350292133,-0.871205967781821));
#93836=CARTESIAN_POINT('Ctrl Pts',(-23.925914177198,2.74925026171735,2.63049881095482));
#93837=CARTESIAN_POINT('Ctrl Pts',(-23.728096183761,-0.706918648264489,
3.73873869412743));
#93838=CARTESIAN_POINT('Ctrl Pts',(-23.5302781903238,-3.51986925989793,
1.44513715284179));
#93839=CARTESIAN_POINT('Ctrl Pts',(-23.3324601968868,-3.13012558468118,
-2.16338041530871));
#93840=CARTESIAN_POINT('Ctrl Pts',(-23.1346422034496,0.107688455305257,
-3.80345950341412));
#93841=CARTESIAN_POINT('Ctrl Pts',(-22.9368242100126,3.24751783306243,-1.98280834205173));
#93842=CARTESIAN_POINT('Ctrl Pts',(-22.7390062165755,3.43246279827112,1.64198055282517));
#93843=CARTESIAN_POINT('Ctrl Pts',(-22.5411882231383,0.494243753116372,
3.77274755449071));
#93844=CARTESIAN_POINT('Ctrl Pts',(-22.3433702297012,-2.89368280317716,
2.47072880583525));
#93845=CARTESIAN_POINT('Ctrl Pts',(-22.1455522362641,-3.64867594709571,
-1.07938168896592));
#93846=CARTESIAN_POINT('Ctrl Pts',(-21.947734242827,-1.08377487127288,-3.64737344205279));
#93847=CARTESIAN_POINT('Ctrl Pts',(-21.7499162493899,2.46724225947258,-2.89665611187517));
#93848=CARTESIAN_POINT('Ctrl Pts',(-21.5520982559528,3.7733400181795,0.489700014903892));
#93849=CARTESIAN_POINT('Ctrl Pts',(-21.3542802625157,1.64611294971294,3.43048293308387));
#93850=CARTESIAN_POINT('Ctrl Pts',(-21.1564622690786,-1.97889603910867,
3.24990330068325));
#93851=CARTESIAN_POINT('Ctrl Pts',(-20.9586442756415,-3.80332706020577,
0.11226874230432));
#93852=CARTESIAN_POINT('Ctrl Pts',(-20.7608262822044,-2.16714834066106,
-3.12751803623289));
#93853=CARTESIAN_POINT('Ctrl Pts',(-20.5630082887673,1.44089725711671,-3.52160703256702));
#93854=CARTESIAN_POINT('Ctrl Pts',(-20.3651902953302,3.73788466707397,-0.711420559897795));
#93855=CARTESIAN_POINT('Ctrl Pts',(-20.1673723018931,2.63380772376682,2.7460804561444));
#93856=CARTESIAN_POINT('Ctrl Pts',(-19.9695543084559,-0.866744862987072,
3.70494997805335));
#93857=CARTESIAN_POINT('Ctrl Pts',(-19.7717363150188,-3.57865485655257,
1.29272209506325));
#93858=CARTESIAN_POINT('Ctrl Pts',(-19.5739183215817,-3.03438212932128,
-2.29574085877471));
#93859=CARTESIAN_POINT('Ctrl Pts',(-19.3761003281446,0.270844937974172,
-3.7953318717822));
#93860=CARTESIAN_POINT('Ctrl Pts',(-19.1782823347075,3.32963287034385,-1.84158788715549));
#93861=CARTESIAN_POINT('Ctrl Pts',(-18.9804643412704,3.35882072849595,1.78779873341992));
#93862=CARTESIAN_POINT('Ctrl Pts',(-18.7826463478333,0.331850768478793,
3.79048493795346));
#93863=CARTESIAN_POINT('Ctrl Pts',(-18.5848283543962,-2.99706692931064,
2.34424632208829));
#93864=CARTESIAN_POINT('Ctrl Pts',(-18.3870103609591,-3.59898301910093,
-1.23499887676674));
#93865=CARTESIAN_POINT('Ctrl Pts',(-18.189192367522,-0.926219993698007,
-3.69053079118249));
#93866=CARTESIAN_POINT('Ctrl Pts',(-17.9913743740849,2.5893014591106,-2.78808517646783));
#93867=CARTESIAN_POINT('Ctrl Pts',(-17.7935563806477,3.74884307925887,0.651211612676593));
#93868=CARTESIAN_POINT('Ctrl Pts',(-17.5957383872107,1.49734939509152,3.49797738506285));
#93869=CARTESIAN_POINT('Ctrl Pts',(-17.3979203937735,-2.11656771987002,
3.16196807140684));
#93870=CARTESIAN_POINT('Ctrl Pts',(-17.2001024003364,-3.80464076405789,
-0.0510847713210306));
#93871=CARTESIAN_POINT('Ctrl Pts',(-17.0022844068993,-2.03090874143955,
-3.21765608499983));
#93872=CARTESIAN_POINT('Ctrl Pts',(-16.8044664134622,1.59072709321647,-3.45651389586373));
#93873=CARTESIAN_POINT('Ctrl Pts',(-16.6066484200251,3.7649760515017,-0.55032384012566));
#93874=CARTESIAN_POINT('Ctrl Pts',(-16.408830426588,2.51351047331346,2.85660044422309));
#93875=CARTESIAN_POINT('Ctrl Pts',(-16.2110124331509,-1.02497346786645,
3.66433218848425));
#93876=CARTESIAN_POINT('Ctrl Pts',(-16.0131944397138,-3.63084417051879,
1.13792425354314));
#93877=CARTESIAN_POINT('Ctrl Pts',(-15.8153764462767,-2.93304561087793,
-2.42386972461428));
#93878=CARTESIAN_POINT('Ctrl Pts',(-15.6175584528396,0.433502191222674,
-3.78020857197022));
#93879=CARTESIAN_POINT('Ctrl Pts',(-15.4197404594025,3.40561062963269,-1.69697296287383));
#93880=CARTESIAN_POINT('Ctrl Pts',(-15.2219224659654,3.27898758080047,1.93032159039582));
#93881=CARTESIAN_POINT('Ctrl Pts',(-15.0241044725282,0.168846106669414,
3.80123558723405));
#93882=CARTESIAN_POINT('Ctrl Pts',(-14.8262864790911,-3.09492677284964,
2.21344285403769));
#93883=CARTESIAN_POINT('Ctrl Pts',(-14.628468485654,-3.54265633893431,-1.38833967803291));
#93884=CARTESIAN_POINT('Ctrl Pts',(-14.4306504922169,-0.766957879978414,
-3.7268856445739));
#93885=CARTESIAN_POINT('Ctrl Pts',(-14.2328324987798,2.70658798155444,-2.6743751598265));
#93886=CARTESIAN_POINT('Ctrl Pts',(-14.0350145053427,3.71743616166189,0.811522877903334));
#93887=CARTESIAN_POINT('Ctrl Pts',(-13.8371965119056,1.34582588168488,3.55902426144851));
#93888=CARTESIAN_POINT('Ctrl Pts',(-13.6393785184685,-2.2503380802767,3.06820460886307));
#93889=CARTESIAN_POINT('Ctrl Pts',(-13.4415605250314,-3.79894164128729,
-0.214344123981669));
#93890=CARTESIAN_POINT('Ctrl Pts',(-13.2437425315943,-1.8909257110314,-3.30186325470216));
#93891=CARTESIAN_POINT('Ctrl Pts',(-13.0459245381572,1.7376248539901,-3.38504961029937));
#93892=CARTESIAN_POINT('Ctrl Pts',(-12.8481065447201,3.78512772048049,-0.388212747140301));
#93893=CARTESIAN_POINT('Ctrl Pts',(-12.6502885512829,2.38858024585731,2.96185506169566));
#93894=CARTESIAN_POINT('Ctrl Pts',(-12.4524705578458,-1.18131281127045,
3.61696019321754));
#93895=CARTESIAN_POINT('Ctrl Pts',(-12.2546525644087,-3.67634100489465,
0.98102895631177));
#93896=CARTESIAN_POINT('Ctrl Pts',(-12.0568345709716,-2.82630281583156,
-2.54753084193589));
#93897=CARTESIAN_POINT('Ctrl Pts',(-11.8590165775345,0.595360400383641,
-3.75811747967609));
#93898=CARTESIAN_POINT('Ctrl Pts',(-11.6611985840974,3.47531106646949,-1.54923012773011));
#93899=CARTESIAN_POINT('Ctrl Pts',(-11.4633805906603,3.19311050600954,2.06928642140315));
#93900=CARTESIAN_POINT('Ctrl Pts',(-11.2655625972232,0.00553022271176743,
3.80497968641473));
#93901=CARTESIAN_POINT('Ctrl Pts',(-11.0677446037861,-3.18708195562982,
2.07855950251388));
#93902=CARTESIAN_POINT('Ctrl Pts',(-10.869926610349,-3.47979972960233,-1.53912145045528));
#93903=CARTESIAN_POINT('Ctrl Pts',(-10.6721086169119,-0.606282086762444,
-3.75637099188338));
#93904=CARTESIAN_POINT('Ctrl Pts',(-10.4742906234748,2.81888564080964,-2.55573565562428));
#93905=CARTESIAN_POINT('Ctrl Pts',(-10.2764726300377,3.67917715554996,0.970338320108655));
#93906=CARTESIAN_POINT('Ctrl Pts',(-10.0786546366006,1.19182170212393,3.61351103882891));
#93907=CARTESIAN_POINT('Ctrl Pts',(-9.88083664316345,-2.37996055083567,
2.96878574064515));
#93908=CARTESIAN_POINT('Ctrl Pts',(-9.68301864972634,-3.78624019668592,
-0.377208391200055));
#93909=CARTESIAN_POINT('Ctrl Pts',(-9.48520065628923,-1.74745727030714,
-3.37998433218895));
#93910=CARTESIAN_POINT('Ctrl Pts',(-9.28738266285213,1.88131977313113,-3.30734590096318));
#93911=CARTESIAN_POINT('Ctrl Pts',(-9.08956466941502,3.79830252985678,-0.225386088913072));
#93912=CARTESIAN_POINT('Ctrl Pts',(-8.8917466759779,2.25924731649643,3.06165030013156));
#93913=CARTESIAN_POINT('Ctrl Pts',(-8.69392868254081,-1.33547472388757,
3.56292130971895));
#93914=CARTESIAN_POINT('Ctrl Pts',(-8.49611068910369,-3.71506149856655,
0.822325397431237));
#93915=CARTESIAN_POINT('Ctrl Pts',(-8.2982926956666,-2.71435049566573,-2.66649627490293));
#93916=CARTESIAN_POINT('Ctrl Pts',(-8.10047470222948,0.756121223608606,
-3.72909931385589));
#93917=CARTESIAN_POINT('Ctrl Pts',(-7.90265670879237,3.53860570694324,-1.39863170569708));
#93918=CARTESIAN_POINT('Ctrl Pts',(-7.70483871535527,3.10134779529267,2.20443708234665));
#93919=CARTESIAN_POINT('Ctrl Pts',(-7.50702072191815,-0.15779585471615,
3.80171033426082));
#93920=CARTESIAN_POINT('Ctrl Pts',(-7.30920272848106,-3.27336261448717,
1.93984488850845));
#93921=CARTESIAN_POINT('Ctrl Pts',(-7.11138473504394,-3.41052905026979,
-1.68706626860225));
#93922=CARTESIAN_POINT('Ctrl Pts',(-6.91356674160684,-0.444488776435454,
-3.77893248484412));
#93923=CARTESIAN_POINT('Ctrl Pts',(-6.71574874816972,2.92598744650415,-2.43238534371312));
#93924=CARTESIAN_POINT('Ctrl Pts',(-6.51793075473262,3.63413658105342,1.12736520596504));
#93925=CARTESIAN_POINT('Ctrl Pts',(-6.32011276129551,1.03562072148409,3.66133728555581));
#93926=CARTESIAN_POINT('Ctrl Pts',(-6.12229476785841,-2.50519620758082,
2.86389471856769));
#93927=CARTESIAN_POINT('Ctrl Pts',(-5.92447677442129,-3.766559841907,-0.539377376750802));
#93928=CARTESIAN_POINT('Ctrl Pts',(-5.72665878098419,-1.60076786459875,
-3.45187532233801));
#93929=CARTESIAN_POINT('Ctrl Pts',(-5.52884078754708,2.02154698800078,-3.22354599370549));
#93930=CARTESIAN_POINT('Ctrl Pts',(-5.33102279410997,3.80447619524911,-0.0621439922320252));
#93931=CARTESIAN_POINT('Ctrl Pts',(-5.13320480067286,2.12575007586871,3.15580221373199));
#93932=CARTESIAN_POINT('Ctrl Pts',(-4.93538680723576,-1.48717505057987,
3.50231514455317));
#93933=CARTESIAN_POINT('Ctrl Pts',(-4.73756881379864,-3.7469342794927,0.662106103061155));
#93934=CARTESIAN_POINT('Ctrl Pts',(-4.53975082036155,-2.59739500666645,
-2.78054674109591));
#93935=CARTESIAN_POINT('Ctrl Pts',(-4.34193282692443,0.91548834647712,-3.69320756511369));
#93936=CARTESIAN_POINT('Ctrl Pts',(-4.14411483348733,3.59537787550923,-1.24545527762321));
#93937=CARTESIAN_POINT('Ctrl Pts',(-3.94629684005022,3.00386860560673,2.33552444683395));
#93938=CARTESIAN_POINT('Ctrl Pts',(-3.74847884661311,-0.320831111098236,
3.79143358123437));
#93939=CARTESIAN_POINT('Ctrl Pts',(-3.55066085317601,-3.35360965126126,
1.79755464838957));
#93940=CARTESIAN_POINT('Ctrl Pts',(-3.35284285973889,-3.33497210351366,
-1.8319013471258));
#93941=CARTESIAN_POINT('Ctrl Pts',(-3.15502486630179,-0.281875939904123,
-3.79452870799989));
#93942=CARTESIAN_POINT('Ctrl Pts',(-2.95720687286468,3.02769554249517,-2.30455126046869));
#93943=CARTESIAN_POINT('Ctrl Pts',(-2.75938887942757,3.58239830638208,1.28231347354763));
#93944=CARTESIAN_POINT('Ctrl Pts',(-2.56157088599047,0.877509230153572,
3.70241604420433));
#93945=CARTESIAN_POINT('Ctrl Pts',(-2.36375289255336,-2.62581110307242,
2.75372258826496));
#93946=CARTESIAN_POINT('Ctrl Pts',(-2.16593489911625,-3.73994280606706,
-0.70054777615089));
#93947=CARTESIAN_POINT('Ctrl Pts',(-1.96811690567914,-1.45111647622458,
-3.51741211898495));
#93948=CARTESIAN_POINT('Ctrl Pts',(-1.77029891224204,2.15802619942714,-3.13378825655336));
#93949=CARTESIAN_POINT('Ctrl Pts',(-1.57248091880493,3.80367913311811,0.10118183309678));
#93950=CARTESIAN_POINT('Ctrl Pts',(-1.37466292536782,1.98825456019507,3.24419626697628));
#93951=CARTESIAN_POINT('Ctrl Pts',(-1.17684493193072,-1.63598093042552,
3.4351404175943));
#93952=CARTESIAN_POINT('Ctrl Pts',(-0.979026938493603,-3.77219405840141,
0.500882787361939));
#93953=CARTESIAN_POINT('Ctrl Pts',(-0.781208945056499,-2.47508968989639,
-2.88988673662884));
#93954=CARTESIAN_POINT('Ctrl Pts',(-0.583390951619393,1.07208850868958,
-3.64971092190177));
#93955=CARTESIAN_POINT('Ctrl Pts',(-0.385572958182278,3.64761664098089,
-1.09154062532392));
#93956=CARTESIAN_POINT('Ctrl Pts',(-0.187754964745176,2.89660315542323,
2.4655623578828));
#93957=CARTESIAN_POINT('Ctrl Pts',(-0.0558763024537703,0.650195932906673,
3.33231950585592));
#93958=CARTESIAN_POINT('Ctrl Pts',(0.0100630286919312,-0.409324828006024,
3.19664992573129));
#93959=CARTESIAN_POINT('Ctrl Pts',(-0.400000000000005,-0.499534418911589,
3.90114782651499));
#93960=CARTESIAN_POINT('Ctrl Pts',(-0.465939331145705,0.793490219260627,
4.06671712560119));
#93961=CARTESIAN_POINT('Ctrl Pts',(-0.531878662291405,2.16423253656064,
3.53782784424547));
#93962=CARTESIAN_POINT('Ctrl Pts',(-0.597817993437104,3.00235812536596,
2.54987656932921));
#93963=CARTESIAN_POINT('Ctrl Pts',(-0.663757324582806,3.84048371417132,
1.56192529441289));
#93964=CARTESIAN_POINT('Ctrl Pts',(-0.729696655728509,4.14599257448196,
0.114912025935935));
#93965=CARTESIAN_POINT('Ctrl Pts',(-0.795635986874212,3.7748904564356,-1.12892061230742));
#93966=CARTESIAN_POINT('Ctrl Pts',(-0.861575318019917,3.40378833838922,
-2.37275325055082));
#93967=CARTESIAN_POINT('Ctrl Pts',(-0.92751464916562,2.3560752419859,-3.41340525856059));
#93968=CARTESIAN_POINT('Ctrl Pts',(-0.993453980311325,1.11073073810251,
-3.77918475618231));
#93969=CARTESIAN_POINT('Ctrl Pts',(-1.05939331145703,-0.134613765780807,
-4.144964253804));
#93970=CARTESIAN_POINT('Ctrl Pts',(-1.12533264260273,-1.57758967714414,
-3.83587124103763));
#93971=CARTESIAN_POINT('Ctrl Pts',(-1.19127197374843,-2.56290570312447,
-2.99164994667031));
#93972=CARTESIAN_POINT('Ctrl Pts',(-1.24846014182062,-3.41745514302525,
-2.25946979813762));
#93973=CARTESIAN_POINT('Ctrl Pts',(-1.30564830989282,-3.92776077108088,
-1.12477545649334));
#93974=CARTESIAN_POINT('Ctrl Pts',(-1.36283647796502,-3.93682057842306,
0.00276514463350926));
#93975=CARTESIAN_POINT('Origin',(-0.4,0.,0.));
#93976=CARTESIAN_POINT('',(0.,-5.30639458070548E-16,4.333));
#93977=CARTESIAN_POINT('Origin',(-0.4,-5.30639458070548E-16,4.333));
#93978=CARTESIAN_POINT('Origin',(0.,0.,0.));
#93979=CARTESIAN_POINT('Origin',(-0.4,0.,0.));
#93980=CARTESIAN_POINT('Origin',(-14.6,0.,0.));
#93981=CARTESIAN_POINT('Origin',(0.,5.8,0.));
#93982=CARTESIAN_POINT('',(0.,-5.8,-7.10295143505465E-16));
#93983=CARTESIAN_POINT('Origin',(0.,0.,0.));
#93984=CARTESIAN_POINT('Origin',(4.8215647221589,0.,0.));
#93985=CARTESIAN_POINT('',(4.55911872188336,3.75277674973257,-6.5));
#93986=CARTESIAN_POINT('',(4.55911872188336,-3.75277674973257,-6.5));
#93987=CARTESIAN_POINT('Ctrl Pts',(4.55911872188336,3.75277674973257,-6.5));
#93988=CARTESIAN_POINT('Ctrl Pts',(5.74495593589618,-6.10622663543836E-15,
-6.5));
#93989=CARTESIAN_POINT('Ctrl Pts',(4.55911872188336,-3.75277674973257,-6.5));
#93990=CARTESIAN_POINT('',(4.55911872188336,7.50555349946513,0.));
#93991=CARTESIAN_POINT('Ctrl Pts',(4.55911872188336,7.50555349946513,0.));
#93992=CARTESIAN_POINT('Ctrl Pts',(5.74495593589617,5.62916512459885,-3.25000000000001));
#93993=CARTESIAN_POINT('Ctrl Pts',(4.55911872188336,3.75277674973257,-6.5));
#93994=CARTESIAN_POINT('',(4.55911872188336,3.75277674973257,6.5));
#93995=CARTESIAN_POINT('Ctrl Pts',(4.55911872188336,3.75277674973257,6.5));
#93996=CARTESIAN_POINT('Ctrl Pts',(5.74495593589617,5.62916512459886,3.25));
#93997=CARTESIAN_POINT('Ctrl Pts',(4.55911872188336,7.50555349946513,0.));
#93998=CARTESIAN_POINT('',(4.55911872188336,-3.75277674973257,6.5));
#93999=CARTESIAN_POINT('Ctrl Pts',(4.55911872188336,-3.75277674973257,6.5));
#94000=CARTESIAN_POINT('Ctrl Pts',(5.74495593589617,6.66133814775094E-15,
6.5));
#94001=CARTESIAN_POINT('Ctrl Pts',(4.55911872188336,3.75277674973257,6.5));
#94002=CARTESIAN_POINT('',(4.55911872188336,-7.50555349946513,9.19165206894919E-16));
#94003=CARTESIAN_POINT('Ctrl Pts',(4.55911872188336,-7.50555349946513,9.19165206894919E-16));
#94004=CARTESIAN_POINT('Ctrl Pts',(5.74495593589617,-5.62916512459885,3.25000000000001));
#94005=CARTESIAN_POINT('Ctrl Pts',(4.55911872188336,-3.75277674973257,6.5));
#94006=CARTESIAN_POINT('',(5.3,-6.33323321723195,-7.7559737877368E-16));
#94007=CARTESIAN_POINT('',(4.8215647221589,-7.09027674973257,-8.68308472662889E-16));
#94008=CARTESIAN_POINT('Origin',(5.3,0.,0.));
#94009=CARTESIAN_POINT('Ctrl Pts',(4.55911872188336,-3.75277674973257,-6.5));
#94010=CARTESIAN_POINT('Ctrl Pts',(5.74495593589617,-5.62916512459886,-3.24999999999999));
#94011=CARTESIAN_POINT('Ctrl Pts',(4.55911872188336,-7.50555349946513,9.19165206894919E-16));
#94012=CARTESIAN_POINT('Origin',(0.2,3.75277674973257,6.5));
#94013=CARTESIAN_POINT('',(0.2,3.75277674973257,6.5));
#94014=CARTESIAN_POINT('',(0.2,3.75277674973257,6.5));
#94015=CARTESIAN_POINT('',(0.2,-3.75277674973257,6.5));
#94016=CARTESIAN_POINT('',(0.2,3.75277674973257,6.5));
#94017=CARTESIAN_POINT('',(0.2,-3.75277674973257,6.5));
#94018=CARTESIAN_POINT('Origin',(0.2,7.50555349946513,0.));
#94019=CARTESIAN_POINT('',(0.2,7.50555349946513,0.));
#94020=CARTESIAN_POINT('',(0.2,7.50555349946513,0.));
#94021=CARTESIAN_POINT('',(0.2,7.50555349946513,0.));
#94022=CARTESIAN_POINT('Origin',(0.2,3.75277674973257,-6.5));
#94023=CARTESIAN_POINT('',(0.2,3.75277674973257,-6.5));
#94024=CARTESIAN_POINT('',(0.2,3.75277674973257,-6.5));
#94025=CARTESIAN_POINT('',(0.2,3.75277674973257,-6.5));
#94026=CARTESIAN_POINT('Origin',(0.125,0.,0.));
#94027=CARTESIAN_POINT('',(0.2,-5.8,-7.10295143505465E-16));
#94028=CARTESIAN_POINT('Origin',(0.2,0.,0.));
#94029=CARTESIAN_POINT('',(0.125,-5.8,-7.10295143505465E-16));
#94030=CARTESIAN_POINT('Origin',(-30.,3.2,0.));
#94031=CARTESIAN_POINT('',(-30.,-3.2,-3.91886975727153E-16));
#94032=CARTESIAN_POINT('Origin',(-30.,0.,0.));
#94033=CARTESIAN_POINT('Origin',(-29.6,0.,0.));
#94034=CARTESIAN_POINT('',(-29.6,-3.6,-4.40872847693047E-16));
#94035=CARTESIAN_POINT('Origin',(0.2,-3.75277674973257,-6.5));
#94036=CARTESIAN_POINT('',(0.2,-3.75277674973257,-6.5));
#94037=CARTESIAN_POINT('',(0.2,-3.75277674973257,-6.5));
#94038=CARTESIAN_POINT('',(0.2,-3.75277674973257,-6.5));
#94039=CARTESIAN_POINT('Origin',(0.2,-7.50555349946513,9.19165206894919E-16));
#94040=CARTESIAN_POINT('',(0.2,-7.50555349946513,9.19165206894919E-16));
#94041=CARTESIAN_POINT('',(0.2,-7.50555349946513,9.19165206894919E-16));
#94042=CARTESIAN_POINT('',(0.2,-7.50555349946513,9.19165206894919E-16));
#94043=CARTESIAN_POINT('Origin',(0.2,-3.75277674973257,6.5));
#94044=CARTESIAN_POINT('',(0.2,-3.75277674973257,6.5));
#94045=CARTESIAN_POINT('Origin',(5.3,0.,0.));
#94046=CARTESIAN_POINT('Origin',(0.2,0.,0.));
#94281=UNCERTAINTY_MEASURE_WITH_UNIT(LENGTH_MEASURE(0.01),#94302,
'DISTANCE_ACCURACY_VALUE',
'Maximum model space distance between geometric entities at asserted c
onnectivities');
#94285=UNCERTAINTY_MEASURE_WITH_UNIT(LENGTH_MEASURE(0.01),#94302,
'DISTANCE_ACCURACY_VALUE',
'Maximum model space distance between geometric entities at asserted c
onnectivities');
#94297=(
GEOMETRIC_REPRESENTATION_CONTEXT(3)
GLOBAL_UNCERTAINTY_ASSIGNED_CONTEXT((#94281))
GLOBAL_UNIT_ASSIGNED_CONTEXT((#94302,#94304,#94305))
REPRESENTATION_CONTEXT('','3D')
);
#94301=(
GEOMETRIC_REPRESENTATION_CONTEXT(3)
GLOBAL_UNCERTAINTY_ASSIGNED_CONTEXT((#94285))
GLOBAL_UNIT_ASSIGNED_CONTEXT((#94302,#94304,#94305))
REPRESENTATION_CONTEXT('','3D')
);
#94302=(
LENGTH_UNIT()
NAMED_UNIT(*)
SI_UNIT(.MILLI.,.METRE.)
);
#94304=(
NAMED_UNIT(*)
PLANE_ANGLE_UNIT()
SI_UNIT($,.RADIAN.)
);
#94305=(
NAMED_UNIT(*)
SI_UNIT($,.STERADIAN.)
SOLID_ANGLE_UNIT()
);
#94317=SHAPE_DEFINITION_REPRESENTATION(#94332,#94381);
#94332=PRODUCT_DEFINITION_SHAPE('',$,#94397);
#94381=SHAPE_REPRESENTATION('',(#55192),#94297);
#94385=PRODUCT_DEFINITION_CONTEXT('part definition',#94432,'design');
#94397=PRODUCT_DEFINITION('2026-10-11-08-26-45-510',
'11_ISO_4017_M8x30_Hex_Bolt',#94412,#94385);
#94412=PRODUCT_DEFINITION_FORMATION('',$,#94445);
#94432=APPLICATION_CONTEXT(
'Core Data for Automotive Mechanical Design Process');
#94433=PRODUCT_CONTEXT('part definition',#94432,'mechanical');
#94445=PRODUCT('2026-10-11-08-26-45-510','11_ISO_4017_M8x30_Hex_Bolt',$,
(#94433));
#94582=COLOUR_RGB('Black',0.12,0.14,0.17);
#94583=FILL_AREA_STYLE_COLOUR('',#94582);
#94584=FILL_AREA_STYLE('',(#94583));
#94585=SURFACE_STYLE_FILL_AREA(#94584);
#94586=SURFACE_SIDE_STYLE('',(#94585));
#94587=SURFACE_STYLE_USAGE(.BOTH.,#94586);
#94588=PRESENTATION_STYLE_ASSIGNMENT((#94587));
ENDSEC;
END-ISO-10303-21;
